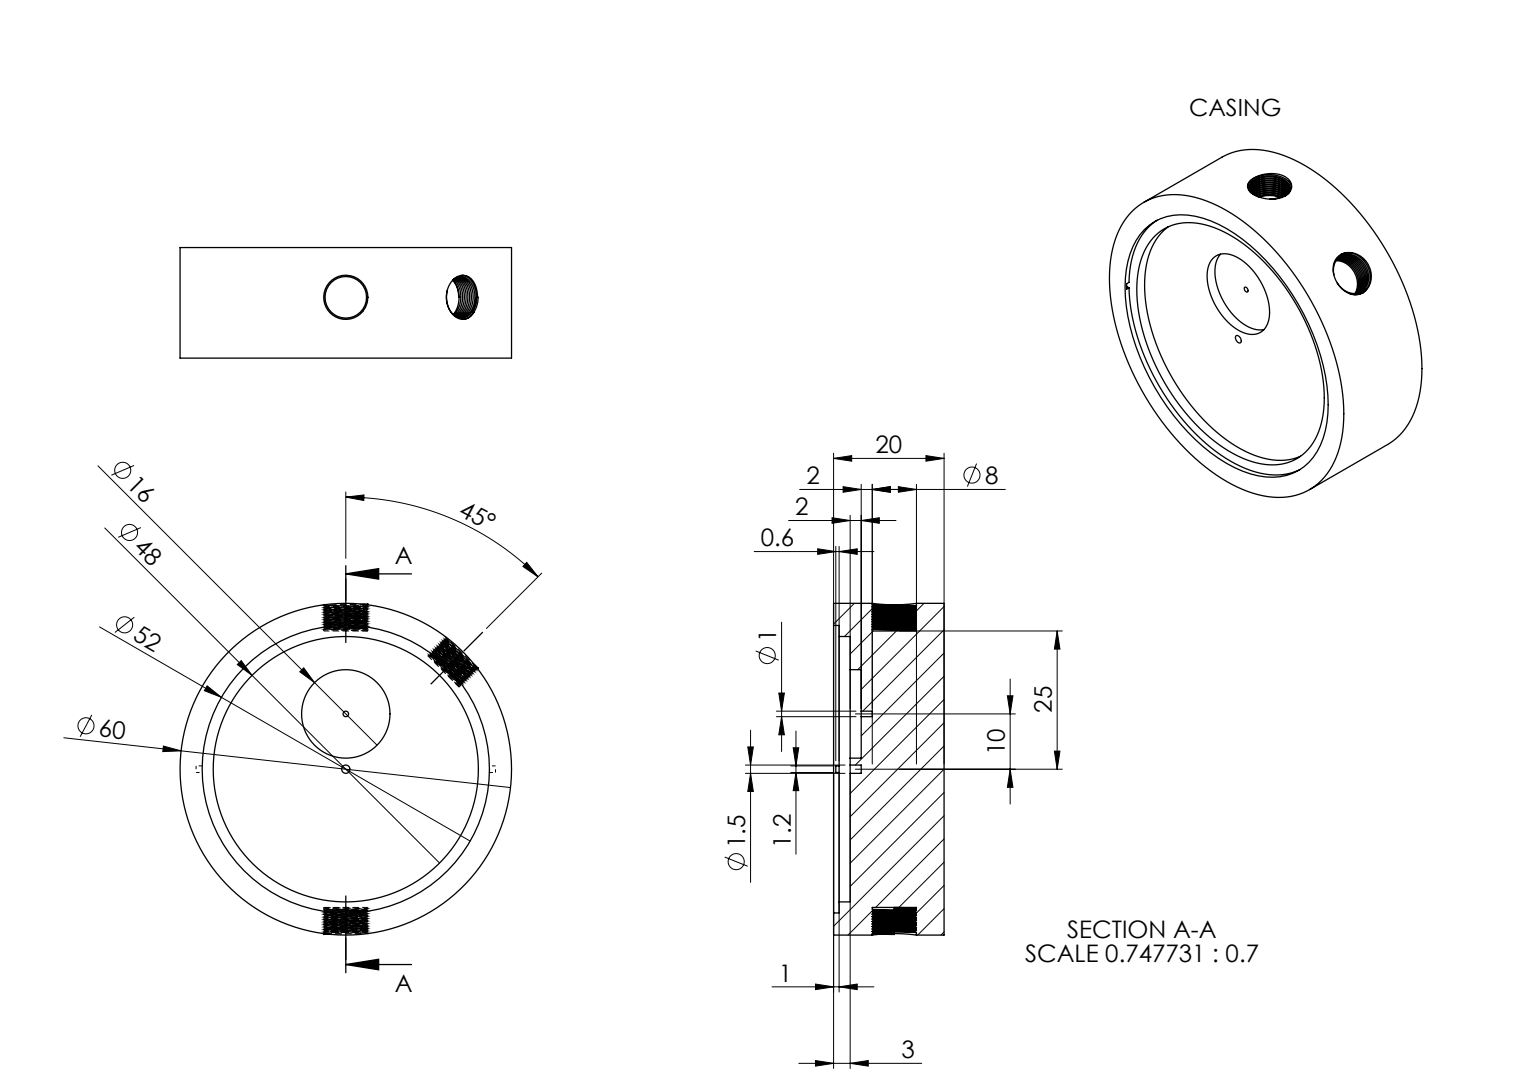
ISO-10303-21;
HEADER;
FILE_DESCRIPTION (('STEP AP214'),
    '1' );
FILE_NAME ('casing.step',
    '2026-10-26T12:50:16',
    ( '' ),
    ( '' ),
    'SwSTEP 2.0',
    'SolidWorks 2026',
    '' );
FILE_SCHEMA (( 'AUTOMOTIVE_DESIGN' ));
ENDSEC;

DATA;
#5=CARTESIAN_POINT ( 'NONE',  ( -3.756430356249995661, 28.14062499938548356, 6.831223922626973533 ) ) ;
#7=CARTESIAN_POINT ( 'NONE',  ( -3.137519842735244810E-15, 26.85624999877096641, 4.999999999999991118 ) ) ;
#13=CARTESIAN_POINT ( 'NONE',  ( 3.999999999999996003, -29.63124999877096499, 6.690598923241487306 ) ) ;
#14=CARTESIAN_POINT ( 'NONE',  ( -1.878215178124995832, 27.65312499938548640, 5.746835883940462963 ) ) ;
#15=CARTESIAN_POINT ( 'NONE',  ( 1.999999999999995781, -26.05000000000000071, 5.535898384862237620 ) ) ;
#21=CARTESIAN_POINT ( 'NONE',  ( -4.000000000000001776, -29.01249999999999929, 11.30940107675849760 ) ) ;
#22=CARTESIAN_POINT ( 'NONE',  ( 1.878215178124995832, -29.34062499938548285, 5.746835883940462963 ) ) ;
#23=ORIENTED_EDGE ( 'NONE', *, *, #8423, .T. ) ;
#24=AXIS2_PLACEMENT_3D ( 'NONE', #8722, #14489, #16466 ) ;
#28=CARTESIAN_POINT ( 'NONE',  ( -1.878215178125000939, -26.86562499938548498, 12.25316411605952283 ) ) ;
#33=CARTESIAN_POINT ( 'NONE',  ( 2.610164000359269210, 29.83019057377770622, 12.11182326528050623 ) ) ;
#34=CARTESIAN_POINT ( 'NONE',  ( 3.756430356250003211, 25.74062499938548498, 6.831223922626973533 ) ) ;
#37=CARTESIAN_POINT ( 'NONE',  ( -1.859271017917182139E-15, -26.18124999877096570, 12.99999999999999289 ) ) ;
#38=CARTESIAN_POINT ( 'NONE',  ( 20.96136040992792715, 18.30516303196848327, 12.25316411605952283 ) ) ;
#41=AXIS2_PLACEMENT_3D ( 'NONE', #20683, #20557, #10217 ) ;
#44=EDGE_CURVE ( 'NONE', #18967, #21735, #3508, .T. ) ;
#45=CARTESIAN_POINT ( 'NONE',  ( 2.620986760973688460E-15, 28.48750000000000071, 13.61880215351699874 ) ) ;
#48=DIRECTION ( 'NONE',  ( -0.7071067811865463515, 0.7071067811865487940, 0.000000000000000000 ) ) ;
#50=CARTESIAN_POINT ( 'NONE',  ( -1.071796769724487675, -29.53615380933863221, 4.999999999999988454 ) ) ;
#52=ORIENTED_EDGE ( 'NONE', *, *, #23161, .T. ) ;
#58=CARTESIAN_POINT ( 'NONE',  ( -3.756430356249996994, 25.47812499938548569, 8.999999999999992895 ) ) ;
#59=DIRECTION ( 'NONE',  ( 0.000000000000000000, 1.000000000000000000, 0.000000000000000000 ) ) ;
#64=ORIENTED_EDGE ( 'NONE', *, *, #14205, .F. ) ;
#65=ADVANCED_FACE ( 'NONE', ( #4510 ), #16441, .F. ) ;
#67=( BOUNDED_CURVE ( )  B_SPLINE_CURVE ( 2, ( #11399, #18754, #8825, #845, #17301 ),
 .UNSPECIFIED., .F., .F. ) 
 B_SPLINE_CURVE_WITH_KNOTS ( ( 3, 2, 3 ),
 ( 0.000000000000000000, 0.01666666666666666644, 0.02500000000000000486 ),
 .UNSPECIFIED. ) 
 CURVE ( )  GEOMETRIC_REPRESENTATION_ITEM ( )  RATIONAL_B_SPLINE_CURVE ( ( 1.000000000000000000, 0.8660254037844387076, 1.000000000000000000, 0.9330127018922194093, 0.9330127018922194093 ) ) 
 REPRESENTATION_ITEM ( '' )  );
#71=CARTESIAN_POINT ( 'NONE',  ( -2.000000000000003997, -26.87500000000000355, 5.535898384862238508 ) ) ;
#76=CARTESIAN_POINT ( 'NONE',  ( -3.756430356249996994, 26.26562499938548711, 8.999999999999992895 ) ) ;
#78=VECTOR ( 'NONE', #8219, 1000.000000000000000 ) ;
#80=CARTESIAN_POINT ( 'NONE',  ( -3.469446951953614189E-15, -30.00000000000000355, 4.999999999999992006 ) ) ;
#82=CARTESIAN_POINT ( 'NONE',  ( 15.67125403804690009, 21.32810828753921228, 11.30940107675849404 ) ) ;
#84=DIRECTION ( 'NONE',  ( 0.000000000000000000, 1.000000000000000000, 0.000000000000000000 ) ) ;
#85=CARTESIAN_POINT ( 'NONE',  ( 0.000000000000000000, 10.00000000000000000, 13.00000000000000178 ) ) ;
#88=CARTESIAN_POINT ( 'NONE',  ( 17.82559248041273037, 23.13798723633140142, 8.999999999999992895 ) ) ;
#91=CARTESIAN_POINT ( 'NONE',  ( -3.752267015613588906E-15, -27.36250000000000071, 4.381197846482986158 ) ) ;
#96=DIRECTION ( 'NONE',  ( 0.000000000000000000, 1.000000000000000000, 0.000000000000000000 ) ) ;
#104=AXIS2_PLACEMENT_3D ( 'NONE', #18680, #4701, #2727 ) ;
#108=FACE_OUTER_BOUND ( 'NONE', #8911, .T. ) ;
#111=FACE_OUTER_BOUND ( 'NONE', #10588, .T. ) ;
#116=CARTESIAN_POINT ( 'NONE',  ( 23.35662086519912606, 17.69976661570667176, 6.690598923241489970 ) ) ;
#119=CARTESIAN_POINT ( 'NONE',  ( 3.472074595960224386, 29.79875828571876184, 6.996763648122163559 ) ) ;
#122=CARTESIAN_POINT ( 'NONE',  ( -3.178742173564956808, 29.83148068024111410, 6.557713274934318548 ) ) ;
#125=VERTEX_POINT ( 'NONE', #4004 ) ;
#130=VERTEX_POINT ( 'NONE', #22041 ) ;
#133=ORIENTED_EDGE ( 'NONE', *, *, #9364, .F. ) ;
#143=CARTESIAN_POINT ( 'NONE',  ( -3.756430356249995661, 26.22812499938548214, 6.831223922626973533 ) ) ;
#149=DIRECTION ( 'NONE',  ( -0.7071067811865487940, -0.7071067811865463515, 0.000000000000000000 ) ) ;
#150=CARTESIAN_POINT ( 'NONE',  ( -3.369928719974892281E-15, -25.50624999877096855, 4.999999999999992006 ) ) ;
#152=CARTESIAN_POINT ( 'NONE',  ( -4.000000000000003553, -28.99374999877096926, 8.999999999999992895 ) ) ;
#153=CARTESIAN_POINT ( 'NONE',  ( -3.756430356249996994, 28.62812499938548427, 8.999999999999992895 ) ) ;
#156=CARTESIAN_POINT ( 'NONE',  ( -3.834746474454188013E-15, -25.95624999877096428, 4.999999999999992006 ) ) ;
#159=CARTESIAN_POINT ( 'NONE',  ( -2.672651547586948120E-15, -29.52812499938548285, 13.33755215474603162 ) ) ;
#160=ORIENTED_EDGE ( 'NONE', *, *, #14930, .T. ) ;
#167=CARTESIAN_POINT ( 'NONE',  ( 1.859271017917182139E-15, 29.78124999877096712, 12.99999999999999289 ) ) ;
#168=CARTESIAN_POINT ( 'NONE',  ( 3.756430356250003211, 26.19062499938548783, 6.831223922626973533 ) ) ;
#172=FACE_OUTER_BOUND ( 'NONE', #2936, .T. ) ;
#173=CARTESIAN_POINT ( 'NONE',  ( 18.33395301051795911, 18.33395301051789161, 13.33755215474602984 ) ) ;
#174=CARTESIAN_POINT ( 'NONE',  ( 17.58044234725058175, 23.23729659674288683, 11.30940107675849404 ) ) ;
#177=CARTESIAN_POINT ( 'NONE',  ( 4.000000000000003553, 28.18750000000000000, 6.690598923241489970 ) ) ;
#178=CARTESIAN_POINT ( 'NONE',  ( 3.756430356250003211, 28.77812499938548285, 6.831223922626973533 ) ) ;
#180=DIRECTION ( 'NONE',  ( 1.000000000000000000, 0.000000000000000000, 0.000000000000000000 ) ) ;
#188=CARTESIAN_POINT ( 'NONE',  ( 4.000000000000003553, 29.44374999877096855, 8.999999999999992895 ) ) ;
#201=CARTESIAN_POINT ( 'NONE',  ( 15.35955758102464408, 20.67195233694332401, 8.999999999999992895 ) ) ;
#202=EDGE_CURVE ( 'NONE', #18727, #446, #20080, .T. ) ;
#203=CARTESIAN_POINT ( 'NONE',  ( -1.878215178124998497, 25.44062499938548427, 12.25316411605951927 ) ) ;
#205=CARTESIAN_POINT ( 'NONE',  ( 3.999999999999996447, -28.76874999877096784, 8.999999999999992895 ) ) ;
#206=CARTESIAN_POINT ( 'NONE',  ( 20.78010053211970032, 20.78010053211962926, 13.61880215351699874 ) ) ;
#210=CARTESIAN_POINT ( 'NONE',  ( 21.65072575558658130, 18.82229863084031507, 5.535898384862238508 ) ) ;
#212=FACE_BOUND ( 'NONE', #16233, .T. ) ;
#213=ORIENTED_EDGE ( 'NONE', *, *, #20465, .F. ) ;
#215=CARTESIAN_POINT ( 'NONE',  ( -4.000000000000003553, -28.18750000000000000, 6.690598923241489970 ) ) ;
#217=ORIENTED_EDGE ( 'NONE', *, *, #6066, .T. ) ;
#219=CARTESIAN_POINT ( 'NONE',  ( 23.82728881686095335, 18.17043456736849549, 8.999999999999992895 ) ) ;
#223=( NAMED_UNIT ( * ) PLANE_ANGLE_UNIT ( ) SI_UNIT ( $, .RADIAN. ) );
#225=( BOUNDED_SURFACE ( )  B_SPLINE_SURFACE ( 1, 2, ( 
 ( #23282, #15066, #19226, #12835, #25256, #13355, #9305, #1328, #23041, #11121, #11003, #7335, #805, #4859, #6951, #3034, #14929, #17290, #15314, #5365, #6826, #4989, #3408, #23165, #3271, #1184, #20809, #11245, #18713, #14809, #25127, #22903, #22782, #7213, #5128, #3154, #5245, #18859, #15195, #2891, #949, #8926, #12968, #18983, #9042, #17024, #13105, #21078, #19100, #11896, #19864, #23669, #17408, #3538, #9928, #7455, #23415, #17792, #7595, #5502, #13493, #15443, #3926, #23933, #5746, #11511, #11387, #7721, #9545, #15581, #17532, #25759, #1963, #17913, #11771, #13997, #19750, #5, #5885, #21462, #15967, #25506, #15705, #23549, #1848, #23795, #25372, #17671, #13730, #5631, #19480, #7979, #6016, #21968, #13611, #19361, #1456, #1574, #21577, #3656, #11632, #19609, #21708, #3793, #1713, #9427, #9810, #9687, #25639, #7840, #15824, #13869, #21843, #20128, #2470, #14641, #12011, #18436, #18572, #4433, #18301 ),
 ( #24054, #14507, #12542, #2614, #10441, #2229, #2094, #531, #16352, #14392, #16485, #4175, #8503, #22479, #10573, #24447, #10187, #4559, #4044, #6524, #20373, #20519, #19988, #654, #8623, #24321, #10061, #22086, #16600, #143, #16090, #24562, #267, #6138, #14122, #8116, #6652, #18060, #6401, #12154, #18184, #393, #8235, #16212, #24181, #6269, #14261, #22228, #12407, #4313, #12287, #20253, #2351, #10306, #8362, #22349, #1037, #20778, #13070, #9481, #10697, #2998, #18952, #8890, #4827, #13549, #5568, #15512, #911, #19534, #11566, #772, #10827, #8745, #16735, #4951, #7655, #10966, #14776, #22871, #18820, #12933, #17460, #9011, #22621, #22752, #12804, #21513, #16992, #2857, #24957, #14897, #16874, #24838, #7039, #24705, #25571, #25432, #6915, #12683, #18684, #9614, #1636, #15027, #23481, #21048, #20911, #20652, #3123, #23005, #5092, #7517, #11091, #19070, #3595, #17594, #1512, #4708, #2735, #6791, #18129 ) ),
 .UNSPECIFIED., .F., .F., .F. ) 
 B_SPLINE_SURFACE_WITH_KNOTS ( ( 2, 2 ),
 ( 3, 2, 2, 2, 2, 2, 2, 2, 2, 2, 2, 2, 2, 2, 2, 2, 2, 2, 2, 2, 2, 2, 2, 2, 2, 2, 2, 2, 2, 2, 2, 2, 2, 2, 2, 2, 2, 2, 2, 2, 2, 2, 2, 2, 2, 2, 2, 2, 2, 2, 2, 2, 2, 2, 2, 2, 2, 2, 2, 2, 3 ),
 ( 0.000000000000000000, 1.000000000000000000 ),
 ( 0.000000000000000000, 0.01666666666666666644, 0.03333333333333333287, 0.05000000000000000278, 0.06666666666666666574, 0.08333333333333332871, 0.1000000000000000056, 0.1166666666666666685, 0.1333333333333333315, 0.1499999999999999944, 0.1666666666666666574, 0.1833333333333333204, 0.2000000000000000111, 0.2166666666666666741, 0.2333333333333333370, 0.2500000000000000000, 0.2666666666666666630, 0.2833333333333333259, 0.2999999999999999889, 0.3166666666666666519, 0.3333333333333333148, 0.3499999999999999778, 0.3666666666666666408, 0.3833333333333333592, 0.4000000000000000222, 0.4166666666666666852, 0.4333333333333333481, 0.4500000000000000111, 0.4666666666666666741, 0.4833333333333333370, 0.5000000000000000000, 0.5166666666666667185, 0.5333333333333333259, 0.5500000000000000444, 0.5666666666666666519, 0.5833333333333333703, 0.5999999999999999778, 0.6166666666666666963, 0.6333333333333333037, 0.6500000000000000222, 0.6666666666666666297, 0.6833333333333333481, 0.6999999999999999556, 0.7166666666666666741, 0.7333333333333332815, 0.7500000000000000000, 0.7666666666666667185, 0.7833333333333333259, 0.8000000000000000444, 0.8166666666666666519, 0.8333333333333333703, 0.8499999999999999778, 0.8666666666666666963, 0.8833333333333333037, 0.9000000000000000222, 0.9166666666666666297, 0.9333333333333333481, 0.9499999999999999556, 0.9666666666666666741, 0.9833333333333332815, 1.000000000000000000 ),
 .UNSPECIFIED. ) 
 GEOMETRIC_REPRESENTATION_ITEM ( )  RATIONAL_B_SPLINE_SURFACE ( (
 ( 1.000000000000000000, 0.8660254037844387076, 1.000000000000000000, 0.8660254037844387076, 1.000000000000000000, 0.8660254037844387076, 1.000000000000000000, 0.8660254037844387076, 1.000000000000000000, 0.8660254037844387076, 1.000000000000000000, 0.8660254037844387076, 1.000000000000000000, 0.8660254037844387076, 1.000000000000000000, 0.8660254037844387076, 1.000000000000000000, 0.8660254037844387076, 1.000000000000000000, 0.8660254037844387076, 1.000000000000000000, 0.8660254037844387076, 1.000000000000000000, 0.8660254037844387076, 1.000000000000000000, 0.8660254037844387076, 1.000000000000000000, 0.8660254037844387076, 1.000000000000000000, 0.8660254037844387076, 1.000000000000000000, 0.8660254037844387076, 1.000000000000000000, 0.8660254037844387076, 1.000000000000000000, 0.8660254037844387076, 1.000000000000000000, 0.8660254037844387076, 1.000000000000000000, 0.8660254037844387076, 1.000000000000000000, 0.8660254037844387076, 1.000000000000000000, 0.8660254037844387076, 1.000000000000000000, 0.8660254037844387076, 1.000000000000000000, 0.8660254037844387076, 1.000000000000000000, 0.8660254037844387076, 1.000000000000000000, 0.8660254037844387076, 1.000000000000000000, 0.8660254037844387076, 1.000000000000000000, 0.8660254037844387076, 1.000000000000000000, 0.8660254037844387076, 1.000000000000000000, 0.8660254037844387076, 1.000000000000000000, 0.8660254037844387076, 1.000000000000000000, 0.8660254037844387076, 1.000000000000000000, 0.8660254037844387076, 1.000000000000000000, 0.8660254037844387076, 1.000000000000000000, 0.8660254037844387076, 1.000000000000000000, 0.8660254037844387076, 1.000000000000000000, 0.8660254037844387076, 1.000000000000000000, 0.8660254037844387076, 1.000000000000000000, 0.8660254037844387076, 1.000000000000000000, 0.8660254037844387076, 1.000000000000000000, 0.8660254037844387076, 1.000000000000000000, 0.8660254037844387076, 1.000000000000000000, 0.8660254037844387076, 1.000000000000000000, 0.8660254037844387076, 1.000000000000000000, 0.8660254037844387076, 1.000000000000000000, 0.8660254037844387076, 1.000000000000000000, 0.8660254037844387076, 1.000000000000000000, 0.8660254037844387076, 1.000000000000000000, 0.8660254037844387076, 1.000000000000000000, 0.8660254037844387076, 1.000000000000000000, 0.8660254037844387076, 1.000000000000000000, 0.8660254037844387076, 1.000000000000000000, 0.8660254037844387076, 1.000000000000000000, 0.8660254037844387076, 1.000000000000000000, 0.8660254037844387076, 1.000000000000000000, 0.8660254037844387076, 1.000000000000000000, 0.8660254037844387076, 1.000000000000000000, 0.8660254037844387076, 1.000000000000000000, 0.8660254037844387076, 1.000000000000000000, 0.8660254037844387076, 1.000000000000000000),
 ( 1.000000000000000000, 0.8660254037844387076, 1.000000000000000000, 0.8660254037844387076, 1.000000000000000000, 0.8660254037844387076, 1.000000000000000000, 0.8660254037844387076, 1.000000000000000000, 0.8660254037844387076, 1.000000000000000000, 0.8660254037844387076, 1.000000000000000000, 0.8660254037844387076, 1.000000000000000000, 0.8660254037844387076, 1.000000000000000000, 0.8660254037844387076, 1.000000000000000000, 0.8660254037844387076, 1.000000000000000000, 0.8660254037844387076, 1.000000000000000000, 0.8660254037844387076, 1.000000000000000000, 0.8660254037844387076, 1.000000000000000000, 0.8660254037844387076, 1.000000000000000000, 0.8660254037844387076, 1.000000000000000000, 0.8660254037844387076, 1.000000000000000000, 0.8660254037844387076, 1.000000000000000000, 0.8660254037844387076, 1.000000000000000000, 0.8660254037844387076, 1.000000000000000000, 0.8660254037844387076, 1.000000000000000000, 0.8660254037844387076, 1.000000000000000000, 0.8660254037844387076, 1.000000000000000000, 0.8660254037844387076, 1.000000000000000000, 0.8660254037844387076, 1.000000000000000000, 0.8660254037844387076, 1.000000000000000000, 0.8660254037844387076, 1.000000000000000000, 0.8660254037844387076, 1.000000000000000000, 0.8660254037844387076, 1.000000000000000000, 0.8660254037844387076, 1.000000000000000000, 0.8660254037844387076, 1.000000000000000000, 0.8660254037844387076, 1.000000000000000000, 0.8660254037844387076, 1.000000000000000000, 0.8660254037844387076, 1.000000000000000000, 0.8660254037844387076, 1.000000000000000000, 0.8660254037844387076, 1.000000000000000000, 0.8660254037844387076, 1.000000000000000000, 0.8660254037844387076, 1.000000000000000000, 0.8660254037844387076, 1.000000000000000000, 0.8660254037844387076, 1.000000000000000000, 0.8660254037844387076, 1.000000000000000000, 0.8660254037844387076, 1.000000000000000000, 0.8660254037844387076, 1.000000000000000000, 0.8660254037844387076, 1.000000000000000000, 0.8660254037844387076, 1.000000000000000000, 0.8660254037844387076, 1.000000000000000000, 0.8660254037844387076, 1.000000000000000000, 0.8660254037844387076, 1.000000000000000000, 0.8660254037844387076, 1.000000000000000000, 0.8660254037844387076, 1.000000000000000000, 0.8660254037844387076, 1.000000000000000000, 0.8660254037844387076, 1.000000000000000000, 0.8660254037844387076, 1.000000000000000000, 0.8660254037844387076, 1.000000000000000000, 0.8660254037844387076, 1.000000000000000000, 0.8660254037844387076, 1.000000000000000000, 0.8660254037844387076, 1.000000000000000000, 0.8660254037844387076, 1.000000000000000000, 0.8660254037844387076, 1.000000000000000000, 0.8660254037844387076, 1.000000000000000000, 0.8660254037844387076, 1.000000000000000000) ) ) 
 REPRESENTATION_ITEM ( '' )  SURFACE ( )  );
#230=CIRCLE ( 'NONE', #3567, 26.00000000000000355 ) ;
#234=CARTESIAN_POINT ( 'NONE',  ( 22.12360341637413441, 16.46674916688168366, 6.690598923241489970 ) ) ;
#235=CARTESIAN_POINT ( 'NONE',  ( 21.07620149587250680, 15.41934724638005605, 11.30940107675849760 ) ) ;
#237=CARTESIAN_POINT ( 'NONE',  ( 16.26111872703749128, 21.57351348295617299, 11.16877607737301226 ) ) ;
#238=CARTESIAN_POINT ( 'NONE',  ( 20.69613160098474580, 17.86770447623847957, 5.535898384862238508 ) ) ;
#245=CARTESIAN_POINT ( 'NONE',  ( -1.290629128713961293, 29.97320584640673147, 5.204870533884474071 ) ) ;
#249=AXIS2_PLACEMENT_3D ( 'NONE', #7329, #17401, #17148 ) ;
#253=CARTESIAN_POINT ( 'NONE',  ( 1.878215178124998497, -26.79062499938548214, 12.25316411605951927 ) ) ;
#256=VERTEX_POINT ( 'NONE', #11047 ) ;
#267=CARTESIAN_POINT ( 'NONE',  ( -1.878215178124998497, 26.34062499938548285, 12.25316411605951927 ) ) ;
#274=CARTESIAN_POINT ( 'NONE',  ( 15.32653948221845575, 20.98339373171076971, 8.999999999999992895 ) ) ;
#275=CARTESIAN_POINT ( 'NONE',  ( 3.999999999999996003, -29.18124999877096926, 6.690598923241487306 ) ) ;
#278=DIRECTION ( 'NONE',  ( 0.000000000000000000, 1.000000000000000000, 0.000000000000000000 ) ) ;
#280=CARTESIAN_POINT ( 'NONE',  ( 3.178742173564956808, -29.83148068024111410, 6.557713274934318548 ) ) ;
#282=CARTESIAN_POINT ( 'NONE',  ( 1.057460391440397258E-14, -29.16249999999999787, 4.999999999999992006 ) ) ;
#283=FACE_OUTER_BOUND ( 'NONE', #1653, .T. ) ;
#285=EDGE_LOOP ( 'NONE', ( #3996, #19961, #21885, #25596, #64, #22498, #18380, #2629, #2882, #13648, #16581, #11690, #2311, #3515, #5348, #18845, #16021, #25747, #20827, #6154, #13089, #936, #2532, #21309 ) ) ;
#290=EDGE_LOOP ( 'NONE', ( #13571, #12401, #24240, #13980, #21957, #2916, #23588, #1468, #14108, #13538, #2496, #5234, #22275, #20569, #6506, #25331, #10531, #8615, #1170, #12139, #14587, #14625, #15332, #12330, #21832 ) ) ;
#292=CARTESIAN_POINT ( 'NONE',  ( 3.756430356250002323, 27.01562499938548356, 11.16877607737301403 ) ) ;
#295=CARTESIAN_POINT ( 'NONE',  ( 20.11283227250407180, 17.45663489454462436, 5.746835883940462963 ) ) ;
#301=CARTESIAN_POINT ( 'NONE',  ( 3.756430356250003655, 29.64062499938548356, 8.999999999999992895 ) ) ;
#304=CARTESIAN_POINT ( 'NONE',  ( 21.21320343559646915, 21.21320343559638744, 8.999999999999992895 ) ) ;
#312=CARTESIAN_POINT ( 'NONE',  ( 21.42091605170094937, 15.76406180220850040, 8.999999999999992895 ) ) ;
#315=DIRECTION ( 'NONE',  ( 0.000000000000000000, 1.000000000000000000, 0.000000000000000000 ) ) ;
#319=CARTESIAN_POINT ( 'NONE',  ( 4.000000000000003553, 29.08750000000000213, 6.690598923241489970 ) ) ;
#323=CARTESIAN_POINT ( 'NONE',  ( -3.756430356249995661, 26.67812499938548498, 6.831223922626973533 ) ) ;
#325=CARTESIAN_POINT ( 'NONE',  ( 18.91510639674018890, 21.74353352148630236, 5.535898384862237620 ) ) ;
#328=CARTESIAN_POINT ( 'NONE',  ( 4.000000000000003553, 25.03750000000000142, 6.690598923241489970 ) ) ;
#329=CARTESIAN_POINT ( 'NONE',  ( 1.878215178124998497, -25.89062499938548356, 12.25316411605951927 ) ) ;
#331=AXIS2_PLACEMENT_3D ( 'NONE', #1726, #17803, #5513 ) ;
#338=ORIENTED_EDGE ( 'NONE', *, *, #8418, .T. ) ;
#339=CARTESIAN_POINT ( 'NONE',  ( 1.071796769724493448, -29.12634618820329990, 4.999999999999995559 ) ) ;
#347=CARTESIAN_POINT ( 'NONE',  ( 3.756430356249996994, -26.82812499938548711, 8.999999999999992895 ) ) ;
#356=CARTESIAN_POINT ( 'NONE',  ( 19.96824085905927149, 21.48399038691124474, 12.99999999999999289 ) ) ;
#358=CIRCLE ( 'NONE', #25835, 0.5000000000000001110 ) ;
#360=CARTESIAN_POINT ( 'NONE',  ( -3.469446951953614189E-15, -30.00000000000000355, 8.999999999999992895 ) ) ;
#361=CARTESIAN_POINT ( 'NONE',  ( 21.67957950013421353, 16.36718474421539682, 11.16877607737301226 ) ) ;
#363=CARTESIAN_POINT ( 'NONE',  ( 16.55955693104344206, 22.21641118053575426, 8.999999999999992895 ) ) ;
#365=CARTESIAN_POINT ( 'NONE',  ( 3.999999999999996447, -27.02500000000000213, 8.999999999999992895 ) ) ;
#368=CARTESIAN_POINT ( 'NONE',  ( -2.007411586324088226, 29.93355017142139118, 12.46960170373642640 ) ) ;
#370=CARTESIAN_POINT ( 'NONE',  ( 17.85665593321704137, 17.85665593321697386, 4.662447845253954171 ) ) ;
#371=CARTESIAN_POINT ( 'NONE',  ( -1.626862140677534194E-14, -28.03750000000000497, 12.99999999999999289 ) ) ;
#374=CARTESIAN_POINT ( 'NONE',  ( 2.620986760973688460E-15, 26.63124999877097565, 13.61880215351699874 ) ) ;
#375=CARTESIAN_POINT ( 'NONE',  ( 3.756430356249996994, -26.71562499938548285, 8.999999999999992895 ) ) ;
#377=ORIENTED_EDGE ( 'NONE', *, *, #20034, .T. ) ;
#393=CARTESIAN_POINT ( 'NONE',  ( -3.756430356249995661, 26.67812499938548498, 6.831223922626973533 ) ) ;
#400=CARTESIAN_POINT ( 'NONE',  ( -1.999999999999995781, 28.69374999877096855, 5.535898384862237620 ) ) ;
#401=CARTESIAN_POINT ( 'NONE',  ( -3.756430356250003655, -25.70312499938548356, 8.999999999999992895 ) ) ;
#410=CARTESIAN_POINT ( 'NONE',  ( 21.21320343559646915, 21.21320343559638744, 8.999999999999992895 ) ) ;
#421=VERTEX_POINT ( 'NONE', #17718 ) ;
#424=CARTESIAN_POINT ( 'NONE',  ( -1.878215178124995832, 25.85312499938548569, 5.746835883940462963 ) ) ;
#426=ADVANCED_FACE ( 'NONE', ( #15751 ), #3586, .T. ) ;
#430=CARTESIAN_POINT ( 'NONE',  ( 20.64316235839397962, 17.98696498043453573, 12.25316411605952283 ) ) ;
#437=CARTESIAN_POINT ( 'NONE',  ( -1.878215178124995832, 28.89062499938548356, 5.746835883940462963 ) ) ;
#440=CARTESIAN_POINT ( 'NONE',  ( 18.19474136253732865, 18.19474136253726826, 12.99999999999999289 ) ) ;
#446=VERTEX_POINT ( 'NONE', #13409 ) ;
#449=CARTESIAN_POINT ( 'NONE',  ( -3.999999999999996447, 26.12500000000000355, 8.999999999999992895 ) ) ;
#461=AXIS2_PLACEMENT_3D ( 'NONE', #21744, #5539, #19508 ) ;
#465=CARTESIAN_POINT ( 'NONE',  ( 3.735045420075836212E-15, 27.05312499938548498, 4.662447845253954171 ) ) ;
#467=CARTESIAN_POINT ( 'NONE',  ( 17.93620544610053003, 17.93620544610046252, 4.662447845253954171 ) ) ;
#468=CARTESIAN_POINT ( 'NONE',  ( 23.66156066545488201, 18.00470641596242771, 11.30940107675849760 ) ) ;
#471=CARTESIAN_POINT ( 'NONE',  ( 0.000000000000000000, 0.000000000000000000, 20.00001200000000168 ) ) ;
#476=VERTEX_POINT ( 'NONE', #17452 ) ;
#478=CARTESIAN_POINT ( 'NONE',  ( -4.000000000000003553, -28.15000000000000213, 8.999999999999992895 ) ) ;
#487=CARTESIAN_POINT ( 'NONE',  ( -1.878215178125004048, -27.57812499938548711, 5.746835883940462963 ) ) ;
#494=CARTESIAN_POINT ( 'NONE',  ( 21.86285778994254514, 19.03443066519628601, 12.46410161513774817 ) ) ;
#499=CARTESIAN_POINT ( 'NONE',  ( 18.02680350200553150, 20.85523062675164851, 12.46410161513774639 ) ) ;
#501=CARTESIAN_POINT ( 'NONE',  ( 15.94292067550354730, 21.25531543142222901, 11.16877607737301226 ) ) ;
#502=CARTESIAN_POINT ( 'NONE',  ( 22.18105584147648912, 19.35262871673023000, 12.46410161513774817 ) ) ;
#503=CARTESIAN_POINT ( 'NONE',  ( 3.834746474454188013E-15, 28.26249999999999929, 4.999999999999992006 ) ) ;
#504=CARTESIAN_POINT ( 'NONE',  ( 21.55218544786934132, 20.03643592001721530, 12.99999999999999467 ) ) ;
#506=CARTESIAN_POINT ( 'NONE',  ( 27.09999999999999787, 0.6000000000000000888, 19.59999999999999787 ) ) ;
#509=CARTESIAN_POINT ( 'NONE',  ( 18.33395301051795911, 18.33395301051789517, 13.33755215474603162 ) ) ;
#511=CARTESIAN_POINT ( 'NONE',  ( 3.756430356250003655, 29.69687499938548569, 8.999999999999992895 ) ) ;
#513=CARTESIAN_POINT ( 'NONE',  ( 3.756430356249996994, -27.16562499938548214, 8.999999999999992895 ) ) ;
#514=CARTESIAN_POINT ( 'NONE',  ( -3.999999999999995559, 25.18750000000000000, 6.690598923241487306 ) ) ;
#517=LINE ( 'NONE', #10811, #790 ) ;
#520=CARTESIAN_POINT ( 'NONE',  ( 3.756430356249995661, -29.49062499938548498, 6.831223922626973533 ) ) ;
#522=AXIS2_PLACEMENT_3D ( 'NONE', #18913, #11050, #20738 ) ;
#531=CARTESIAN_POINT ( 'NONE',  ( -3.756430356249997882, 25.40312499938548285, 11.16877607737301226 ) ) ;
#540=CARTESIAN_POINT ( 'NONE',  ( 1.999999999999998224, -29.29374999877096997, 12.46410161513774639 ) ) ;
#542=CARTESIAN_POINT ( 'NONE',  ( 21.21320343559646915, 21.21320343559638744, 12.99999999999999289 ) ) ;
#544=CARTESIAN_POINT ( 'NONE',  ( 1.290629128713961293, -29.97320584640673147, 5.204870533884474071 ) ) ;
#548=LINE ( 'NONE', #4449, #1635 ) ;
#551=ORIENTED_EDGE ( 'NONE', *, *, #25079, .T. ) ;
#555=CARTESIAN_POINT ( 'NONE',  ( -4.000000000000003553, -27.73750000000000071, 6.690598923241489970 ) ) ;
#557=EDGE_LOOP ( 'NONE', ( #23842, #6060, #17814, #23687, #3257, #25679 ) ) ;
#559=CARTESIAN_POINT ( 'NONE',  ( 3.756430356250002323, 26.56562499938548783, 11.16877607737301403 ) ) ;
#563=CARTESIAN_POINT ( 'NONE',  ( 21.73261250872320716, 16.42021775280438689, 6.831223922626973533 ) ) ;
#570=CARTESIAN_POINT ( 'NONE',  ( -1.071796769724487230, 27.77634618820330559, 4.999999999999992006 ) ) ;
#572=CARTESIAN_POINT ( 'NONE',  ( -1.878215178124998497, 29.04062499938548569, 12.25316411605951927 ) ) ;
#584=CARTESIAN_POINT ( 'NONE',  ( 1.057460391440397258E-14, -28.71250000000000213, 4.999999999999992006 ) ) ;
#589=ORIENTED_EDGE ( 'NONE', *, *, #21385, .T. ) ;
#590=FACE_OUTER_BOUND ( 'NONE', #13824, .T. ) ;
#592=CARTESIAN_POINT ( 'NONE',  ( 1.071796769724487675, 29.14240381056766438, 4.999999999999988454 ) ) ;
#594=CARTESIAN_POINT ( 'NONE',  ( 20.53936981547090568, 15.22697505955208896, 6.831223922626973533 ) ) ;
#596=CARTESIAN_POINT ( 'NONE',  ( -1.878215178124995832, 28.44062499938548427, 5.746835883940462963 ) ) ;
#598=ADVANCED_FACE ( 'NONE', ( #6456 ), #4362, .F. ) ;
#599=APPLICATION_CONTEXT ( 'automotive_design' ) ;
#602=CARTESIAN_POINT ( 'NONE',  ( 1.859271017917182139E-15, 29.33124999877096428, 12.99999999999999289 ) ) ;
#603=CARTESIAN_POINT ( 'NONE',  ( -2.672651547586948120E-15, -27.72812499938548569, 13.33755215474603162 ) ) ;
#608=CARTESIAN_POINT ( 'NONE',  ( -3.752267015613588906E-15, -29.16250000000000142, 4.381197846482986158 ) ) ;
#611=ORIENTED_EDGE ( 'NONE', *, *, #24958, .T. ) ;
#617=CARTESIAN_POINT ( 'NONE',  ( -2.672651547586948120E-15, -26.04062499938548925, 13.33755215474603162 ) ) ;
#619=CARTESIAN_POINT ( 'NONE',  ( 20.05209915500855544, 18.53634962715644363, 4.999999999999989342 ) ) ;
#622=CARTESIAN_POINT ( 'NONE',  ( 3.469446951953614189E-15, 30.00000000000000355, 4.999999999999992006 ) ) ;
#623=CARTESIAN_POINT ( 'NONE',  ( 18.60454468811453310, 20.12029421596650991, 4.999999999999992006 ) ) ;
#626=CARTESIAN_POINT ( 'NONE',  ( 16.89751483010538990, 22.20990958602406451, 11.16877607737301226 ) ) ;
#627=CARTESIAN_POINT ( 'NONE',  ( 18.87533163942939041, 21.70375876417550032, 5.535898384862237620 ) ) ;
#628=CARTESIAN_POINT ( 'NONE',  ( 23.96650046397252609, 18.30964621448006824, 8.999999999999992895 ) ) ;
#629=CARTESIAN_POINT ( 'NONE',  ( 23.66156066545488201, 18.00470641596242771, 11.30940107675849760 ) ) ;
#637=CARTESIAN_POINT ( 'NONE',  ( 2.000000000000000888, 27.56874999877096855, 12.46410161513774817 ) ) ;
#638=CARTESIAN_POINT ( 'NONE',  ( 3.756430356249995661, -25.77812499938548640, 6.831223922626973533 ) ) ;
#640=ORIENTED_EDGE ( 'NONE', *, *, #22909, .T. ) ;
#644=CARTESIAN_POINT ( 'NONE',  ( 3.756430356249995661, -25.32812499938548356, 6.831223922626973533 ) ) ;
#645=ORIENTED_EDGE ( 'NONE', *, *, #15056, .T. ) ;
#646=ORIENTED_EDGE ( 'NONE', *, *, #19907, .T. ) ;
#653=CARTESIAN_POINT ( 'NONE',  ( -3.369928719974892281E-15, -25.50624999877096855, 4.999999999999992006 ) ) ;
#654=CARTESIAN_POINT ( 'NONE',  ( 3.756430356250002323, 26.00312499938548427, 11.16877607737301226 ) ) ;
#658=DIRECTION ( 'NONE',  ( 0.000000000000000000, 0.000000000000000000, -1.000000000000000000 ) ) ;
#660=CARTESIAN_POINT ( 'NONE',  ( -3.999999999999997335, 28.80624999877096926, 11.30940107675849404 ) ) ;
#661=CARTESIAN_POINT ( 'NONE',  ( -3.735045420075836212E-15, -27.16562499938548569, 4.662447845253954171 ) ) ;
#663=CARTESIAN_POINT ( 'NONE',  ( 3.999999999999996447, -26.12500000000000355, 8.999999999999992895 ) ) ;
#664=CARTESIAN_POINT ( 'NONE',  ( 1.999999999999995781, -25.15000000000000213, 5.535898384862237620 ) ) ;
#665=CARTESIAN_POINT ( 'NONE',  ( 3.974007292349814424, -29.73566758725665338, 9.525109153848150711 ) ) ;
#670=EDGE_CURVE ( 'NONE', #18554, #13915, #7548, .T. ) ;
#673=ORIENTED_EDGE ( 'NONE', *, *, #14998, .F. ) ;
#676=ADVANCED_FACE ( 'NONE', ( #6327 ), #18231, .F. ) ;
#681=CARTESIAN_POINT ( 'NONE',  ( 1.878215178125000939, 28.77812499938548640, 12.25316411605952283 ) ) ;
#684=CARTESIAN_POINT ( 'NONE',  ( 17.53391093317328142, 22.84630568909195958, 11.16877607737301226 ) ) ;
#695=CARTESIAN_POINT ( 'NONE',  ( -1.626862140677534194E-14, -28.03750000000000497, 12.99999999999999289 ) ) ;
#696=AXIS2_PLACEMENT_3D ( 'NONE', #9375, #6205, #16157 ) ;
#697=ORIENTED_EDGE ( 'NONE', *, *, #18302, .T. ) ;
#709=CARTESIAN_POINT ( 'NONE',  ( 16.28113363682029657, 21.93798788631260877, 8.999999999999992895 ) ) ;
#710=CARTESIAN_POINT ( 'NONE',  ( 4.000000000000001776, 26.76250000000000284, 11.30940107675849760 ) ) ;
#712=CARTESIAN_POINT ( 'NONE',  ( 19.23778763078571430, 16.58159025282627397, 5.746835883940462963 ) ) ;
#713=ADVANCED_FACE ( 'NONE', ( #25117 ), #1318, .F. ) ;
#715=CARTESIAN_POINT ( 'NONE',  ( 3.735045420075836212E-15, 28.40312499938548640, 4.662447845253954171 ) ) ;
#716=CARTESIAN_POINT ( 'NONE',  ( 19.55598568231966539, 16.89978830436022150, 5.746835883940462963 ) ) ;
#717=CARTESIAN_POINT ( 'NONE',  ( 20.14370442905180880, 20.14370442905173775, 13.61880215351699874 ) ) ;
#720=CARTESIAN_POINT ( 'NONE',  ( -3.735045420075836212E-15, -27.05312499938548498, 4.662447845253954171 ) ) ;
#724=CARTESIAN_POINT ( 'NONE',  ( 1.999999999999995781, -28.75000000000000000, 5.535898384862237620 ) ) ;
#731=CARTESIAN_POINT ( 'NONE',  ( 1.878215178124995832, -26.75312499938548783, 5.746835883940462963 ) ) ;
#739=( BOUNDED_CURVE ( )  B_SPLINE_CURVE ( 2, ( #20311, #10242, #24247, #15891, #16419, #18125, #8045, #19919, #14185 ),
 .UNSPECIFIED., .F., .F. ) 
 B_SPLINE_CURVE_WITH_KNOTS ( ( 3, 2, 2, 2, 3 ),
 ( 0.8750000000000000000, 0.8833333333333333037, 0.9000000000000000222, 0.9166666666666666297, 0.9250000000000000444 ),
 .UNSPECIFIED. ) 
 CURVE ( )  GEOMETRIC_REPRESENTATION_ITEM ( )  RATIONAL_B_SPLINE_CURVE ( ( 0.9330127018922194093, 0.9330127018922194093, 1.000000000000000000, 0.8660254037844387076, 1.000000000000000000, 0.8660254037844387076, 1.000000000000000000, 0.9330127018922189652, 0.9330127018922194093 ) ) 
 REPRESENTATION_ITEM ( '' )  );
#744=CARTESIAN_POINT ( 'NONE',  ( 1.999999999999995781, -28.24374999877096570, 5.535898384862237620 ) ) ;
#745=CARTESIAN_POINT ( 'NONE',  ( 16.23460222274299980, 21.54699697866167440, 8.999999999999992895 ) ) ;
#746=CARTESIAN_POINT ( 'NONE',  ( 20.19238178538755690, 17.53618440742811302, 5.746835883940462963 ) ) ;
#748=( BOUNDED_CURVE ( )  B_SPLINE_CURVE ( 2, ( #10541, #623, #16571, #872, #4915, #24529, #14867, #6614, #12897 ),
 .UNSPECIFIED., .F., .F. ) 
 B_SPLINE_CURVE_WITH_KNOTS ( ( 3, 2, 2, 2, 3 ),
 ( 0.5250000000000000222, 0.5333333333333333259, 0.5500000000000000444, 0.5666666666666666519, 0.5750000000000000666 ),
 .UNSPECIFIED. ) 
 CURVE ( )  GEOMETRIC_REPRESENTATION_ITEM ( )  RATIONAL_B_SPLINE_CURVE ( ( 0.9330127018922194093, 0.9330127018922194093, 1.000000000000000000, 0.8660254037844387076, 1.000000000000000000, 0.8660254037844387076, 1.000000000000000000, 0.9330127018922189652, 0.9330127018922194093 ) ) 
 REPRESENTATION_ITEM ( '' )  );
#752=CARTESIAN_POINT ( 'NONE',  ( 19.68856820379214057, 17.03237082583270023, 12.25316411605952283 ) ) ;
#753=ORIENTED_EDGE ( 'NONE', *, *, #6718, .T. ) ;
#755=CARTESIAN_POINT ( 'NONE',  ( 4.000000000000001776, 27.60624999877096641, 11.30940107675849760 ) ) ;
#756=CARTESIAN_POINT ( 'NONE',  ( -2.672651547586948120E-15, -27.72812499938548569, 13.33755215474602984 ) ) ;
#761=CARTESIAN_POINT ( 'NONE',  ( -3.756430356250004099, -29.34062499938548640, 6.831223922626973533 ) ) ;
#763=ORIENTED_EDGE ( 'NONE', *, *, #18899, .F. ) ;
#767=CARTESIAN_POINT ( 'NONE',  ( 1.071796769724494558, 27.79240381056766651, 4.999999999999992895 ) ) ;
#769=EDGE_CURVE ( 'NONE', #20241, #8698, #8602, .T. ) ;
#772=CARTESIAN_POINT ( 'NONE',  ( 3.756430356250002323, 27.80312499938548143, 11.16877607737301226 ) ) ;
#777=CARTESIAN_POINT ( 'NONE',  ( 23.01498157845693981, 19.24484030382106781, 11.99618178085344589 ) ) ;
#778=CARTESIAN_POINT ( 'NONE',  ( 1.859271017917182139E-15, 28.88124999877096499, 12.99999999999999289 ) ) ;
#779=CARTESIAN_POINT ( 'NONE',  ( 3.756430356249996994, -27.72812499938548569, 8.999999999999992895 ) ) ;
#780=CARTESIAN_POINT ( 'NONE',  ( -3.756430356249997882, 29.56562499938549138, 11.16877607737301226 ) ) ;
#783=AXIS2_PLACEMENT_3D ( 'NONE', #21558, #5346, #13473 ) ;
#784=CARTESIAN_POINT ( 'NONE',  ( 1.071796769724487230, -25.13259618943233420, 4.999999999999992006 ) ) ;
#785=PLANE ( 'NONE',  #21415 ) ;
#786=ORIENTED_EDGE ( 'NONE', *, *, #24587, .F. ) ;
#790=VECTOR ( 'NONE', #20010, 1000.000000000000000 ) ;
#794=ORIENTED_EDGE ( 'NONE', *, *, #11379, .T. ) ;
#796=CARTESIAN_POINT ( 'NONE',  ( 27.09999999999999787, -0.5999999999999998668, 19.00000000000000000 ) ) ;
#799=CARTESIAN_POINT ( 'NONE',  ( -1.878215178124998497, 29.15312499938548640, 12.25316411605951927 ) ) ;
#805=CARTESIAN_POINT ( 'NONE',  ( 3.756430356250003655, 25.70312499938548356, 8.999999999999992895 ) ) ;
#815=CYLINDRICAL_SURFACE ( 'NONE', #1171, 4.000000000000000000 ) ;
#825=CARTESIAN_POINT ( 'NONE',  ( 1.878215178124998497, -26.00312499938548783, 12.25316411605951927 ) ) ;
#827=CARTESIAN_POINT ( 'NONE',  ( 23.26836714124207361, 18.93629030671969460, 11.57226653943512851 ) ) ;
#833=CARTESIAN_POINT ( 'NONE',  ( 3.999999999999995559, -27.43750000000000000, 6.690598923241487306 ) ) ;
#835=FACE_OUTER_BOUND ( 'NONE', #22363, .T. ) ;
#836=CARTESIAN_POINT ( 'NONE',  ( 3.834746474454188013E-15, 28.20624999877096428, 4.999999999999992006 ) ) ;
#837=CARTESIAN_POINT ( 'NONE',  ( 16.97706434298888212, 22.28945909890755317, 11.16877607737301226 ) ) ;
#839=CARTESIAN_POINT ( 'NONE',  ( 3.756430356250003655, 29.19062499938548072, 8.999999999999992895 ) ) ;
#842=CARTESIAN_POINT ( 'NONE',  ( 16.95282131294928263, 19.60901869090858796, 5.746835883940462963 ) ) ;
#843=CARTESIAN_POINT ( 'NONE',  ( 20.85081121023834427, 15.19395696074590596, 6.690598923241489970 ) ) ;
#845=CARTESIAN_POINT ( 'NONE',  ( -1.071796769724494336, -25.09240381056766367, 4.999999999999992895 ) ) ;
#848=CARTESIAN_POINT ( 'NONE',  ( -1.878215178125000939, -26.41562499938548214, 12.25316411605952283 ) ) ;
#852=CARTESIAN_POINT ( 'NONE',  ( 4.000000000000003553, 29.89374999877096784, 8.999999999999992895 ) ) ;
#862=CARTESIAN_POINT ( 'NONE',  ( 1.878215178124995832, -27.20312499938548711, 5.746835883940462963 ) ) ;
#863=DIRECTION ( 'NONE',  ( 0.000000000000000000, 0.000000000000000000, -1.000000000000000000 ) ) ;
#872=CARTESIAN_POINT ( 'NONE',  ( 16.57281518405975262, 22.22966943355206126, 6.690598923241487306 ) ) ;
#874=CARTESIAN_POINT ( 'NONE',  ( 1.878215178125000939, 25.51562499938548356, 12.25316411605952283 ) ) ;
#876=CARTESIAN_POINT ( 'NONE',  ( 15.00834143068450999, 20.66519568017682573, 8.999999999999992895 ) ) ;
#877=CARTESIAN_POINT ( 'NONE',  ( 19.76811771667562567, 17.11192033871618534, 12.25316411605952283 ) ) ;
#879=CYLINDRICAL_SURFACE ( 'NONE', #12623, 4.000000000000000000 ) ;
#883=CARTESIAN_POINT ( 'NONE',  ( -3.469446951953614189E-15, -30.00000000000000355, 4.999999999999992006 ) ) ;
#885=CARTESIAN_POINT ( 'NONE',  ( 4.000000000000003553, 25.39374999877096784, 8.999999999999992895 ) ) ;
#888=CARTESIAN_POINT ( 'NONE',  ( -3.999999999999996003, 27.83124999877096784, 6.690598923241487306 ) ) ;
#889=CARTESIAN_POINT ( 'NONE',  ( 1.878215178124995832, -27.99062499938548143, 5.746835883940462963 ) ) ;
#891=CARTESIAN_POINT ( 'NONE',  ( -1.071796769724487230, 25.31740381056767220, 12.99999999999999467 ) ) ;
#896=CARTESIAN_POINT ( 'NONE',  ( 1.878215178124995832, -26.64062499938548711, 5.746835883940462963 ) ) ;
#905=( BOUNDED_CURVE ( )  B_SPLINE_CURVE ( 2, ( #836, #22811, #4886, #22547, #12860, #20838, #2928, #10889, #5157 ),
 .UNSPECIFIED., .F., .F. ) 
 B_SPLINE_CURVE_WITH_KNOTS ( ( 3, 2, 2, 2, 3 ),
 ( 0.6250000000000000000, 0.6333333333333333037, 0.6500000000000000222, 0.6666666666666666297, 0.6750000000000000444 ),
 .UNSPECIFIED. ) 
 CURVE ( )  GEOMETRIC_REPRESENTATION_ITEM ( )  RATIONAL_B_SPLINE_CURVE ( ( 0.9330127018922194093, 0.9330127018922194093, 1.000000000000000000, 0.8660254037844387076, 1.000000000000000000, 0.8660254037844387076, 1.000000000000000000, 0.9330127018922189652, 0.9330127018922194093 ) ) 
 REPRESENTATION_ITEM ( '' )  );
#909=CARTESIAN_POINT ( 'NONE',  ( 21.21320343559646915, 21.21320343559638744, 12.99999999999999289 ) ) ;
#911=CARTESIAN_POINT ( 'NONE',  ( -1.878215178124998497, 27.69062499938548427, 12.25316411605951927 ) ) ;
#912=CARTESIAN_POINT ( 'NONE',  ( 16.91752973988819164, 22.57438398938050028, 8.999999999999992895 ) ) ;
#916=CARTESIAN_POINT ( 'NONE',  ( 22.71619846896431483, 19.59662171127745367, 12.34935938736417071 ) ) ;
#919=CARTESIAN_POINT ( 'NONE',  ( -3.756430356250004099, -27.99062499938548498, 6.831223922626973533 ) ) ;
#920=VECTOR ( 'NONE', #11822, 1000.000000000000000 ) ;
#925=EDGE_CURVE ( 'NONE', #2876, #7537, #14389, .T. ) ;
#926=CARTESIAN_POINT ( 'NONE',  ( 1.057460391440397258E-14, -28.71250000000000213, 4.999999999999992006 ) ) ;
#933=VERTEX_POINT ( 'NONE', #17905 ) ;
#936=ORIENTED_EDGE ( 'NONE', *, *, #14930, .F. ) ;
#939=VERTEX_POINT ( 'NONE', #5622 ) ;
#941=CARTESIAN_POINT ( 'NONE',  ( -3.756430356249997438, 28.66562499938548569, 11.16877607737301048 ) ) ;
#947=CARTESIAN_POINT ( 'NONE',  ( 18.11727402765218287, 23.42966878357085037, 6.831223922626973533 ) ) ;
#949=CARTESIAN_POINT ( 'NONE',  ( -1.878215178124995832, 26.75312499938548783, 5.746835883940462963 ) ) ;
#950=CARTESIAN_POINT ( 'NONE',  ( -20.67279826512042007, -15.85973458909327150, 20.00001200000000168 ) ) ;
#952=LINE ( 'NONE', #11007, #17147 ) ;
#954=CARTESIAN_POINT ( 'NONE',  ( 20.26302869750798408, 20.26302869750790947, 4.999999999999992006 ) ) ;
#957=CARTESIAN_POINT ( 'NONE',  ( 2.000000000000003997, 27.71874999877097068, 5.535898384862238508 ) ) ;
#961=VERTEX_POINT ( 'NONE', #19858 ) ;
#965=CARTESIAN_POINT ( 'NONE',  ( -1.878215178125004048, -25.32812499938548356, 5.746835883940462963 ) ) ;
#967=PLANE ( 'NONE',  #8845 ) ;
#969=ORIENTED_EDGE ( 'NONE', *, *, #11626, .T. ) ;
#970=CARTESIAN_POINT ( 'NONE',  ( 3.999999999999996447, -29.27500000000000213, 8.999999999999992895 ) ) ;
#972=CARTESIAN_POINT ( 'NONE',  ( 17.74838020778238246, 20.57680733252850303, 12.46410161513774639 ) ) ;
#976=CARTESIAN_POINT ( 'NONE',  ( 21.04090992281141581, 18.38471254485196837, 12.25316411605952283 ) ) ;
#978=CARTESIAN_POINT ( 'NONE',  ( 2.000000000000003997, 26.87500000000000355, 5.535898384862238508 ) ) ;
#979=CARTESIAN_POINT ( 'NONE',  ( 20.08631576820957321, 17.43011839025013288, 12.25316411605952283 ) ) ;
#983=CARTESIAN_POINT ( 'NONE',  ( -3.735045420075836212E-15, -27.95312499938548001, 4.662447845253954171 ) ) ;
#987=LINE ( 'NONE', #19022, #11275 ) ;
#990=VERTEX_POINT ( 'NONE', #9919 ) ;
#991=DIRECTION ( 'NONE',  ( 0.000000000000000000, -1.000000000000000000, 0.000000000000000000 ) ) ;
#994=ORIENTED_EDGE ( 'NONE', *, *, #24626, .F. ) ;
#995=CARTESIAN_POINT ( 'NONE',  ( -3.999999999999996447, 25.67500000000000071, 8.999999999999992895 ) ) ;
#1003=CARTESIAN_POINT ( 'NONE',  ( 3.959305671612554781E-15, 30.00000000000000355, 12.99999999999999289 ) ) ;
#1008=CARTESIAN_POINT ( 'NONE',  ( 1.878215178125000939, 27.31562499938548427, 12.25316411605952283 ) ) ;
#1009=CARTESIAN_POINT ( 'NONE',  ( 21.76563060752939549, 16.10877635803693764, 6.690598923241489970 ) ) ;
#1010=CARTESIAN_POINT ( 'NONE',  ( 19.35704813498177046, 16.52862101023551844, 12.46410161513774817 ) ) ;
#1011=CARTESIAN_POINT ( 'NONE',  ( 20.51057983692150444, 17.85438245896205700, 5.746835883940462963 ) ) ;
#1015=( BOUNDED_SURFACE ( )  B_SPLINE_SURFACE ( 1, 2, ( 
 ( #20359, #23917, #22212, #24040, #19970, #12521, #4299, #10557, #20237, #8483, #12270, #2334, #7960, #4030, #8345, #24161, #25873, #15946, #11996, #2075, #6121, #14105, #22069, #10417, #4158, #12134, #20111, #2215, #10172, #16469, #14242, #22336, #10294, #374, #16333, #6387, #14377, #24545, #18556, #18669, #2717, #10807, #19051, #22987, #4931, #2978, #20635, #10946, #21149, #3220, #1136, #8725, #10680, #7159, #13051, #18937, #16856, #22735, #637, #755, #20891, #8605, #20761, #5072, #25073, #888, #1021, #16712, #4814, #24940, #12914, #16586, #13179, #6630, #14622, #16975, #8995, #24821, #3108, #5200, #12789, #21029, #2840, #6898, #12664, #11073, #22602, #9109, #17098, #14881, #4685, #24687, #7020, #22856, #6772, #14757, #15150, #15006, #18800, #8872, #23118, #7886, #3355, #13298, #17836, #2147, #21890, #21272, #188, #11330, #16015, #6182, #11938, #19908, #2007, #15386, #14171, #9977, #3973, #6062, #17968 ),
 ( #24100, #11192, #5935, #19313, #12064, #23981, #58, #23359, #5448, #14046, #15876, #1408, #9383, #25805, #10112, #8031, #17362, #8158, #25327, #22011, #22143, #4089, #20043, #18113, #13440, #19172, #16139, #1269, #9253, #17241, #21410, #25211, #5318, #7291, #15267, #23235, #7407, #23848, #3491, #13920, #11462, #19793, #1890, #9854, #25768, #1856, #7848, #15589, #17680, #19760, #9554, #1972, #5894, #9938, #17923, #15714, #13880, #13620, #1723, #9698, #15979, #2102, #21853, #15833, #14, #23559, #19999, #3936, #11904, #11783, #5640, #9817, #14130, #17802, #21585, #3665, #23942, #17543, #19872, #6025, #4052, #21977, #7990, #14007, #25518, #12021, #24064, #10070, #18071, #11643, #153, #19618, #25649, #7605, #23806, #7729, #23677, #5754, #8124, #6146, #16099, #13741, #22096, #21718, #4185, #3803, #19489, #1585, #12691, #4569, #10706, #16609, #18446, #16364, #22760, #780, #4719, #8245, #8631, #22632, #12162 ) ),
 .UNSPECIFIED., .F., .F., .T. ) 
 B_SPLINE_SURFACE_WITH_KNOTS ( ( 2, 2 ),
 ( 3, 2, 2, 2, 2, 2, 2, 2, 2, 2, 2, 2, 2, 2, 2, 2, 2, 2, 2, 2, 2, 2, 2, 2, 2, 2, 2, 2, 2, 2, 2, 2, 2, 2, 2, 2, 2, 2, 2, 2, 2, 2, 2, 2, 2, 2, 2, 2, 2, 2, 2, 2, 2, 2, 2, 2, 2, 2, 2, 2, 3 ),
 ( 0.000000000000000000, 1.000000000000000000 ),
 ( 0.000000000000000000, 0.01666666666666666644, 0.03333333333333333287, 0.05000000000000000278, 0.06666666666666666574, 0.08333333333333332871, 0.1000000000000000056, 0.1166666666666666685, 0.1333333333333333315, 0.1499999999999999944, 0.1666666666666666574, 0.1833333333333333204, 0.2000000000000000111, 0.2166666666666666741, 0.2333333333333333370, 0.2500000000000000000, 0.2666666666666666630, 0.2833333333333333259, 0.2999999999999999889, 0.3166666666666666519, 0.3333333333333333148, 0.3499999999999999778, 0.3666666666666666408, 0.3833333333333333592, 0.4000000000000000222, 0.4166666666666666852, 0.4333333333333333481, 0.4500000000000000111, 0.4666666666666666741, 0.4833333333333333370, 0.5000000000000000000, 0.5166666666666667185, 0.5333333333333333259, 0.5500000000000000444, 0.5666666666666666519, 0.5833333333333333703, 0.5999999999999999778, 0.6166666666666666963, 0.6333333333333333037, 0.6500000000000000222, 0.6666666666666666297, 0.6833333333333333481, 0.6999999999999999556, 0.7166666666666666741, 0.7333333333333332815, 0.7500000000000000000, 0.7666666666666667185, 0.7833333333333333259, 0.8000000000000000444, 0.8166666666666666519, 0.8333333333333333703, 0.8499999999999999778, 0.8666666666666666963, 0.8833333333333333037, 0.9000000000000000222, 0.9166666666666666297, 0.9333333333333333481, 0.9499999999999999556, 0.9666666666666666741, 0.9833333333333332815, 1.000000000000000000 ),
 .UNSPECIFIED. ) 
 GEOMETRIC_REPRESENTATION_ITEM ( )  RATIONAL_B_SPLINE_SURFACE ( (
 ( 1.000000000000000000, 0.8660254037844387076, 1.000000000000000000, 0.8660254037844387076, 1.000000000000000000, 0.8660254037844387076, 1.000000000000000000, 0.8660254037844387076, 1.000000000000000000, 0.8660254037844387076, 1.000000000000000000, 0.8660254037844387076, 1.000000000000000000, 0.8660254037844387076, 1.000000000000000000, 0.8660254037844387076, 1.000000000000000000, 0.8660254037844387076, 1.000000000000000000, 0.8660254037844387076, 1.000000000000000000, 0.8660254037844387076, 1.000000000000000000, 0.8660254037844387076, 1.000000000000000000, 0.8660254037844387076, 1.000000000000000000, 0.8660254037844387076, 1.000000000000000000, 0.8660254037844387076, 1.000000000000000000, 0.8660254037844387076, 1.000000000000000000, 0.8660254037844387076, 1.000000000000000000, 0.8660254037844387076, 1.000000000000000000, 0.8660254037844387076, 1.000000000000000000, 0.8660254037844387076, 1.000000000000000000, 0.8660254037844387076, 1.000000000000000000, 0.8660254037844387076, 1.000000000000000000, 0.8660254037844387076, 1.000000000000000000, 0.8660254037844387076, 1.000000000000000000, 0.8660254037844387076, 1.000000000000000000, 0.8660254037844387076, 1.000000000000000000, 0.8660254037844387076, 1.000000000000000000, 0.8660254037844387076, 1.000000000000000000, 0.8660254037844387076, 1.000000000000000000, 0.8660254037844387076, 1.000000000000000000, 0.8660254037844387076, 1.000000000000000000, 0.8660254037844387076, 1.000000000000000000, 0.8660254037844387076, 1.000000000000000000, 0.8660254037844387076, 1.000000000000000000, 0.8660254037844387076, 1.000000000000000000, 0.8660254037844387076, 1.000000000000000000, 0.8660254037844387076, 1.000000000000000000, 0.8660254037844387076, 1.000000000000000000, 0.8660254037844387076, 1.000000000000000000, 0.8660254037844387076, 1.000000000000000000, 0.8660254037844387076, 1.000000000000000000, 0.8660254037844387076, 1.000000000000000000, 0.8660254037844387076, 1.000000000000000000, 0.8660254037844387076, 1.000000000000000000, 0.8660254037844387076, 1.000000000000000000, 0.8660254037844387076, 1.000000000000000000, 0.8660254037844387076, 1.000000000000000000, 0.8660254037844387076, 1.000000000000000000, 0.8660254037844387076, 1.000000000000000000, 0.8660254037844387076, 1.000000000000000000, 0.8660254037844387076, 1.000000000000000000, 0.8660254037844387076, 1.000000000000000000, 0.8660254037844387076, 1.000000000000000000, 0.8660254037844387076, 1.000000000000000000, 0.8660254037844387076, 1.000000000000000000, 0.8660254037844387076, 1.000000000000000000, 0.8660254037844387076, 1.000000000000000000, 0.8660254037844387076, 1.000000000000000000, 0.8660254037844387076, 1.000000000000000000, 0.8660254037844387076, 1.000000000000000000),
 ( 1.000000000000000000, 0.8660254037844387076, 1.000000000000000000, 0.8660254037844387076, 1.000000000000000000, 0.8660254037844387076, 1.000000000000000000, 0.8660254037844387076, 1.000000000000000000, 0.8660254037844387076, 1.000000000000000000, 0.8660254037844387076, 1.000000000000000000, 0.8660254037844387076, 1.000000000000000000, 0.8660254037844387076, 1.000000000000000000, 0.8660254037844387076, 1.000000000000000000, 0.8660254037844387076, 1.000000000000000000, 0.8660254037844387076, 1.000000000000000000, 0.8660254037844387076, 1.000000000000000000, 0.8660254037844387076, 1.000000000000000000, 0.8660254037844387076, 1.000000000000000000, 0.8660254037844387076, 1.000000000000000000, 0.8660254037844387076, 1.000000000000000000, 0.8660254037844387076, 1.000000000000000000, 0.8660254037844387076, 1.000000000000000000, 0.8660254037844387076, 1.000000000000000000, 0.8660254037844387076, 1.000000000000000000, 0.8660254037844387076, 1.000000000000000000, 0.8660254037844387076, 1.000000000000000000, 0.8660254037844387076, 1.000000000000000000, 0.8660254037844387076, 1.000000000000000000, 0.8660254037844387076, 1.000000000000000000, 0.8660254037844387076, 1.000000000000000000, 0.8660254037844387076, 1.000000000000000000, 0.8660254037844387076, 1.000000000000000000, 0.8660254037844387076, 1.000000000000000000, 0.8660254037844387076, 1.000000000000000000, 0.8660254037844387076, 1.000000000000000000, 0.8660254037844387076, 1.000000000000000000, 0.8660254037844387076, 1.000000000000000000, 0.8660254037844387076, 1.000000000000000000, 0.8660254037844387076, 1.000000000000000000, 0.8660254037844387076, 1.000000000000000000, 0.8660254037844387076, 1.000000000000000000, 0.8660254037844387076, 1.000000000000000000, 0.8660254037844387076, 1.000000000000000000, 0.8660254037844387076, 1.000000000000000000, 0.8660254037844387076, 1.000000000000000000, 0.8660254037844387076, 1.000000000000000000, 0.8660254037844387076, 1.000000000000000000, 0.8660254037844387076, 1.000000000000000000, 0.8660254037844387076, 1.000000000000000000, 0.8660254037844387076, 1.000000000000000000, 0.8660254037844387076, 1.000000000000000000, 0.8660254037844387076, 1.000000000000000000, 0.8660254037844387076, 1.000000000000000000, 0.8660254037844387076, 1.000000000000000000, 0.8660254037844387076, 1.000000000000000000, 0.8660254037844387076, 1.000000000000000000, 0.8660254037844387076, 1.000000000000000000, 0.8660254037844387076, 1.000000000000000000, 0.8660254037844387076, 1.000000000000000000, 0.8660254037844387076, 1.000000000000000000, 0.8660254037844387076, 1.000000000000000000, 0.8660254037844387076, 1.000000000000000000, 0.8660254037844387076, 1.000000000000000000, 0.8660254037844387076, 1.000000000000000000) ) ) 
 REPRESENTATION_ITEM ( '' )  SURFACE ( )  );
#1017=CARTESIAN_POINT ( 'NONE',  ( 21.38789795289476103, 16.07550319697594432, 8.999999999999992895 ) ) ;
#1019=ORIENTED_EDGE ( 'NONE', *, *, #4892, .T. ) ;
#1021=CARTESIAN_POINT ( 'NONE',  ( -3.999999999999996447, 27.86874999877096570, 8.999999999999992895 ) ) ;
#1022=CARTESIAN_POINT ( 'NONE',  ( 3.999999999999996447, -25.22500000000000142, 8.999999999999992895 ) ) ;
#1025=CARTESIAN_POINT ( 'NONE',  ( 18.05905254985559338, 19.57480207770756664, 12.99999999999999467 ) ) ;
#1027=CARTESIAN_POINT ( 'NONE',  ( -3.756430356250002323, -28.70312499938548356, 11.16877607737301226 ) ) ;
#1028=ORIENTED_EDGE ( 'NONE', *, *, #14569, .T. ) ;
#1029=ORIENTED_EDGE ( 'NONE', *, *, #11563, .T. ) ;
#1030=CARTESIAN_POINT ( 'NONE',  ( 20.28164449898397947, 22.10686971680496882, 5.204870533884474959 ) ) ;
#1037=CARTESIAN_POINT ( 'NONE',  ( -1.878215178124998497, 27.24062499938548498, 12.25316411605951927 ) ) ;
#1046=CARTESIAN_POINT ( 'NONE',  ( -3.735045420075836212E-15, -28.06562499938548427, 4.662447845253954171 ) ) ;
#1047=CARTESIAN_POINT ( 'NONE',  ( 18.55713358789543932, 21.38556071264155634, 5.535898384862237620 ) ) ;
#1049=CARTESIAN_POINT ( 'NONE',  ( -1.999999999999995781, 25.99374999877096926, 5.535898384862237620 ) ) ;
#1057=ORIENTED_EDGE ( 'NONE', *, *, #1504, .F. ) ;
#1059=CARTESIAN_POINT ( 'NONE',  ( -1.071796769724498999, -27.60759618943233207, 12.99999999999998757 ) ) ;
#1062=CARTESIAN_POINT ( 'NONE',  ( 3.756430356250003211, 27.99062499938548498, 6.831223922626973533 ) ) ;
#1064=ADVANCED_FACE ( 'NONE', ( #24442 ), #12677, .F. ) ;
#1066=CARTESIAN_POINT ( 'NONE',  ( 23.29708626209844269, 17.98469150617961887, 8.999999999999992895 ) ) ;
#1067=DIRECTION ( 'NONE',  ( -0.000000000000000000, -0.000000000000000000, 1.000000000000000000 ) ) ;
#1072=DIRECTION ( 'NONE',  ( -0.7071067811865487940, -0.7071067811865463515, 0.000000000000000000 ) ) ;
#1077=CARTESIAN_POINT ( 'NONE',  ( -1.071796769724494558, -25.54240381056766651, 4.999999999999992895 ) ) ;
#1084=CARTESIAN_POINT ( 'NONE',  ( -2.672651547586948120E-15, -26.04062499938548925, 13.33755215474602984 ) ) ;
#1092=CARTESIAN_POINT ( 'NONE',  ( 15.67775563255858984, 20.99015038847727155, 8.999999999999992895 ) ) ;
#1095=CARTESIAN_POINT ( 'NONE',  ( -1.878215178124995832, 29.34062499938548285, 5.746835883940462963 ) ) ;
#1096=EDGE_CURVE ( 'NONE', #4544, #12039, #7136, .T. ) ;
#1097=CARTESIAN_POINT ( 'NONE',  ( 21.17576591853880075, 15.86337116261998048, 6.831223922626973533 ) ) ;
#1098=CARTESIAN_POINT ( 'NONE',  ( 3.469446951953614189E-15, 30.00000000000000355, 8.999999999999992895 ) ) ;
#1101=CARTESIAN_POINT ( 'NONE',  ( 1.878215178124998497, -27.69062499938548427, 12.25316411605951927 ) ) ;
#1103=CARTESIAN_POINT ( 'NONE',  ( 25.99307600111999150, -0.5999999999999998668, 20.00001200000000168 ) ) ;
#1105=CARTESIAN_POINT ( 'NONE',  ( 0.5788183228083377818, 29.99578766836522092, 12.96878440844335678 ) ) ;
#1111=VERTEX_POINT ( 'NONE', #20862 ) ;
#1112=CARTESIAN_POINT ( 'NONE',  ( -3.735045420075836212E-15, -29.41562499938548569, 4.662447845253954171 ) ) ;
#1113=CARTESIAN_POINT ( 'NONE',  ( 4.000000000000003553, 25.93750000000000000, 6.690598923241489970 ) ) ;
#1115=CARTESIAN_POINT ( 'NONE',  ( 20.94803839265150458, 18.11961126790524901, 12.46410161513774817 ) ) ;
#1119=CARTESIAN_POINT ( 'NONE',  ( -1.999999999999995781, 26.95000000000000284, 5.535898384862237620 ) ) ;
#1123=CARTESIAN_POINT ( 'NONE',  ( -1.878215178124995832, 26.64062499938548711, 5.746835883940462963 ) ) ;
#1124=CARTESIAN_POINT ( 'NONE',  ( -4.000000000000002665, -29.73213749463701205, 8.735714247490120599 ) ) ;
#1125=CARTESIAN_POINT ( 'NONE',  ( 17.85210898470722896, 23.16450374062589646, 11.16877607737301226 ) ) ;
#1126=CARTESIAN_POINT ( 'NONE',  ( 22.49925389301043666, 19.67082676826417398, 12.46410161513774817 ) ) ;
#1127=CARTESIAN_POINT ( 'NONE',  ( 17.26224429571663066, 22.91909854520893930, 11.30940107675849404 ) ) ;
#1130=EDGE_CURVE ( 'NONE', #17660, #23467, #24227, .T. ) ;
#1131=CARTESIAN_POINT ( 'NONE',  ( 20.43103032403801578, 17.77483294607857189, 5.746835883940462963 ) ) ;
#1132=CARTESIAN_POINT ( 'NONE',  ( 3.137519842735244810E-15, -26.85624999877096641, 4.999999999999991118 ) ) ;
#1136=CARTESIAN_POINT ( 'NONE',  ( 2.000000000000003997, 27.26874999877097139, 5.535898384862238508 ) ) ;
#1137=CARTESIAN_POINT ( 'NONE',  ( 1.878215178124998497, -29.49062499938548498, 12.25316411605951927 ) ) ;
#1138=CARTESIAN_POINT ( 'NONE',  ( 5.577813053751546416E-15, 25.33750000000000213, 12.99999999999999289 ) ) ;
#1142=CARTESIAN_POINT ( 'NONE',  ( -3.756430356250003655, -27.39062499938548356, 8.999999999999992895 ) ) ;
#1146=CARTESIAN_POINT ( 'NONE',  ( 18.29814930579269827, 23.77352349748025517, 7.961019890438434388 ) ) ;
#1150=ADVANCED_FACE ( 'NONE', ( #17075 ), #10655, .F. ) ;
#1151=DIRECTION ( 'NONE',  ( 0.000000000000000000, 1.000000000000000000, 0.000000000000000000 ) ) ;
#1153=CYLINDRICAL_SURFACE ( 'NONE', #17186, 4.000000000000000000 ) ;
#1156=CARTESIAN_POINT ( 'NONE',  ( -3.834746474454188013E-15, -25.56250000000000000, 4.999999999999992006 ) ) ;
#1159=CARTESIAN_POINT ( 'NONE',  ( -2.672651547586948120E-15, -29.64062499938548356, 13.33755215474602984 ) ) ;
#1163=CARTESIAN_POINT ( 'NONE',  ( 8.831537335106614961E-15, 27.13750000000000284, 12.99999999999999112 ) ) ;
#1164=CARTESIAN_POINT ( 'NONE',  ( 3.595408253811773758, -29.78394301743083261, 10.77252090037689136 ) ) ;
#1170=ORIENTED_EDGE ( 'NONE', *, *, #23564, .T. ) ;
#1171=AXIS2_PLACEMENT_3D ( 'NONE', #304, #18486, #14429 ) ;
#1173=VERTEX_POINT ( 'NONE', #5181 ) ;
#1175=VERTEX_POINT ( 'NONE', #16952 ) ;
#1180=CARTESIAN_POINT ( 'NONE',  ( -30.00000000000000355, 0.000000000000000000, 20.00000000000000000 ) ) ;
#1183=CARTESIAN_POINT ( 'NONE',  ( 19.92494326818769323, 19.92494326818762218, 13.33755215474602984 ) ) ;
#1184=CARTESIAN_POINT ( 'NONE',  ( 3.756430356250004099, 26.19062499938548783, 6.831223922626973533 ) ) ;
#1185=CARTESIAN_POINT ( 'NONE',  ( -4.000000000000001776, -26.70624999877097139, 11.30940107675849760 ) ) ;
#1192=CARTESIAN_POINT ( 'NONE',  ( 17.48763458135079318, 23.14448883084309827, 6.690598923241487306 ) ) ;
#1193=CARTESIAN_POINT ( 'NONE',  ( -3.752267015613588906E-15, -25.50624999877097565, 4.381197846482986158 ) ) ;
#1199=ORIENTED_EDGE ( 'NONE', *, *, #5496, .T. ) ;
#1205=CARTESIAN_POINT ( 'NONE',  ( -3.735045420075836212E-15, -26.71562499938548640, 4.662447845253954171 ) ) ;
#1208=DIRECTION ( 'NONE',  ( 0.000000000000000000, 1.000000000000000000, 0.000000000000000000 ) ) ;
#1210=ADVANCED_FACE ( 'NONE', ( #3711 ), #1900, .F. ) ;
#1216=CARTESIAN_POINT ( 'NONE',  ( 1.071796769724487230, -27.38259618943233420, 4.999999999999992006 ) ) ;
#1221=CARTESIAN_POINT ( 'NONE',  ( 16.31415173562648491, 21.62654649154516306, 8.999999999999992895 ) ) ;
#1223=CARTESIAN_POINT ( 'NONE',  ( 1.878215178125000939, 29.56562499938548427, 12.25316411605952283 ) ) ;
#1224=CARTESIAN_POINT ( 'NONE',  ( 21.44093096148375466, 16.12853620556493794, 11.16877607737301403 ) ) ;
#1225=FACE_OUTER_BOUND ( 'NONE', #6945, .T. ) ;
#1228=VERTEX_POINT ( 'NONE', #17343 ) ;
#1234=DIRECTION ( 'NONE',  ( 0.000000000000000000, 1.000000000000000000, 0.000000000000000000 ) ) ;
#1242=CARTESIAN_POINT ( 'NONE',  ( 3.756430356249996105, -29.04062499938548569, 6.831223922626973533 ) ) ;
#1247=CARTESIAN_POINT ( 'NONE',  ( 21.05410440982949183, 18.22567728508322205, 5.535898384862238508 ) ) ;
#1255=CARTESIAN_POINT ( 'NONE',  ( 1.878215178125000939, 26.86562499938548498, 12.25316411605952283 ) ) ;
#1257=CARTESIAN_POINT ( 'NONE',  ( -2.444316569969958497, -29.90105888194226580, 5.822820249163556561 ) ) ;
#1258=CARTESIAN_POINT ( 'NONE',  ( 17.53391093317328142, 22.84630568909195958, 11.16877607737301226 ) ) ;
#1259=CARTESIAN_POINT ( 'NONE',  ( 19.55598568231966539, 16.89978830436022150, 5.746835883940462963 ) ) ;
#1263=CARTESIAN_POINT ( 'NONE',  ( -3.469446951953614189E-15, -25.00000000000000000, 8.999999999999992895 ) ) ;
#1265=CARTESIAN_POINT ( 'NONE',  ( 17.18919637734483885, 22.50159113326351346, 8.999999999999992895 ) ) ;
#1266=CARTESIAN_POINT ( 'NONE',  ( 21.51241069055853927, 19.99666116270642036, 12.99999999999999467 ) ) ;
#1268=CARTESIAN_POINT ( 'NONE',  ( 21.46069080901174786, 15.80383655951930066, 8.999999999999992895 ) ) ;
#1269=CARTESIAN_POINT ( 'NONE',  ( 3.735045420075836212E-15, 26.26562499938548356, 4.662447845253954171 ) ) ;
#1270=CARTESIAN_POINT ( 'NONE',  ( -3.756430356250003655, -29.19062499938548072, 8.999999999999992895 ) ) ;
#1275=ORIENTED_EDGE ( 'NONE', *, *, #7993, .T. ) ;
#1276=CARTESIAN_POINT ( 'NONE',  ( -3.756430356250002323, -28.25312499938548427, 11.16877607737301226 ) ) ;
#1278=EDGE_LOOP ( 'NONE', ( #4589, #25272, #5489, #14857 ) ) ;
#1288=CARTESIAN_POINT ( 'NONE',  ( -4.000000000000003553, -27.25000000000000000, 8.999999999999992895 ) ) ;
#1294=FACE_OUTER_BOUND ( 'NONE', #19245, .T. ) ;
#1296=DIRECTION ( 'NONE',  ( 0.7071067811865487940, 0.7071067811865463515, -0.000000000000000000 ) ) ;
#1297=LINE ( 'NONE', #23257, #6343 ) ;
#1298=CARTESIAN_POINT ( 'NONE',  ( 3.756430356249997882, -29.11562499938548143, 11.16877607737301226 ) ) ;
#1301=VECTOR ( 'NONE', #19260, 1000.000000000000000 ) ;
#1302=CARTESIAN_POINT ( 'NONE',  ( -27.10000000000000497, -0.5999999999999998668, 19.59999999999999787 ) ) ;
#1306=CARTESIAN_POINT ( 'NONE',  ( 1.071796769724488563, -27.06115380933863435, 12.99999999999999289 ) ) ;
#1308=CARTESIAN_POINT ( 'NONE',  ( 21.21320343559646915, 21.21320343559638744, 12.99999999999999289 ) ) ;
#1312=ORIENTED_EDGE ( 'NONE', *, *, #25575, .F. ) ;
#1316=DIRECTION ( 'NONE',  ( 0.000000000000000000, 0.000000000000000000, -1.000000000000000000 ) ) ;
#1318=CYLINDRICAL_SURFACE ( 'NONE', #6505, 4.000000000000000000 ) ;
#1321=EDGE_CURVE ( 'NONE', #10871, #23470, #3412, .T. ) ;
#1322=VECTOR ( 'NONE', #7540, 1000.000000000000000 ) ;
#1328=CARTESIAN_POINT ( 'NONE',  ( -3.756430356249997882, 25.51562499938548356, 11.16877607737301226 ) ) ;
#1337=CARTESIAN_POINT ( 'NONE',  ( 19.51936408540558077, 21.03511361325754692, 4.999999999999992006 ) ) ;
#1338=CARTESIAN_POINT ( 'NONE',  ( 3.999999999999996447, -26.06874999877096855, 8.999999999999992895 ) ) ;
#1342=DIRECTION ( 'NONE',  ( 0.000000000000000000, 0.000000000000000000, 1.000000000000000000 ) ) ;
#1348=VERTEX_POINT ( 'NONE', #20279 ) ;
#1349=CARTESIAN_POINT ( 'NONE',  ( -1.878215178125004048, -28.92812499938548854, 5.746835883940462963 ) ) ;
#1352=VECTOR ( 'NONE', #18435, 1000.000000000000000 ) ;
#1353=VECTOR ( 'NONE', #17499, 1000.000000000000000 ) ;
#1357=DIRECTION ( 'NONE',  ( 1.000000000000000000, 0.000000000000000000, 0.000000000000000000 ) ) ;
#1362=CARTESIAN_POINT ( 'NONE',  ( 20.85756786700484966, 15.54517311108603472, 6.831223922626973533 ) ) ;
#1366=CARTESIAN_POINT ( 'NONE',  ( 2.000000000000003997, 25.52500000000000213, 5.535898384862238508 ) ) ;
#1368=CARTESIAN_POINT ( 'NONE',  ( 19.20899765223631661, 19.20899765223624200, 4.662447845253954171 ) ) ;
#1371=ORIENTED_EDGE ( 'NONE', *, *, #18568, .F. ) ;
#1373=CARTESIAN_POINT ( 'NONE',  ( 3.756430356249996994, -28.96562499938548285, 8.999999999999992895 ) ) ;
#1377=DIRECTION ( 'NONE',  ( 0.000000000000000000, 1.000000000000000000, 0.000000000000000000 ) ) ;
#1378=ORIENTED_EDGE ( 'NONE', *, *, #11699, .F. ) ;
#1384=CARTESIAN_POINT ( 'NONE',  ( -1.878215178125000939, -28.77812499938548640, 12.25316411605952283 ) ) ;
#1385=CARTESIAN_POINT ( 'NONE',  ( 0.000000000000000000, 0.000000000000000000, 17.00000000000000000 ) ) ;
#1394=EDGE_CURVE ( 'NONE', #7772, #25535, #6551, .T. ) ;
#1396=( GEOMETRIC_REPRESENTATION_CONTEXT ( 3 ) GLOBAL_UNCERTAINTY_ASSIGNED_CONTEXT ( ( #7042 ) ) GLOBAL_UNIT_ASSIGNED_CONTEXT ( ( #11728, #223, #13826 ) ) REPRESENTATION_CONTEXT ( 'NONE', 'WORKASPACE' ) );
#1397=CARTESIAN_POINT ( 'NONE',  ( 3.735045420075836212E-15, 27.05312499938548498, 4.662447845253954171 ) ) ;
#1399=CARTESIAN_POINT ( 'NONE',  ( 22.95237170627000367, 17.63997695035117985, 11.16877607737301226 ) ) ;
#1400=CARTESIAN_POINT ( 'NONE',  ( 20.64088888413906986, 20.64088888413900236, 13.33755215474602984 ) ) ;
#1404=CARTESIAN_POINT ( 'NONE',  ( 17.53391093317328142, 22.84630568909195958, 11.16877607737301048 ) ) ;
#1405=CARTESIAN_POINT ( 'NONE',  ( 20.68849525807644696, 19.17274573022432094, 4.999999999999992895 ) ) ;
#1408=CARTESIAN_POINT ( 'NONE',  ( 3.756430356250002323, 25.66562499938548569, 11.16877607737301226 ) ) ;
#1409=CARTESIAN_POINT ( 'NONE',  ( 3.756430356249997882, -29.00312499938548072, 11.16877607737301226 ) ) ;
#1415=CARTESIAN_POINT ( 'NONE',  ( 1.878215178124998497, -28.14062499938548356, 12.25316411605951927 ) ) ;
#1416=ORIENTED_EDGE ( 'NONE', *, *, #16411, .F. ) ;
#1423=CARTESIAN_POINT ( 'NONE',  ( -27.10000000000000497, 0.6000000000000000888, 19.00000000000000000 ) ) ;
#1425=DIRECTION ( 'NONE',  ( 0.000000000000000000, -1.000000000000000000, 0.000000000000000000 ) ) ;
#1427=CARTESIAN_POINT ( 'NONE',  ( -3.999999999999996447, 26.57500000000000284, 8.999999999999992895 ) ) ;
#1430=CARTESIAN_POINT ( 'NONE',  ( 21.07620149587250680, 15.41934724638005605, 11.30940107675849760 ) ) ;
#1433=CARTESIAN_POINT ( 'NONE',  ( 3.756430356249997882, -28.66562499938548569, 11.16877607737301226 ) ) ;
#1436=CARTESIAN_POINT ( 'NONE',  ( 18.23451611984813425, 18.23451611984805609, 12.99999999999999112 ) ) ;
#1438=CARTESIAN_POINT ( 'NONE',  ( 20.91578934480144625, 19.40003981694932733, 12.99999999999999467 ) ) ;
#1440=CARTESIAN_POINT ( 'NONE',  ( 3.999999999999996447, -26.96874999877096712, 8.999999999999992895 ) ) ;
#1450=( BOUNDED_CURVE ( )  B_SPLINE_CURVE ( 2, ( #24955, #20651, #14896, #8622, #12803, #20777, #2733, #5091, #2856 ),
 .UNSPECIFIED., .F., .F. ) 
 B_SPLINE_CURVE_WITH_KNOTS ( ( 3, 2, 2, 2, 3 ),
 ( 0.3750000000000000000, 0.3833333333333333592, 0.4000000000000000222, 0.4166666666666666852, 0.4250000000000000444 ),
 .UNSPECIFIED. ) 
 CURVE ( )  GEOMETRIC_REPRESENTATION_ITEM ( )  RATIONAL_B_SPLINE_CURVE ( ( 0.9330127018922194093, 0.9330127018922194093, 1.000000000000000000, 0.8660254037844387076, 1.000000000000000000, 0.8660254037844387076, 1.000000000000000000, 0.9330127018922191873, 0.9330127018922194093 ) ) 
 REPRESENTATION_ITEM ( '' )  );
#1455=SURFACE_SIDE_STYLE ('',( #19360 ) ) ;
#1456=CARTESIAN_POINT ( 'NONE',  ( 3.756430356250003655, 28.85312499938548569, 8.999999999999992895 ) ) ;
#1458=CARTESIAN_POINT ( 'NONE',  ( 1.071796769724494558, 28.63615380933863364, 4.999999999999992895 ) ) ;
#1460=CARTESIAN_POINT ( 'NONE',  ( -4.000000000000001776, -25.80624999877096926, 11.30940107675849760 ) ) ;
#1462=CARTESIAN_POINT ( 'NONE',  ( 18.87533163942939041, 21.70375876417550032, 5.535898384862237620 ) ) ;
#1463=CARTESIAN_POINT ( 'NONE',  ( 3.999999999999996003, -26.93124999877096926, 6.690598923241487306 ) ) ;
#1465=CYLINDRICAL_SURFACE ( 'NONE', #331, 4.000000000000000000 ) ;
#1468=ORIENTED_EDGE ( 'NONE', *, *, #14358, .T. ) ;
#1475=CARTESIAN_POINT ( 'NONE',  ( -3.756430356250002323, -27.91562499938548569, 11.16877607737301226 ) ) ;
#1484=CARTESIAN_POINT ( 'NONE',  ( 16.87327180006579752, 19.52946917802510285, 5.746835883940462963 ) ) ;
#1487=CARTESIAN_POINT ( 'NONE',  ( 4.000000000000003553, 26.83749999999999503, 6.690598923241489970 ) ) ;
#1488=CARTESIAN_POINT ( 'NONE',  ( 21.49396397007274473, 16.18156921415393157, 6.831223922626973533 ) ) ;
#1489=CARTESIAN_POINT ( 'NONE',  ( -3.137519842735244810E-15, 26.85624999877096641, 4.999999999999991118 ) ) ;
#1494=CARTESIAN_POINT ( 'NONE',  ( 3.756430356249997438, -29.45312499938548356, 11.16877607737301048 ) ) ;
#1504=EDGE_CURVE ( 'NONE', #11855, #2116, #230, .T. ) ;
#1505=CARTESIAN_POINT ( 'NONE',  ( 1.878215178124995832, -28.10312499938548569, 5.746835883940462963 ) ) ;
#1512=CARTESIAN_POINT ( 'NONE',  ( -1.878215178124998497, 29.49062499938548498, 12.25316411605951927 ) ) ;
#1515=CARTESIAN_POINT ( 'NONE',  ( 1.878215178125004048, 26.56562499938548427, 5.746835883940462963 ) ) ;
#1516=CARTESIAN_POINT ( 'NONE',  ( 4.000000000000003553, 25.00000000000000000, 8.999999999999992895 ) ) ;
#1517=CARTESIAN_POINT ( 'NONE',  ( 16.59933168835424411, 22.25618593784655630, 8.999999999999992895 ) ) ;
#1518=CARTESIAN_POINT ( 'NONE',  ( 21.04090992281141581, 18.38471254485196837, 12.25316411605952283 ) ) ;
#1520=CARTESIAN_POINT ( 'NONE',  ( -0.7500000000000001110, 9.184850993605150903E-17, 15.00000000000000178 ) ) ;
#1521=CARTESIAN_POINT ( 'NONE',  ( 23.52603154635960436, 18.61577656318150176, 6.996763648122161783 ) ) ;
#1522=CARTESIAN_POINT ( 'NONE',  ( 21.99777755166815751, 16.68538279574934435, 11.16877607737301403 ) ) ;
#1526=CARTESIAN_POINT ( 'NONE',  ( 3.999999999999996447, -26.57500000000000284, 8.999999999999992895 ) ) ;
#1530=CARTESIAN_POINT ( 'NONE',  ( 1.999999999999998224, -29.74374999877096926, 12.46410161513774639 ) ) ;
#1532=CARTESIAN_POINT ( 'NONE',  ( -3.756430356250003655, -27.84062499938548640, 8.999999999999992895 ) ) ;
#1534=PRODUCT_DEFINITION_SHAPE ( 'NONE', 'NONE',  #17976 ) ;
#1537=CARTESIAN_POINT ( 'NONE',  ( 19.74676196587764210, 22.58567065652198735, 12.46960170373642107 ) ) ;
#1550=CARTESIAN_POINT ( 'NONE',  ( 16.64794527869176122, 19.47637240343788179, 5.535898384862237620 ) ) ;
#1555=DIRECTION ( 'NONE',  ( 0.000000000000000000, -0.000000000000000000, 1.000000000000000000 ) ) ;
#1556=CARTESIAN_POINT ( 'NONE',  ( 3.834746474454188013E-15, 27.36250000000000426, 4.999999999999992006 ) ) ;
#1564=ORIENTED_EDGE ( 'NONE', *, *, #24964, .T. ) ;
#1574=CARTESIAN_POINT ( 'NONE',  ( 3.756430356250004099, 28.89062499938548356, 6.831223922626973533 ) ) ;
#1583=( BOUNDED_CURVE ( )  B_SPLINE_CURVE ( 2, ( #2616, #8892, #23007, #22623, #20520, #20913, #10828, #18822, #12408 ),
 .UNSPECIFIED., .F., .F. ) 
 B_SPLINE_CURVE_WITH_KNOTS ( ( 3, 2, 2, 2, 3 ),
 ( 0.8750000000000000000, 0.8833333333333333037, 0.9000000000000000222, 0.9166666666666666297, 0.9250000000000000444 ),
 .UNSPECIFIED. ) 
 CURVE ( )  GEOMETRIC_REPRESENTATION_ITEM ( )  RATIONAL_B_SPLINE_CURVE ( ( 0.9330127018922194093, 0.9330127018922194093, 1.000000000000000000, 0.8660254037844387076, 1.000000000000000000, 0.8660254037844387076, 1.000000000000000000, 0.9330127018922189652, 0.9330127018922194093 ) ) 
 REPRESENTATION_ITEM ( '' )  );
#1584=CARTESIAN_POINT ( 'NONE',  ( -4.000000000000003553, -26.33124999877097139, 6.690598923241489970 ) ) ;
#1585=CARTESIAN_POINT ( 'NONE',  ( 3.756430356250002323, 29.26562499938548356, 11.16877607737301226 ) ) ;
#1591=DIRECTION ( 'NONE',  ( 1.000000000000000000, 0.000000000000000000, -0.000000000000000000 ) ) ;
#1594=EDGE_LOOP ( 'NONE', ( #24309, #8224, #19587, #15571 ) ) ;
#1597=ORIENTED_EDGE ( 'NONE', *, *, #18674, .T. ) ;
#1598=CARTESIAN_POINT ( 'NONE',  ( -1.878215178125004048, -27.12812499938548783, 5.746835883940462963 ) ) ;
#1599=ORIENTED_EDGE ( 'NONE', *, *, #15919, .F. ) ;
#1600=ORIENTED_EDGE ( 'NONE', *, *, #24972, .T. ) ;
#1602=VERTEX_POINT ( 'NONE', #6000 ) ;
#1607=CARTESIAN_POINT ( 'NONE',  ( 19.60447174239884305, 22.26066912035814127, 12.25316411605951927 ) ) ;
#1610=CARTESIAN_POINT ( 'NONE',  ( -3.999999999999997335, 28.86250000000000071, 11.30940107675849404 ) ) ;
#1612=CARTESIAN_POINT ( 'NONE',  ( 23.08495422774248240, 17.77255947182365503, 6.831223922626973533 ) ) ;
#1614=VERTEX_POINT ( 'NONE', #16077 ) ;
#1619=CARTESIAN_POINT ( 'NONE',  ( -3.834746474454188013E-15, -27.81249999999999645, 4.999999999999992006 ) ) ;
#1620=AXIS2_PLACEMENT_3D ( 'NONE', #360, #1937, #4144 ) ;
#1623=ORIENTED_EDGE ( 'NONE', *, *, #8353, .F. ) ;
#1635=VECTOR ( 'NONE', #16499, 999.9999999999998863 ) ;
#1636=CARTESIAN_POINT ( 'NONE',  ( -3.756430356249996994, 28.96562499938548285, 8.999999999999992895 ) ) ;
#1637=ADVANCED_FACE ( 'NONE', ( #24301 ), #1015, .F. ) ;
#1638=LINE ( 'NONE', #17462, #24206 ) ;
#1641=CARTESIAN_POINT ( 'NONE',  ( -1.878215178124998497, 28.14062499938548356, 12.25316411605951927 ) ) ;
#1643=CARTESIAN_POINT ( 'NONE',  ( 3.878215178125003604, 29.82343749907822783, 8.999999999999992895 ) ) ;
#1644=CARTESIAN_POINT ( 'NONE',  ( 16.28113363682029657, 21.93798788631260877, 8.999999999999992895 ) ) ;
#1645=CARTESIAN_POINT ( 'NONE',  ( 22.13036007314063625, 16.81796531722181598, 6.831223922626973533 ) ) ;
#1648=CARTESIAN_POINT ( 'NONE',  ( 3.469446951953614189E-15, 30.00000000000000355, 8.999999999999992895 ) ) ;
#1649=CARTESIAN_POINT ( 'NONE',  ( 23.60239120520362022, 18.51856749399161473, 7.226316032987424975 ) ) ;
#1653=EDGE_LOOP ( 'NONE', ( #16304, #8249, #22495, #7437 ) ) ;
#1655=CARTESIAN_POINT ( 'NONE',  ( -3.752267015613588906E-15, -25.56250000000000000, 4.381197846482986158 ) ) ;
#1657=VERTEX_POINT ( 'NONE', #16220 ) ;
#1661=DIRECTION ( 'NONE',  ( 0.000000000000000000, -1.000000000000000000, 0.000000000000000000 ) ) ;
#1680=CARTESIAN_POINT ( 'NONE',  ( 20.75150184982686596, 15.43910709390805280, 8.999999999999992895 ) ) ;
#1685=CARTESIAN_POINT ( 'NONE',  ( 3.756430356249996994, -29.52812499938548640, 8.999999999999992895 ) ) ;
#1690=DIRECTION ( 'NONE',  ( 0.000000000000000000, 1.000000000000000000, 0.000000000000000000 ) ) ;
#1707=CLOSED_SHELL ( 'NONE', ( #20653, #11784, #20616, #2004, #13663, #21351, #1930, #21195, #2430, #23617, #4209, #4037, #21887, #11701, #10287, #9179, #24063, #13901, #21749, #1210, #17984, #25388, #6940, #22389, #10182, #2011, #24637, #20740, #8165, #15835, #14762, #17627, #23412, #16719, #4571, #6059, #1064, #3906, #4390, #16275, #15401, #13456, #9685, #11222, #5105, #18015, #16983, #19187, #13692, #1977, #5001, #19635, #17079, #20177, #1150, #5131, #3102, #676, #7145, #24903, #14109, #598, #13778, #20832, #14216, #713, #16143, #20555, #11466, #65, #12736, #9369, #6134, #426, #9609, #2958, #3530, #10783, #16931, #18200, #24170, #24494, #8665, #3823, #18770, #25765, #8141, #12180, #7903, #12881, #22087, #1905, #15163, #8674, #4136, #11422, #9408, #7262, #7190, #1637, #14444, #2194, #25555, #20558, #6885, #5485, #9859, #19759, #18095, #19399, #3559, #16200, #11747, #22253, #20841, #17559, #21319 ) ) ;
#1708=CARTESIAN_POINT ( 'NONE',  ( 23.80283954968513171, 18.26064280072889190, 9.928636277907715524 ) ) ;
#1712=FILL_AREA_STYLE_COLOUR ( '', #7654 ) ;
#1713=CARTESIAN_POINT ( 'NONE',  ( -1.878215178124998497, 29.15312499938548640, 12.25316411605951927 ) ) ;
#1721=CARTESIAN_POINT ( 'NONE',  ( -2.000000000000000888, -25.76874999877096784, 12.46410161513774817 ) ) ;
#1723=CARTESIAN_POINT ( 'NONE',  ( 1.878215178125000939, 27.42812499938548498, 12.25316411605952283 ) ) ;
#1726=CARTESIAN_POINT ( 'NONE',  ( 21.21320343559646915, 21.21320343559638744, 8.999999999999992895 ) ) ;
#1728=CARTESIAN_POINT ( 'NONE',  ( 3.834746474454188013E-15, 26.40624999877096357, 4.999999999999992006 ) ) ;
#1730=CARTESIAN_POINT ( 'NONE',  ( -2.000000000000003997, -29.12500000000000000, 5.535898384862238508 ) ) ;
#1731=ORIENTED_EDGE ( 'NONE', *, *, #9338, .T. ) ;
#1736=CARTESIAN_POINT ( 'NONE',  ( 3.756430356249996994, -27.72812499938548569, 8.999999999999992895 ) ) ;
#1738=ORIENTED_EDGE ( 'NONE', *, *, #1394, .F. ) ;
#1739=CARTESIAN_POINT ( 'NONE',  ( -3.999999999999996447, 28.82499999999999929, 8.999999999999992895 ) ) ;
#1740=EDGE_CURVE ( 'NONE', #19049, #20151, #10315, .T. ) ;
#1748=DIRECTION ( 'NONE',  ( 0.000000000000000000, 0.000000000000000000, -1.000000000000000000 ) ) ;
#1749=CARTESIAN_POINT ( 'NONE',  ( 21.14697593998939595, 18.49077856202994852, 5.746835883940462963 ) ) ;
#1754=CARTESIAN_POINT ( 'NONE',  ( -1.999999999999995781, 28.75000000000000000, 5.535898384862237620 ) ) ;
#1755=( BOUNDED_SURFACE ( )  B_SPLINE_SURFACE ( 1, 2, ( 
 ( #22911, #15204, #2653, #1193, #9174, #25135, #10614, #9695, #23676, #25264, #1721, #3664, #17416, #19369, #7464, #5253, #9553, #25767, #1338, #21336, #23423, #21471, #7344, #13619, #21717, #1584, #17542, #3801, #9312, #21202, #3418, #17679, #19488, #23558, #25648, #13231, #11395, #17297, #15321, #11518, #25515, #1463, #5639, #5510, #9435, #13500, #7728, #15713, #19235, #7603, #5753, #13740, #15588, #25379, #3545, #15454, #21584, #11642, #19617, #23289, #7847, #11781, #19758, #3280, #11253, #9816, #1855, #17801, #23172, #5374, #13364, #10449, #6409, #24330, #22095, #8243, #8123, #22357, #23805, #14399, #14270, #10068, #17922, #16362, #4441, #12414, #21852, #2101, #20381, #20261, #10314, #19998, #18444, #18069, #2479, #4051, #152, #15832, #23941, #22236, #2238, #275, #2358, #21976, #540, #12020, #3934, #4319, #14005, #5893, #13878, #7988, #16098, #13, #9937, #18308, #11903, #19871, #4184, #15977, #1971 ),
 ( #24062, #12160, #6024, #14129, #6145, #24189, #20136, #10195, #6279, #18191, #12294, #16219, #401, #8370, #4568, #18691, #6532, #17001, #20785, #20527, #22630, #4718, #11101, #12690, #6660, #6924, #2621, #24571, #15036, #24454, #12549, #8754, #23016, #14648, #10582, #16883, #20662, #14784, #24848, #7049, #12813, #2866, #5100, #18577, #14515, #2743, #12942, #4837, #8901, #20922, #16492, #661, #8630, #16608, #13080, #3006, #14909, #21055, #10705, #3134, #16744, #22759, #19078, #6802, #8512, #22879, #779, #24713, #4961, #10835, #10977, #18830, #22486, #919, #18960, #1046, #9018, #24966, #13469, #13202, #15291, #23258, #3766, #5344, #25234, #25481, #21173, #17267, #7698, #17129, #5223, #1433, #15679, #7314, #23144, #9521, #13326, #7431, #19202, #25101, #5724, #3245, #13705, #1298, #7187, #25349, #15175, #11219, #9280, #21436, #21681, #21302, #11360, #25614, #1685, #11744, #3382, #1159, #17503, #11488, #21555 ) ),
 .UNSPECIFIED., .F., .F., .F. ) 
 B_SPLINE_SURFACE_WITH_KNOTS ( ( 2, 2 ),
 ( 3, 2, 2, 2, 2, 2, 2, 2, 2, 2, 2, 2, 2, 2, 2, 2, 2, 2, 2, 2, 2, 2, 2, 2, 2, 2, 2, 2, 2, 2, 2, 2, 2, 2, 2, 2, 2, 2, 2, 2, 2, 2, 2, 2, 2, 2, 2, 2, 2, 2, 2, 2, 2, 2, 2, 2, 2, 2, 2, 2, 3 ),
 ( 0.000000000000000000, 1.000000000000000000 ),
 ( 0.000000000000000000, 0.01666666666666666644, 0.03333333333333333287, 0.05000000000000000278, 0.06666666666666666574, 0.08333333333333332871, 0.1000000000000000056, 0.1166666666666666685, 0.1333333333333333315, 0.1499999999999999944, 0.1666666666666666574, 0.1833333333333333204, 0.2000000000000000111, 0.2166666666666666741, 0.2333333333333333370, 0.2500000000000000000, 0.2666666666666666630, 0.2833333333333333259, 0.2999999999999999889, 0.3166666666666666519, 0.3333333333333333148, 0.3499999999999999778, 0.3666666666666666408, 0.3833333333333333592, 0.4000000000000000222, 0.4166666666666666852, 0.4333333333333333481, 0.4500000000000000111, 0.4666666666666666741, 0.4833333333333333370, 0.5000000000000000000, 0.5166666666666667185, 0.5333333333333333259, 0.5500000000000000444, 0.5666666666666666519, 0.5833333333333333703, 0.5999999999999999778, 0.6166666666666666963, 0.6333333333333333037, 0.6500000000000000222, 0.6666666666666666297, 0.6833333333333333481, 0.6999999999999999556, 0.7166666666666666741, 0.7333333333333332815, 0.7500000000000000000, 0.7666666666666667185, 0.7833333333333333259, 0.8000000000000000444, 0.8166666666666666519, 0.8333333333333333703, 0.8499999999999999778, 0.8666666666666666963, 0.8833333333333333037, 0.9000000000000000222, 0.9166666666666666297, 0.9333333333333333481, 0.9499999999999999556, 0.9666666666666666741, 0.9833333333333332815, 1.000000000000000000 ),
 .UNSPECIFIED. ) 
 GEOMETRIC_REPRESENTATION_ITEM ( )  RATIONAL_B_SPLINE_SURFACE ( (
 ( 1.000000000000000000, 0.8660254037844387076, 1.000000000000000000, 0.8660254037844387076, 1.000000000000000000, 0.8660254037844387076, 1.000000000000000000, 0.8660254037844387076, 1.000000000000000000, 0.8660254037844387076, 1.000000000000000000, 0.8660254037844387076, 1.000000000000000000, 0.8660254037844387076, 1.000000000000000000, 0.8660254037844387076, 1.000000000000000000, 0.8660254037844387076, 1.000000000000000000, 0.8660254037844387076, 1.000000000000000000, 0.8660254037844387076, 1.000000000000000000, 0.8660254037844387076, 1.000000000000000000, 0.8660254037844387076, 1.000000000000000000, 0.8660254037844387076, 1.000000000000000000, 0.8660254037844387076, 1.000000000000000000, 0.8660254037844387076, 1.000000000000000000, 0.8660254037844387076, 1.000000000000000000, 0.8660254037844387076, 1.000000000000000000, 0.8660254037844387076, 1.000000000000000000, 0.8660254037844387076, 1.000000000000000000, 0.8660254037844387076, 1.000000000000000000, 0.8660254037844387076, 1.000000000000000000, 0.8660254037844387076, 1.000000000000000000, 0.8660254037844387076, 1.000000000000000000, 0.8660254037844387076, 1.000000000000000000, 0.8660254037844387076, 1.000000000000000000, 0.8660254037844387076, 1.000000000000000000, 0.8660254037844387076, 1.000000000000000000, 0.8660254037844387076, 1.000000000000000000, 0.8660254037844387076, 1.000000000000000000, 0.8660254037844387076, 1.000000000000000000, 0.8660254037844387076, 1.000000000000000000, 0.8660254037844387076, 1.000000000000000000, 0.8660254037844387076, 1.000000000000000000, 0.8660254037844387076, 1.000000000000000000, 0.8660254037844387076, 1.000000000000000000, 0.8660254037844387076, 1.000000000000000000, 0.8660254037844387076, 1.000000000000000000, 0.8660254037844387076, 1.000000000000000000, 0.8660254037844387076, 1.000000000000000000, 0.8660254037844387076, 1.000000000000000000, 0.8660254037844387076, 1.000000000000000000, 0.8660254037844387076, 1.000000000000000000, 0.8660254037844387076, 1.000000000000000000, 0.8660254037844387076, 1.000000000000000000, 0.8660254037844387076, 1.000000000000000000, 0.8660254037844387076, 1.000000000000000000, 0.8660254037844387076, 1.000000000000000000, 0.8660254037844387076, 1.000000000000000000, 0.8660254037844387076, 1.000000000000000000, 0.8660254037844387076, 1.000000000000000000, 0.8660254037844387076, 1.000000000000000000, 0.8660254037844387076, 1.000000000000000000, 0.8660254037844387076, 1.000000000000000000, 0.8660254037844387076, 1.000000000000000000, 0.8660254037844387076, 1.000000000000000000, 0.8660254037844387076, 1.000000000000000000, 0.8660254037844387076, 1.000000000000000000, 0.8660254037844387076, 1.000000000000000000, 0.8660254037844387076, 1.000000000000000000),
 ( 1.000000000000000000, 0.8660254037844387076, 1.000000000000000000, 0.8660254037844387076, 1.000000000000000000, 0.8660254037844387076, 1.000000000000000000, 0.8660254037844387076, 1.000000000000000000, 0.8660254037844387076, 1.000000000000000000, 0.8660254037844387076, 1.000000000000000000, 0.8660254037844387076, 1.000000000000000000, 0.8660254037844387076, 1.000000000000000000, 0.8660254037844387076, 1.000000000000000000, 0.8660254037844387076, 1.000000000000000000, 0.8660254037844387076, 1.000000000000000000, 0.8660254037844387076, 1.000000000000000000, 0.8660254037844387076, 1.000000000000000000, 0.8660254037844387076, 1.000000000000000000, 0.8660254037844387076, 1.000000000000000000, 0.8660254037844387076, 1.000000000000000000, 0.8660254037844387076, 1.000000000000000000, 0.8660254037844387076, 1.000000000000000000, 0.8660254037844387076, 1.000000000000000000, 0.8660254037844387076, 1.000000000000000000, 0.8660254037844387076, 1.000000000000000000, 0.8660254037844387076, 1.000000000000000000, 0.8660254037844387076, 1.000000000000000000, 0.8660254037844387076, 1.000000000000000000, 0.8660254037844387076, 1.000000000000000000, 0.8660254037844387076, 1.000000000000000000, 0.8660254037844387076, 1.000000000000000000, 0.8660254037844387076, 1.000000000000000000, 0.8660254037844387076, 1.000000000000000000, 0.8660254037844387076, 1.000000000000000000, 0.8660254037844387076, 1.000000000000000000, 0.8660254037844387076, 1.000000000000000000, 0.8660254037844387076, 1.000000000000000000, 0.8660254037844387076, 1.000000000000000000, 0.8660254037844387076, 1.000000000000000000, 0.8660254037844387076, 1.000000000000000000, 0.8660254037844387076, 1.000000000000000000, 0.8660254037844387076, 1.000000000000000000, 0.8660254037844387076, 1.000000000000000000, 0.8660254037844387076, 1.000000000000000000, 0.8660254037844387076, 1.000000000000000000, 0.8660254037844387076, 1.000000000000000000, 0.8660254037844387076, 1.000000000000000000, 0.8660254037844387076, 1.000000000000000000, 0.8660254037844387076, 1.000000000000000000, 0.8660254037844387076, 1.000000000000000000, 0.8660254037844387076, 1.000000000000000000, 0.8660254037844387076, 1.000000000000000000, 0.8660254037844387076, 1.000000000000000000, 0.8660254037844387076, 1.000000000000000000, 0.8660254037844387076, 1.000000000000000000, 0.8660254037844387076, 1.000000000000000000, 0.8660254037844387076, 1.000000000000000000, 0.8660254037844387076, 1.000000000000000000, 0.8660254037844387076, 1.000000000000000000, 0.8660254037844387076, 1.000000000000000000, 0.8660254037844387076, 1.000000000000000000, 0.8660254037844387076, 1.000000000000000000, 0.8660254037844387076, 1.000000000000000000, 0.8660254037844387076, 1.000000000000000000) ) ) 
 REPRESENTATION_ITEM ( '' )  SURFACE ( )  );
#1757=CARTESIAN_POINT ( 'NONE',  ( 18.22334004483017011, 23.53573480074883761, 8.999999999999992895 ) ) ;
#1758=CARTESIAN_POINT ( 'NONE',  ( 1.057460391440397258E-14, -29.55624999877096926, 4.999999999999992006 ) ) ;
#1764=VECTOR ( 'NONE', #1067, 1000.000000000000000 ) ;
#1768=CARTESIAN_POINT ( 'NONE',  ( 16.36952198446861217, 19.19794910921473630, 5.535898384862237620 ) ) ;
#1769=ORIENTED_EDGE ( 'NONE', *, *, #24964, .F. ) ;
#1771=VECTOR ( 'NONE', #22592, 1000.000000000000000 ) ;
#1785=CARTESIAN_POINT ( 'NONE',  ( 15.98945208958084230, 21.64630633907315982, 11.30940107675849404 ) ) ;
#1786=CARTESIAN_POINT ( 'NONE',  ( 20.79998790990604718, 20.79998790990596902, 4.662447845253954171 ) ) ;
#1794=CARTESIAN_POINT ( 'NONE',  ( 3.999999999999996447, -27.02500000000000213, 8.999999999999992895 ) ) ;
#1799=CARTESIAN_POINT ( 'NONE',  ( 3.959305671612554781E-15, 30.00000000000000355, 12.99999999999999289 ) ) ;
#1800=CARTESIAN_POINT ( 'NONE',  ( 11.52193136556786257, 23.36965697125208052, 20.00001200000000168 ) ) ;
#1801=CARTESIAN_POINT ( 'NONE',  ( 4.000000000000003553, 26.33124999877097139, 6.690598923241489970 ) ) ;
#1804=EDGE_CURVE ( 'NONE', #17932, #25409, #2835, .T. ) ;
#1811=CARTESIAN_POINT ( 'NONE',  ( -1.057460391440397258E-14, 29.10624999877096641, 4.999999999999992006 ) ) ;
#1815=LINE ( 'NONE', #22055, #16365 ) ;
#1817=CARTESIAN_POINT ( 'NONE',  ( -3.999999999999995559, 26.93124999877096926, 6.690598923241487306 ) ) ;
#1818=CARTESIAN_POINT ( 'NONE',  ( 18.01575495898401513, 18.01575495898394408, 13.33755215474602984 ) ) ;
#1819=CARTESIAN_POINT ( 'NONE',  ( 16.21484237521500305, 21.87169662470731524, 6.690598923241487306 ) ) ;
#1821=CARTESIAN_POINT ( 'NONE',  ( -1.859271017917182139E-15, -29.78124999877096712, 12.99999999999999289 ) ) ;
#1847=( LENGTH_UNIT ( ) NAMED_UNIT ( * ) SI_UNIT ( .MILLI., .METRE. ) );
#1848=CARTESIAN_POINT ( 'NONE',  ( 3.756430356250003655, 28.40312499938548640, 8.999999999999992895 ) ) ;
#1849=CARTESIAN_POINT ( 'NONE',  ( -1.057460391440397258E-14, 28.71250000000000213, 4.999999999999992006 ) ) ;
#1855=CARTESIAN_POINT ( 'NONE',  ( 3.999999999999996447, -27.86874999877096570, 8.999999999999992895 ) ) ;
#1856=CARTESIAN_POINT ( 'NONE',  ( 2.672651547586948120E-15, 26.94062499938548783, 13.33755215474602984 ) ) ;
#1859=CARTESIAN_POINT ( 'NONE',  ( 1.999999999999998224, -26.14374999877096784, 12.46410161513774639 ) ) ;
#1863=ORIENTED_EDGE ( 'NONE', *, *, #5533, .F. ) ;
#1867=CARTESIAN_POINT ( 'NONE',  ( -3.756430356250003655, -27.95312499938548711, 8.999999999999992895 ) ) ;
#1877=CARTESIAN_POINT ( 'NONE',  ( 23.05843772344798381, 17.74604296752915999, 8.999999999999992895 ) ) ;
#1881=CARTESIAN_POINT ( 'NONE',  ( 3.752267015613588906E-15, 29.16250000000000142, 4.381197846482986158 ) ) ;
#1883=CARTESIAN_POINT ( 'NONE',  ( 20.48178985837210320, 20.48178985837202504, 4.662447845253954171 ) ) ;
#1885=ORIENTED_EDGE ( 'NONE', *, *, #23874, .T. ) ;
#1888=ORIENTED_EDGE ( 'NONE', *, *, #24958, .F. ) ;
#1890=CARTESIAN_POINT ( 'NONE',  ( -3.756430356249996994, 26.82812499938548711, 8.999999999999992895 ) ) ;
#1900=CYLINDRICAL_SURFACE ( 'NONE', #11777, 4.000000000000000000 ) ;
#1905=ADVANCED_FACE ( 'NONE', ( #13943 ), #13433, .F. ) ;
#1906=CARTESIAN_POINT ( 'NONE',  ( 1.878215178125000939, 25.96562499938548285, 12.25316411605952283 ) ) ;
#1910=DIRECTION ( 'NONE',  ( 0.8660254037844397068, 0.4999999999999983347, 0.000000000000000000 ) ) ;
#1911=CARTESIAN_POINT ( 'NONE',  ( 21.75237235625120036, 16.09551810675874961, 11.30940107675849760 ) ) ;
#1912=CARTESIAN_POINT ( 'NONE',  ( 17.93165849759071762, 23.24405325350938867, 11.16877607737301226 ) ) ;
#1913=CARTESIAN_POINT ( 'NONE',  ( -1.071796769724498999, -28.45134618820330275, 12.99999999999998757 ) ) ;
#1914=CARTESIAN_POINT ( 'NONE',  ( -1.878215178125004048, -26.11562499938548498, 5.746835883940462963 ) ) ;
#1915=CARTESIAN_POINT ( 'NONE',  ( 23.58876780933789519, 18.27637305341907492, 11.16877607737301403 ) ) ;
#1917=EDGE_LOOP ( 'NONE', ( #11967, #217, #10984, #17041 ) ) ;
#1919=CARTESIAN_POINT ( 'NONE',  ( 1.999999999999998224, -26.64999999999999858, 12.46410161513774639 ) ) ;
#1923=CARTESIAN_POINT ( 'NONE',  ( -1.859271017917182139E-15, -29.78124999877096712, 12.99999999999999289 ) ) ;
#1924=CARTESIAN_POINT ( 'NONE',  ( 15.85973458909325728, 20.67279826512042362, 20.00001200000000168 ) ) ;
#1925=CARTESIAN_POINT ( 'NONE',  ( 4.000000000000001776, 26.25624999877096855, 11.30940107675849760 ) ) ;
#1926=VERTEX_POINT ( 'NONE', #1520 ) ;
#1927=VERTEX_POINT ( 'NONE', #21404 ) ;
#1930=ADVANCED_FACE ( 'NONE', ( #3868 ), #25442, .F. ) ;
#1931=PLANE ( 'NONE',  #2503 ) ;
#1933=EDGE_CURVE ( 'NONE', #14528, #5581, #19396, .T. ) ;
#1934=CARTESIAN_POINT ( 'NONE',  ( 19.83756213693951764, 21.35331166479149090, 4.999999999999995559 ) ) ;
#1935=CARTESIAN_POINT ( 'NONE',  ( 19.96119519019960720, 18.44544566234749183, 12.99999999999999112 ) ) ;
#1937=DIRECTION ( 'NONE',  ( 0.000000000000000000, 1.000000000000000000, 0.000000000000000000 ) ) ;
#1938=CARTESIAN_POINT ( 'NONE',  ( 15.62472262396960154, 20.93711737988828503, 11.16877607737301226 ) ) ;
#1945=DIRECTION ( 'NONE',  ( 0.000000000000000000, 0.000000000000000000, -1.000000000000000000 ) ) ;
#1948=CARTESIAN_POINT ( 'NONE',  ( 1.859271017917182139E-15, 27.08124999877096784, 12.99999999999999289 ) ) ;
#1952=ORIENTED_EDGE ( 'NONE', *, *, #14569, .F. ) ;
#1953=ORIENTED_EDGE ( 'NONE', *, *, #17459, .F. ) ;
#1956=CARTESIAN_POINT ( 'NONE',  ( -4.000000000000003553, -28.09374999877097068, 8.999999999999992895 ) ) ;
#1963=CARTESIAN_POINT ( 'NONE',  ( 3.756430356250003655, 27.95312499938548711, 8.999999999999992895 ) ) ;
#1965=CARTESIAN_POINT ( 'NONE',  ( 19.66640735175089105, 19.66640735175081289, 4.999999999999992006 ) ) ;
#1966=DIRECTION ( 'NONE',  ( 0.000000000000000000, -1.000000000000000000, 0.000000000000000000 ) ) ;
#1970=EDGE_CURVE ( 'NONE', #13143, #2042, #5277, .T. ) ;
#1971=CARTESIAN_POINT ( 'NONE',  ( -4.000000000000003553, -29.89374999877096784, 8.999999999999992895 ) ) ;
#1972=CARTESIAN_POINT ( 'NONE',  ( 3.735045420075836212E-15, 27.16562499938548569, 4.662447845253954171 ) ) ;
#1973=CARTESIAN_POINT ( 'NONE',  ( 1.071796769724487230, -26.03259618943233278, 4.999999999999992006 ) ) ;
#1974=DIRECTION ( 'NONE',  ( -0.7071067811865487940, -0.7071067811865463515, 0.000000000000000000 ) ) ;
#1976=ORIENTED_EDGE ( 'NONE', *, *, #13413, .F. ) ;
#1977=ADVANCED_FACE ( 'NONE', ( #4376 ), #4639, .F. ) ;
#1979=CARTESIAN_POINT ( 'NONE',  ( 1.626862140677534194E-14, 28.03750000000000497, 12.99999999999999289 ) ) ;
#1980=EDGE_LOOP ( 'NONE', ( #9772, #7853, #12703, #18590 ) ) ;
#1984=CARTESIAN_POINT ( 'NONE',  ( -1.878215178125000939, -25.96562499938548285, 12.25316411605952283 ) ) ;
#1985=EDGE_LOOP ( 'NONE', ( #611, #6697, #5907, #16169 ) ) ;
#1989=CARTESIAN_POINT ( 'NONE',  ( 3.735045420075836212E-15, 27.16562499938547859, 4.662447845253954171 ) ) ;
#1991=DIRECTION ( 'NONE',  ( 0.000000000000000000, 0.000000000000000000, -1.000000000000000000 ) ) ;
#1992=CARTESIAN_POINT ( 'NONE',  ( 19.44764619088677549, 19.44764619088670088, 4.662447845253954171 ) ) ;
#1996=CARTESIAN_POINT ( 'NONE',  ( -3.999999999999996003, 26.98750000000000426, 6.690598923241487306 ) ) ;
#2001=EDGE_CURVE ( 'NONE', #23534, #2876, #6355, .T. ) ;
#2004=ADVANCED_FACE ( 'NONE', ( #12092 ), #24395, .F. ) ;
#2007=CARTESIAN_POINT ( 'NONE',  ( -3.999999999999996447, 29.66874999877096997, 8.999999999999992895 ) ) ;
#2011=ADVANCED_FACE ( 'NONE', ( #20068 ), #2296, .F. ) ;
#2013=CIRCLE ( 'NONE', #11178, 8.000000000000000000 ) ;
#2023=CARTESIAN_POINT ( 'NONE',  ( -3.756430356249997882, 26.75312499938548427, 11.16877607737301226 ) ) ;
#2028=LINE ( 'NONE', #15763, #18740 ) ;
#2029=CARTESIAN_POINT ( 'NONE',  ( 19.82550637751786482, 19.82550637751779377, 13.61880215351699874 ) ) ;
#2032=CARTESIAN_POINT ( 'NONE',  ( 1.999999999999995781, -27.79374999877096997, 5.535898384862237620 ) ) ;
#2034=CARTESIAN_POINT ( 'NONE',  ( 3.756430356249997438, -25.85312499938548569, 11.16877607737301048 ) ) ;
#2035=EDGE_CURVE ( 'NONE', #14487, #10748, #9232, .T. ) ;
#2036=CARTESIAN_POINT ( 'NONE',  ( 20.56133937125558830, 20.56133937125551370, 13.33755215474603162 ) ) ;
#2040=CARTESIAN_POINT ( 'NONE',  ( -4.000000000000003553, -27.73750000000000071, 6.690598923241489970 ) ) ;
#2042=VERTEX_POINT ( 'NONE', #10371 ) ;
#2044=LINE ( 'NONE', #1799, #1322 ) ;
#2052=EDGE_CURVE ( 'NONE', #22340, #17898, #23384, .T. ) ;
#2064=CARTESIAN_POINT ( 'NONE',  ( 17.48763458135079318, 23.14448883084309472, 6.690598923241487306 ) ) ;
#2065=ORIENTED_EDGE ( 'NONE', *, *, #10383, .F. ) ;
#2071=CARTESIAN_POINT ( 'NONE',  ( 3.834746474454188013E-15, 26.40624999877096357, 4.999999999999992006 ) ) ;
#2072=CARTESIAN_POINT ( 'NONE',  ( 2.000000000000000888, 28.91874999877096997, 12.46410161513774817 ) ) ;
#2074=CARTESIAN_POINT ( 'NONE',  ( 1.071796769724491227, 27.28615380933863577, 4.999999999999989342 ) ) ;
#2075=CARTESIAN_POINT ( 'NONE',  ( -3.999999999999997335, 26.10624999877096997, 11.30940107675849404 ) ) ;
#2089=EDGE_CURVE ( 'NONE', #25409, #23573, #13729, .T. ) ;
#2094=CARTESIAN_POINT ( 'NONE',  ( -3.756430356249996994, 25.36562499938548498, 8.999999999999992895 ) ) ;
#2095=CARTESIAN_POINT ( 'NONE',  ( 18.27871029367229383, 21.10713741841841085, 5.535898384862237620 ) ) ;
#2099=DIRECTION ( 'NONE',  ( 0.000000000000000000, 0.000000000000000000, 1.000000000000000000 ) ) ;
#2101=CARTESIAN_POINT ( 'NONE',  ( -3.752267015613588906E-15, -28.65624999877096712, 4.381197846482986158 ) ) ;
#2102=CARTESIAN_POINT ( 'NONE',  ( 3.756430356250004099, 27.54062499938548569, 6.831223922626973533 ) ) ;
#2105=CARTESIAN_POINT ( 'NONE',  ( -1.999999999999998224, 29.74374999877096926, 12.46410161513774639 ) ) ;
#2107=EDGE_LOOP ( 'NONE', ( #7495, #22644, #3467, #8386 ) ) ;
#2108=CARTESIAN_POINT ( 'NONE',  ( -1.878215178125004048, -28.81562499938548427, 5.746835883940462963 ) ) ;
#2116=VERTEX_POINT ( 'NONE', #5258 ) ;
#2124=CARTESIAN_POINT ( 'NONE',  ( 3.756430356250002323, 26.11562499938548498, 11.16877607737301403 ) ) ;
#2127=CARTESIAN_POINT ( 'NONE',  ( 16.55280027427694378, 21.86519503019561839, 8.999999999999992895 ) ) ;
#2135=CARTESIAN_POINT ( 'NONE',  ( -3.999999999999997335, 28.41249999999999787, 11.30940107675849404 ) ) ;
#2137=CARTESIAN_POINT ( 'NONE',  ( 3.756430356250003655, 28.29062499938548569, 8.999999999999992895 ) ) ;
#2139=CARTESIAN_POINT ( 'NONE',  ( 17.87862548900172399, 23.19102024492039504, 6.831223922626973533 ) ) ;
#2141=ORIENTED_EDGE ( 'NONE', *, *, #7653, .F. ) ;
#2147=CARTESIAN_POINT ( 'NONE',  ( 2.620986760973688460E-15, 29.33124999877096784, 13.61880215351699874 ) ) ;
#2149=CARTESIAN_POINT ( 'NONE',  ( 3.834746474454188013E-15, 26.01249999999999574, 4.999999999999992006 ) ) ;
#2152=CARTESIAN_POINT ( 'NONE',  ( -3.469446951953614189E-15, -30.00000000000000355, 8.999999999999992895 ) ) ;
#2158=DIRECTION ( 'NONE',  ( -0.7071067811865487940, -0.7071067811865463515, 0.000000000000000000 ) ) ;
#2163=CARTESIAN_POINT ( 'NONE',  ( -3.756430356249997882, 26.30312499938548498, 11.16877607737301226 ) ) ;
#2164=CIRCLE ( 'NONE', #24280, 8.000000000000000000 ) ;
#2168=CARTESIAN_POINT ( 'NONE',  ( 23.05168106668148553, 17.39482681718902768, 8.999999999999992895 ) ) ;
#2177=CARTESIAN_POINT ( 'NONE',  ( -2.000000000000003997, -28.67500000000000426, 5.535898384862238508 ) ) ;
#2188=CARTESIAN_POINT ( 'NONE',  ( 20.69613160098474580, 17.86770447623847957, 5.535898384862238508 ) ) ;
#2194=ADVANCED_FACE ( 'NONE', ( #2802 ), #19494, .T. ) ;
#2197=DIRECTION ( 'NONE',  ( 0.000000000000000000, 0.000000000000000000, -1.000000000000000000 ) ) ;
#2200=CARTESIAN_POINT ( 'NONE',  ( 19.46311415215975771, 16.63468702741349858, 5.535898384862238508 ) ) ;
#2202=CARTESIAN_POINT ( 'NONE',  ( 17.85665593321704137, 17.85665593321697742, 4.662447845253954171 ) ) ;
#2203=CARTESIAN_POINT ( 'NONE',  ( 19.46753356867311524, 19.46753356867304774, 13.61880215351699874 ) ) ;
#2210=CARTESIAN_POINT ( 'NONE',  ( 3.469446951953614189E-15, 30.00000000000000355, 4.999999999999992006 ) ) ;
#2212=CARTESIAN_POINT ( 'NONE',  ( 23.83066714524420249, 18.34604264253855987, 8.999999999999992895 ) ) ;
#2215=CARTESIAN_POINT ( 'NONE',  ( 3.752267015613588906E-15, 26.40624999877097068, 4.381197846482986158 ) ) ;
#2216=CARTESIAN_POINT ( 'NONE',  ( -2.672651547586948120E-15, -26.37812499938548427, 13.33755215474602984 ) ) ;
#2217=DIRECTION ( 'NONE',  ( -1.000000000000000000, 0.000000000000000000, 0.000000000000000000 ) ) ;
#2218=ORIENTED_EDGE ( 'NONE', *, *, #14683, .F. ) ;
#2229=CARTESIAN_POINT ( 'NONE',  ( -3.756430356249995661, 25.32812499938548356, 6.831223922626973533 ) ) ;
#2237=CARTESIAN_POINT ( 'NONE',  ( 18.07541709408115693, 18.07541709408108588, 4.999999999999992006 ) ) ;
#2238=CARTESIAN_POINT ( 'NONE',  ( 1.999999999999995781, -29.14374999877096784, 5.535898384862237620 ) ) ;
#2242=DIRECTION ( 'NONE',  ( 0.000000000000000000, 0.000000000000000000, 1.000000000000000000 ) ) ;
#2243=CARTESIAN_POINT ( 'NONE',  ( 3.595210675795415867, -29.78396494222454294, 7.227341970420264161 ) ) ;
#2252=CARTESIAN_POINT ( 'NONE',  ( 19.98460540328483859, 19.98460540328476398, 4.999999999999992006 ) ) ;
#2256=CARTESIAN_POINT ( 'NONE',  ( 3.756430356250003655, 25.25312499938548427, 8.999999999999992895 ) ) ;
#2260=CARTESIAN_POINT ( 'NONE',  ( 17.21571288163933389, 22.52810763755800849, 11.16877607737301226 ) ) ;
#2266=CARTESIAN_POINT ( 'NONE',  ( 1.878215178125000939, 28.66562499938548569, 12.25316411605952283 ) ) ;
#2269=CARTESIAN_POINT ( 'NONE',  ( 15.31328122920215229, 20.97013547869446626, 11.30940107675849404 ) ) ;
#2277=CARTESIAN_POINT ( 'NONE',  ( -1.071796769724485454, 27.51115380933863719, 12.99999999999999467 ) ) ;
#2281=ORIENTED_EDGE ( 'NONE', *, *, #6066, .F. ) ;
#2284=( BOUNDED_CURVE ( )  B_SPLINE_CURVE ( 2, ( #17493, #3372, #7421, #11350, #7306, #9395, #23514, #13578, #7178 ),
 .UNSPECIFIED., .F., .T. ) 
 B_SPLINE_CURVE_WITH_KNOTS ( ( 3, 2, 2, 2, 3 ),
 ( 0.4250000000000000444, 0.4333333333333333481, 0.4500000000000000111, 0.4666666666666666741, 0.4750000000000000333 ),
 .UNSPECIFIED. ) 
 CURVE ( )  GEOMETRIC_REPRESENTATION_ITEM ( )  RATIONAL_B_SPLINE_CURVE ( ( 0.9330127018922194093, 0.9330127018922196314, 1.000000000000000000, 0.8660254037844387076, 1.000000000000000000, 0.8660254037844387076, 1.000000000000000000, 0.9330127018922191873, 0.9330127018922194093 ) ) 
 REPRESENTATION_ITEM ( '' )  );
#2285=CARTESIAN_POINT ( 'NONE',  ( -1.057460391440397258E-14, 29.16249999999999787, 4.999999999999992006 ) ) ;
#2288=EDGE_CURVE ( 'NONE', #20963, #7544, #18242, .T. ) ;
#2292=CARTESIAN_POINT ( 'NONE',  ( 23.39639562250992810, 17.73954137301747380, 6.690598923241489970 ) ) ;
#2296=CYLINDRICAL_SURFACE ( 'NONE', #5713, 4.000000000000000000 ) ;
#2297=CARTESIAN_POINT ( 'NONE',  ( -1.878215178125004048, -25.21562499938548285, 5.746835883940462963 ) ) ;
#2298=DIRECTION ( 'NONE',  ( 0.000000000000000000, 0.000000000000000000, -1.000000000000000000 ) ) ;
#2301=CARTESIAN_POINT ( 'NONE',  ( -4.000000000000001776, -28.11250000000000426, 11.30940107675849760 ) ) ;
#2304=VERTEX_POINT ( 'NONE', #6030 ) ;
#2311=ORIENTED_EDGE ( 'NONE', *, *, #12991, .F. ) ;
#2312=CARTESIAN_POINT ( 'NONE',  ( -3.735045420075836212E-15, -26.71562499938548285, 4.662447845253954171 ) ) ;
#2317=DIRECTION ( 'NONE',  ( 0.000000000000000000, 0.000000000000000000, -1.000000000000000000 ) ) ;
#2318=CARTESIAN_POINT ( 'NONE',  ( 20.26302869750798408, 20.26302869750790947, 4.999999999999992006 ) ) ;
#2320=CARTESIAN_POINT ( 'NONE',  ( 1.071796769724495668, 26.65134618820330203, 12.99999999999999112 ) ) ;
#2322=CARTESIAN_POINT ( 'NONE',  ( 16.97933781724378122, 19.63553519520309010, 12.25316411605951927 ) ) ;
#2323=CARTESIAN_POINT ( 'NONE',  ( 18.34500155353947903, 21.17342867828559605, 12.46410161513774639 ) ) ;
#2328=CARTESIAN_POINT ( 'NONE',  ( -3.794751686895379894, 29.75919970560060079, 7.708599238039753665 ) ) ;
#2329=VERTEX_POINT ( 'NONE', #22103 ) ;
#2330=CARTESIAN_POINT ( 'NONE',  ( 15.62472262396960154, 20.93711737988828148, 11.16877607737301048 ) ) ;
#2331=CARTESIAN_POINT ( 'NONE',  ( 3.999999999999996447, -27.92500000000000071, 8.999999999999992895 ) ) ;
#2334=CARTESIAN_POINT ( 'NONE',  ( 4.000000000000001776, 25.80624999877096926, 11.30940107675849760 ) ) ;
#2335=CARTESIAN_POINT ( 'NONE',  ( -1.878215178125000939, -27.31562499938548427, 12.25316411605952283 ) ) ;
#2336=EDGE_CURVE ( 'NONE', #9154, #24945, #19904, .T. ) ;
#2351=CARTESIAN_POINT ( 'NONE',  ( -1.878215178124995832, 27.09062499938548640, 5.746835883940462963 ) ) ;
#2352=CARTESIAN_POINT ( 'NONE',  ( -3.834746474454188013E-15, -27.36250000000000071, 4.999999999999992006 ) ) ;
#2353=LINE ( 'NONE', #18303, #13470 ) ;
#2355=DIRECTION ( 'NONE',  ( 0.000000000000000000, 1.000000000000000000, 0.000000000000000000 ) ) ;
#2356=CARTESIAN_POINT ( 'NONE',  ( 22.19929630020171274, 20.18069571000422968, 12.74788474329069921 ) ) ;
#2358=CARTESIAN_POINT ( 'NONE',  ( 3.999999999999996447, -29.21874999877096712, 8.999999999999992895 ) ) ;
#2361=CARTESIAN_POINT ( 'NONE',  ( -3.999999999999997335, 29.70624999877096784, 11.30940107675849404 ) ) ;
#2362=DIRECTION ( 'NONE',  ( 0.000000000000000000, -0.000000000000000000, 1.000000000000000000 ) ) ;
#2366=ORIENTED_EDGE ( 'NONE', *, *, #1130, .F. ) ;
#2370=ORIENTED_EDGE ( 'NONE', *, *, #15295, .T. ) ;
#2377=CARTESIAN_POINT ( 'NONE',  ( 3.756430356250002323, 27.46562499938548640, 11.16877607737301403 ) ) ;
#2381=CARTESIAN_POINT ( 'NONE',  ( 22.02429405596265610, 16.71189930004383584, 8.999999999999992895 ) ) ;
#2382=CARTESIAN_POINT ( 'NONE',  ( 19.68981756483611889, 21.20556709268809570, 12.99999999999999289 ) ) ;
#2390=VERTEX_POINT ( 'NONE', #14138 ) ;
#2391=ORIENTED_EDGE ( 'NONE', *, *, #19509, .T. ) ;
#2393=ORIENTED_EDGE ( 'NONE', *, *, #5656, .T. ) ;
#2394=DIRECTION ( 'NONE',  ( 0.000000000000000000, -1.000000000000000000, 0.000000000000000000 ) ) ;
#2395=ORIENTED_EDGE ( 'NONE', *, *, #10863, .T. ) ;
#2404=DIRECTION ( 'NONE',  ( 0.000000000000000000, 0.000000000000000000, -1.000000000000000000 ) ) ;
#2407=CARTESIAN_POINT ( 'NONE',  ( 1.878215178125004048, 27.91562499938548569, 5.746835883940462963 ) ) ;
#2410=( BOUNDED_CURVE ( )  B_SPLINE_CURVE ( 2, ( #20214, #4657, #22577, #12110, #22187, #20086, #2188, #619, #14473 ),
 .UNSPECIFIED., .F., .F. ) 
 B_SPLINE_CURVE_WITH_KNOTS ( ( 3, 2, 2, 2, 3 ),
 ( 0.3750000000000000000, 0.3833333333333333592, 0.4000000000000000222, 0.4166666666666666852, 0.4250000000000000444 ),
 .UNSPECIFIED. ) 
 CURVE ( )  GEOMETRIC_REPRESENTATION_ITEM ( )  RATIONAL_B_SPLINE_CURVE ( ( 0.9330127018922194093, 0.9330127018922194093, 1.000000000000000000, 0.8660254037844387076, 1.000000000000000000, 0.8660254037844387076, 1.000000000000000000, 0.9330127018922191873, 0.9330127018922194093 ) ) 
 REPRESENTATION_ITEM ( '' )  );
#2411=CARTESIAN_POINT ( 'NONE',  ( 3.756430356249996105, -25.32812499938548356, 6.831223922626973533 ) ) ;
#2414=ORIENTED_EDGE ( 'NONE', *, *, #7302, .F. ) ;
#2416=CARTESIAN_POINT ( 'NONE',  ( 19.46753356867312235, 19.46753356867304063, 12.99999999999999112 ) ) ;
#2427=CARTESIAN_POINT ( 'NONE',  ( 1.878215178124995832, -26.30312499938548498, 5.746835883940462963 ) ) ;
#2430=ADVANCED_FACE ( 'NONE', ( #20535 ), #12301, .F. ) ;
#2432=EDGE_CURVE ( 'NONE', #6934, #23536, #16699, .T. ) ;
#2440=CARTESIAN_POINT ( 'NONE',  ( 19.46753356867312235, 19.46753356867304063, 12.99999999999999112 ) ) ;
#2443=CARTESIAN_POINT ( 'NONE',  ( 21.06742642710591440, 18.41122904914646341, 5.746835883940462963 ) ) ;
#2444=CARTESIAN_POINT ( 'NONE',  ( 21.96892380712053239, 19.14049668237426616, 5.535898384862238508 ) ) ;
#2445=CARTESIAN_POINT ( 'NONE',  ( -1.999999999999995781, 28.30000000000000071, 5.535898384862237620 ) ) ;
#2448=CARTESIAN_POINT ( 'NONE',  ( -0.5265545572341292502, 29.99647701088549923, 12.97381592328244082 ) ) ;
#2453=FACE_OUTER_BOUND ( 'NONE', #15004, .T. ) ;
#2455=CARTESIAN_POINT ( 'NONE',  ( 3.756430356249997882, -26.75312499938548427, 11.16877607737301226 ) ) ;
#2459=CARTESIAN_POINT ( 'NONE',  ( -3.756430356250002323, -29.71562499938548640, 11.16877607737301226 ) ) ;
#2464=VECTOR ( 'NONE', #11045, 1000.000000000000000 ) ;
#2466=DIRECTION ( 'NONE',  ( 0.000000000000000000, 0.000000000000000000, -1.000000000000000000 ) ) ;
#2470=CARTESIAN_POINT ( 'NONE',  ( -3.756430356249996994, 29.52812499938548640, 8.999999999999992895 ) ) ;
#2479=CARTESIAN_POINT ( 'NONE',  ( -2.000000000000000888, -28.91874999877096997, 12.46410161513774817 ) ) ;
#2486=CARTESIAN_POINT ( 'NONE',  ( 20.46970022635141362, 14.98507572364578699, 8.999999999999992895 ) ) ;
#2494=VERTEX_POINT ( 'NONE', #14405 ) ;
#2496=ORIENTED_EDGE ( 'NONE', *, *, #10513, .T. ) ;
#2502=CARTESIAN_POINT ( 'NONE',  ( -1.878215178124998497, 26.45312499938548711, 12.25316411605951927 ) ) ;
#2503=AXIS2_PLACEMENT_3D ( 'NONE', #6228, #11733, #22193 ) ;
#2508=CARTESIAN_POINT ( 'NONE',  ( 18.49305203628493288, 18.49305203628486183, 4.662447845253954171 ) ) ;
#2513=CARTESIAN_POINT ( 'NONE',  ( -1.999999999999995781, 27.79374999877096997, 5.535898384862237620 ) ) ;
#2517=CARTESIAN_POINT ( 'NONE',  ( 16.64794527869176122, 19.47637240343788179, 5.535898384862237620 ) ) ;
#2520=ORIENTED_EDGE ( 'NONE', *, *, #16662, .F. ) ;
#2532=ORIENTED_EDGE ( 'NONE', *, *, #3191, .F. ) ;
#2533=LINE ( 'NONE', #10122, #10134 ) ;
#2535=CARTESIAN_POINT ( 'NONE',  ( 1.071796769724492338, 28.95759618943233704, 12.99999999999999467 ) ) ;
#2542=CARTESIAN_POINT ( 'NONE',  ( 3.756430356250003655, 28.74062499938548498, 8.999999999999992895 ) ) ;
#2543=EDGE_CURVE ( 'NONE', #23953, #20546, #6287, .T. ) ;
#2544=CARTESIAN_POINT ( 'NONE',  ( 19.23778763078571430, 16.58159025282627397, 5.746835883940462963 ) ) ;
#2548=CARTESIAN_POINT ( 'NONE',  ( -3.999999999999995559, 29.18124999877096926, 6.690598923241487306 ) ) ;
#2550=CARTESIAN_POINT ( 'NONE',  ( -2.672651547586948120E-15, -28.62812499938548783, 13.33755215474603162 ) ) ;
#2555=CARTESIAN_POINT ( 'NONE',  ( 1.999999999999995781, -28.30000000000000071, 5.535898384862237620 ) ) ;
#2565=CARTESIAN_POINT ( 'NONE',  ( -2.672651547586948120E-15, -27.84062499938548640, 13.33755215474603162 ) ) ;
#2567=CARTESIAN_POINT ( 'NONE',  ( -4.000000000000003553, -29.03124999877096712, 6.690598923241489970 ) ) ;
#2571=CIRCLE ( 'NONE', #5914, 26.00000000000000355 ) ;
#2572=CARTESIAN_POINT ( 'NONE',  ( 20.42212772327495784, 20.42212772327488679, 12.99999999999999289 ) ) ;
#2575=CARTESIAN_POINT ( 'NONE',  ( -3.834746474454188013E-15, -28.26249999999999929, 4.999999999999992006 ) ) ;
#2576=VECTOR ( 'NONE', #24031, 1000.000000000000000 ) ;
#2581=CARTESIAN_POINT ( 'NONE',  ( 17.82786595466764012, 20.48406333262694190, 5.746835883940462963 ) ) ;
#2582=CARTESIAN_POINT ( 'NONE',  ( 22.34899370200829338, 16.69213945251583908, 11.30940107675849760 ) ) ;
#2583=CARTESIAN_POINT ( 'NONE',  ( -1.999999999999998224, 28.44999999999999929, 12.46410161513774639 ) ) ;
#2585=( BOUNDED_CURVE ( )  B_SPLINE_CURVE ( 2, ( #18288, #18174, #16471, #4543, #12523, #18044, #6510, #6633, #18418 ),
 .UNSPECIFIED., .F., .F. ) 
 B_SPLINE_CURVE_WITH_KNOTS ( ( 3, 2, 2, 2, 3 ),
 ( 0.2250000000000000056, 0.2333333333333333370, 0.2500000000000000000, 0.2666666666666666630, 0.2750000000000000222 ),
 .UNSPECIFIED. ) 
 CURVE ( )  GEOMETRIC_REPRESENTATION_ITEM ( )  RATIONAL_B_SPLINE_CURVE ( ( 0.9330127018922194093, 0.9330127018922194093, 1.000000000000000000, 0.8660254037844387076, 1.000000000000000000, 0.8660254037844387076, 1.000000000000000000, 0.9330127018922191873, 0.9330127018922194093 ) ) 
 REPRESENTATION_ITEM ( '' )  );
#2587=CARTESIAN_POINT ( 'NONE',  ( -1.039771317798496408, 29.98307469845295969, 12.87134967428165666 ) ) ;
#2591=CARTESIAN_POINT ( 'NONE',  ( 15.30652457243565046, 20.61891932835433394, 11.16877607737301048 ) ) ;
#2592=CARTESIAN_POINT ( 'NONE',  ( 20.41770830676159676, 17.58928118201533408, 5.535898384862238508 ) ) ;
#2594=CARTESIAN_POINT ( 'NONE',  ( 25.99307600111999150, 0.5999999999999998668, 19.00000000000000000 ) ) ;
#2596=CARTESIAN_POINT ( 'NONE',  ( -3.756430356250003655, -25.59062499938548285, 8.999999999999992895 ) ) ;
#2601=CYLINDRICAL_SURFACE ( 'NONE', #12898, 4.000000000000000000 ) ;
#2602=VECTOR ( 'NONE', #11902, 1000.000000000000000 ) ;
#2603=ORIENTED_EDGE ( 'NONE', *, *, #4982, .T. ) ;
#2604=CARTESIAN_POINT ( 'NONE',  ( 3.756430356249997882, -26.75312499938548427, 11.16877607737301226 ) ) ;
#2610=LINE ( 'NONE', #10434, #6412 ) ;
#2614=CARTESIAN_POINT ( 'NONE',  ( 3.735045420075836212E-15, 25.25312499938548783, 4.662447845253954171 ) ) ;
#2616=CARTESIAN_POINT ( 'NONE',  ( 20.46190248058575634, 20.46190248058568173, 12.99999999999999289 ) ) ;
#2621=CARTESIAN_POINT ( 'NONE',  ( -1.878215178125004048, -26.22812499938548569, 5.746835883940462963 ) ) ;
#2625=CARTESIAN_POINT ( 'NONE',  ( -1.071796769724487230, 27.83259618943233704, 4.999999999999992006 ) ) ;
#2628=DIRECTION ( 'NONE',  ( 0.000000000000000000, 0.000000000000000000, -1.000000000000000000 ) ) ;
#2629=ORIENTED_EDGE ( 'NONE', *, *, #8813, .F. ) ;
#2631=ORIENTED_EDGE ( 'NONE', *, *, #16128, .T. ) ;
#2635=ORIENTED_EDGE ( 'NONE', *, *, #1504, .T. ) ;
#2642=CARTESIAN_POINT ( 'NONE',  ( -1.878215178124998497, 28.25312499938548427, 12.25316411605951927 ) ) ;
#2643=VECTOR ( 'NONE', #17666, 1000.000000000000000 ) ;
#2645=CARTESIAN_POINT ( 'NONE',  ( 22.02202058170775345, 19.36582320374829891, 5.746835883940462963 ) ) ;
#2648=CARTESIAN_POINT ( 'NONE',  ( -26.00000000000000355, -1.592040838891558504E-15, 20.00000599999999906 ) ) ;
#2653=CARTESIAN_POINT ( 'NONE',  ( -2.000000000000003997, -25.46874999877096712, 5.535898384862238508 ) ) ;
#2659=ORIENTED_EDGE ( 'NONE', *, *, #5988, .T. ) ;
#2666=EDGE_CURVE ( 'NONE', #18977, #7736, #18968, .T. ) ;
#2675=CARTESIAN_POINT ( 'NONE',  ( 18.09530447186750024, 18.09530447186743629, 13.33755215474602984 ) ) ;
#2677=CARTESIAN_POINT ( 'NONE',  ( 3.756430356250003655, 28.29062499938548569, 8.999999999999992895 ) ) ;
#2682=CARTESIAN_POINT ( 'NONE',  ( -1.878215178125004048, -27.91562499938548569, 5.746835883940462963 ) ) ;
#2686=CARTESIAN_POINT ( 'NONE',  ( 19.62663259444009611, 19.62663259444001085, 4.999999999999992006 ) ) ;
#2695=CARTESIAN_POINT ( 'NONE',  ( -1.878215178125004048, -28.02812499938548640, 5.746835883940462963 ) ) ;
#2696=CARTESIAN_POINT ( 'NONE',  ( 1.071796769724494558, 25.99240381056766580, 4.999999999999992895 ) ) ;
#2704=CARTESIAN_POINT ( 'NONE',  ( 1.878215178125004048, 25.21562499938548285, 5.746835883940462963 ) ) ;
#2706=CARTESIAN_POINT ( 'NONE',  ( 17.16267987305034382, 22.47507462896901842, 6.831223922626973533 ) ) ;
#2707=CARTESIAN_POINT ( 'NONE',  ( 20.51285331117640709, 15.20045855525759393, 8.999999999999992895 ) ) ;
#2713=CARTESIAN_POINT ( 'NONE',  ( 16.87327180006579752, 19.52946917802510285, 5.746835883940462963 ) ) ;
#2714=CARTESIAN_POINT ( 'NONE',  ( 20.42212772327495784, 20.42212772327488679, 12.99999999999999289 ) ) ;
#2717=CARTESIAN_POINT ( 'NONE',  ( -1.999999999999995781, 26.89374999877097139, 5.535898384862237620 ) ) ;
#2718=CARTESIAN_POINT ( 'NONE',  ( 3.756430356249997882, -27.65312499938548640, 11.16877607737301226 ) ) ;
#2720=ORIENTED_EDGE ( 'NONE', *, *, #22691, .T. ) ;
#2722=VERTEX_POINT ( 'NONE', #22885 ) ;
#2723=CARTESIAN_POINT ( 'NONE',  ( 3.756430356249996994, -26.26562499938548711, 8.999999999999992895 ) ) ;
#2726=CARTESIAN_POINT ( 'NONE',  ( -8.831537335106614961E-15, -27.53124999877097068, 12.99999999999999112 ) ) ;
#2727=DIRECTION ( 'NONE',  ( 0.000000000000000000, 0.000000000000000000, -1.000000000000000000 ) ) ;
#2730=CARTESIAN_POINT ( 'NONE',  ( 1.071796769724498999, 27.60759618943233207, 12.99999999999998757 ) ) ;
#2733=CARTESIAN_POINT ( 'NONE',  ( -2.000000000000003997, -27.26874999877097139, 5.535898384862238508 ) ) ;
#2735=CARTESIAN_POINT ( 'NONE',  ( 1.878215178125000939, 29.56562499938548427, 12.25316411605952283 ) ) ;
#2736=CARTESIAN_POINT ( 'NONE',  ( 16.94404624418269023, 22.60090049367499532, 11.30940107675849404 ) ) ;
#2742=CARTESIAN_POINT ( 'NONE',  ( 17.46243120409849325, 18.97818073195047361, 12.99999999999999467 ) ) ;
#2743=CARTESIAN_POINT ( 'NONE',  ( -2.672651547586948120E-15, -26.94062499938548783, 13.33755215474602984 ) ) ;
#2745=CARTESIAN_POINT ( 'NONE',  ( -3.469446951953614189E-15, -30.00000000000000355, 8.999999999999992895 ) ) ;
#2747=CARTESIAN_POINT ( 'NONE',  ( -3.999999999999996447, 27.92500000000000071, 8.999999999999992895 ) ) ;
#2751=DIRECTION ( 'NONE',  ( -0.7071067811865487940, -0.7071067811865463515, 0.000000000000000000 ) ) ;
#2758=FACE_OUTER_BOUND ( 'NONE', #3165, .T. ) ;
#2761=CARTESIAN_POINT ( 'NONE',  ( 3.756430356250003655, 27.95312499938548711, 8.999999999999992895 ) ) ;
#2765=CARTESIAN_POINT ( 'NONE',  ( 23.32360276639294128, 18.01120801047411746, 6.831223922626973533 ) ) ;
#2767=CARTESIAN_POINT ( 'NONE',  ( 17.55392584295608316, 23.21078009244839180, 8.999999999999992895 ) ) ;
#2783=ORIENTED_EDGE ( 'NONE', *, *, #15065, .F. ) ;
#2784=CARTESIAN_POINT ( 'NONE',  ( 3.756430356249995661, -25.44062499938548427, 6.831223922626973533 ) ) ;
#2793=CARTESIAN_POINT ( 'NONE',  ( 15.99595368409253915, 21.30834844001121553, 8.999999999999992895 ) ) ;
#2794=EDGE_CURVE ( 'NONE', #22706, #23573, #3253, .T. ) ;
#2795=CARTESIAN_POINT ( 'NONE',  ( 3.756430356250004099, 27.87812499938548427, 6.831223922626973533 ) ) ;
#2802=FACE_OUTER_BOUND ( 'NONE', #6159, .T. ) ;
#2803=CARTESIAN_POINT ( 'NONE',  ( -3.756430356250002323, -28.25312499938548427, 11.16877607737301403 ) ) ;
#2811=CARTESIAN_POINT ( 'NONE',  ( -1.859271017917182139E-15, -29.33124999877096428, 12.99999999999999289 ) ) ;
#2815=CARTESIAN_POINT ( 'NONE',  ( -1.878215178125004048, -25.77812499938548640, 5.746835883940462963 ) ) ;
#2823=CARTESIAN_POINT ( 'NONE',  ( 3.756430356250003655, 25.25312499938548427, 8.999999999999992895 ) ) ;
#2827=CARTESIAN_POINT ( 'NONE',  ( 17.92073748482754780, 20.74916460957366127, 5.535898384862237620 ) ) ;
#2829=CARTESIAN_POINT ( 'NONE',  ( 17.18919637734483885, 22.50159113326351346, 8.999999999999992895 ) ) ;
#2830=CARTESIAN_POINT ( 'NONE',  ( 16.31415173562648491, 21.62654649154516306, 8.999999999999992895 ) ) ;
#2835=( BOUNDED_CURVE ( )  B_SPLINE_CURVE ( 2, ( #14910, #15176, #1047, #18961, #19203, #5345, #23145, #3383, #9282 ),
 .UNSPECIFIED., .F., .F. ) 
 B_SPLINE_CURVE_WITH_KNOTS ( ( 3, 2, 2, 2, 3 ),
 ( 0.6250000000000000000, 0.6333333333333333037, 0.6500000000000000222, 0.6666666666666666297, 0.6750000000000000444 ),
 .UNSPECIFIED. ) 
 CURVE ( )  GEOMETRIC_REPRESENTATION_ITEM ( )  RATIONAL_B_SPLINE_CURVE ( ( 0.9330127018922194093, 0.9330127018922194093, 1.000000000000000000, 0.8660254037844387076, 1.000000000000000000, 0.8660254037844387076, 1.000000000000000000, 0.9330127018922189652, 0.9330127018922194093 ) ) 
 REPRESENTATION_ITEM ( '' )  );
#2836=CARTESIAN_POINT ( 'NONE',  ( 20.72498534553237093, 15.41259058961355954, 11.16877607737301403 ) ) ;
#2839=CARTESIAN_POINT ( 'NONE',  ( 3.834746474454188013E-15, 27.81249999999999645, 4.999999999999992006 ) ) ;
#2840=CARTESIAN_POINT ( 'NONE',  ( 2.000000000000000888, 28.46874999877097068, 12.46410161513774817 ) ) ;
#2841=CARTESIAN_POINT ( 'NONE',  ( -3.756430356250004099, -28.77812499938548285, 6.831223922626973533 ) ) ;
#2847=CARTESIAN_POINT ( 'NONE',  ( -1.878215178125004048, -25.66562499938548569, 5.746835883940462963 ) ) ;
#2849=ORIENTED_EDGE ( 'NONE', *, *, #20421, .F. ) ;
#2856=CARTESIAN_POINT ( 'NONE',  ( 3.137519842735244810E-15, -27.30624999877096926, 4.999999999999991118 ) ) ;
#2857=CARTESIAN_POINT ( 'NONE',  ( -3.756430356249995661, 28.47812499938548569, 6.831223922626973533 ) ) ;
#2864=CARTESIAN_POINT ( 'NONE',  ( 4.000000000000003553, 25.84374999877096712, 8.999999999999992895 ) ) ;
#2866=CARTESIAN_POINT ( 'NONE',  ( 3.756430356249995661, -26.79062499938548925, 6.831223922626973533 ) ) ;
#2870=CARTESIAN_POINT ( 'NONE',  ( 1.289143957944685281, -29.97326948525437729, 12.79562863665509553 ) ) ;
#2876=VERTEX_POINT ( 'NONE', #13983 ) ;
#2879=VECTOR ( 'NONE', #23809, 1000.000000000000000 ) ;
#2882=ORIENTED_EDGE ( 'NONE', *, *, #11177, .F. ) ;
#2886=CARTESIAN_POINT ( 'NONE',  ( 2.672651547586948120E-15, 29.19062499938548427, 13.33755215474603162 ) ) ;
#2890=CARTESIAN_POINT ( 'NONE',  ( 4.000000000000001776, 29.46250000000000213, 11.30940107675849760 ) ) ;
#2891=CARTESIAN_POINT ( 'NONE',  ( 3.735045420075836212E-15, 26.71562499938548640, 4.662447845253954171 ) ) ;
#2892=CIRCLE ( 'NONE', #10395, 4.000000000000000000 ) ;
#2893=CARTESIAN_POINT ( 'NONE',  ( 17.18149551509901585, -19.58805710660145749, 20.00001200000000168 ) ) ;
#2897=DIRECTION ( 'NONE',  ( 0.000000000000000000, 0.000000000000000000, -1.000000000000000000 ) ) ;
#2898=CYLINDRICAL_SURFACE ( 'NONE', #16642, 4.000000000000000000 ) ;
#2902=CARTESIAN_POINT ( 'NONE',  ( 1.626862140677534194E-14, 27.98124999877096997, 12.99999999999999289 ) ) ;
#2913=ORIENTED_EDGE ( 'NONE', *, *, #13233, .T. ) ;
#2914=CARTESIAN_POINT ( 'NONE',  ( -3.756430356250003655, -26.60312499938548569, 8.999999999999992895 ) ) ;
#2916=ORIENTED_EDGE ( 'NONE', *, *, #3429, .T. ) ;
#2928=CARTESIAN_POINT ( 'NONE',  ( -1.999999999999998224, 28.39374999877096784, 12.46410161513774639 ) ) ;
#2929=CARTESIAN_POINT ( 'NONE',  ( 22.13036007314063625, 16.81796531722181598, 6.831223922626973533 ) ) ;
#2932=CARTESIAN_POINT ( 'NONE',  ( 1.878215178125004048, 27.46562499938548640, 5.746835883940462963 ) ) ;
#2934=CARTESIAN_POINT ( 'NONE',  ( 15.67775563255858984, 20.99015038847727155, 8.999999999999992895 ) ) ;
#2936=EDGE_LOOP ( 'NONE', ( #14382, #3286, #21484, #21600 ) ) ;
#2938=CARTESIAN_POINT ( 'NONE',  ( -3.999999999999997335, 29.31250000000000000, 11.30940107675849404 ) ) ;
#2939=CARTESIAN_POINT ( 'NONE',  ( 3.756430356249996105, -26.67812499938548498, 6.831223922626973533 ) ) ;
#2954=CARTESIAN_POINT ( 'NONE',  ( -1.878215178125004048, -28.92812499938548854, 5.746835883940462963 ) ) ;
#2955=CARTESIAN_POINT ( 'NONE',  ( 1.071796769724492338, 25.80759618943233491, 12.99999999999999467 ) ) ;
#2958=ADVANCED_FACE ( 'NONE', ( #25742 ), #21757, .F. ) ;
#2962=LINE ( 'NONE', #1003, #6270 ) ;
#2964=VECTOR ( 'NONE', #10548, 1000.000000000000000 ) ;
#2967=CARTESIAN_POINT ( 'NONE',  ( 1.071796769724494558, 25.54240381056766651, 4.999999999999992895 ) ) ;
#2968=CARTESIAN_POINT ( 'NONE',  ( 23.61528431363239022, 18.30288955771356640, 8.999999999999992895 ) ) ;
#2969=CARTESIAN_POINT ( 'NONE',  ( 21.78564551731219723, 16.47325076139337696, 8.999999999999992895 ) ) ;
#2970=CARTESIAN_POINT ( 'NONE',  ( -1.071796769724487230, 28.28259618943233988, 4.999999999999992006 ) ) ;
#2974=CARTESIAN_POINT ( 'NONE',  ( 19.92494326818769323, 19.92494326818762218, 13.33755215474603162 ) ) ;
#2978=CARTESIAN_POINT ( 'NONE',  ( 2.620986760973688460E-15, 27.08124999877096784, 13.61880215351699874 ) ) ;
#2979=CARTESIAN_POINT ( 'NONE',  ( -1.878215178125004048, -28.81562499938548427, 5.746835883940462963 ) ) ;
#2980=CARTESIAN_POINT ( 'NONE',  ( -1.071796769724487230, 25.52634618820330559, 4.999999999999992006 ) ) ;
#2981=EDGE_LOOP ( 'NONE', ( #7500, #17396, #15813, #10815 ) ) ;
#2982=DIRECTION ( 'NONE',  ( 0.000000000000000000, 0.000000000000000000, -1.000000000000000000 ) ) ;
#2985=EDGE_CURVE ( 'NONE', #256, #20149, #3675, .T. ) ;
#2986=CARTESIAN_POINT ( 'NONE',  ( 3.756430356249996994, -28.51562499938548356, 8.999999999999992895 ) ) ;
#2990=AXIS2_PLACEMENT_3D ( 'NONE', #6251, #22211, #18285 ) ;
#2994=VECTOR ( 'NONE', #13283, 1000.000000000000000 ) ;
#2998=CARTESIAN_POINT ( 'NONE',  ( 3.756430356250004099, 27.42812499938548143, 6.831223922626973533 ) ) ;
#3003=DIRECTION ( 'NONE',  ( -1.000000000000000000, 0.000000000000000000, 0.000000000000000000 ) ) ;
#3006=CARTESIAN_POINT ( 'NONE',  ( 3.756430356249997882, -27.31562499938548427, 11.16877607737301226 ) ) ;
#3011=CARTESIAN_POINT ( 'NONE',  ( -3.369928719974892281E-15, -25.11250000000000426, 4.999999999999992006 ) ) ;
#3013=ORIENTED_EDGE ( 'NONE', *, *, #24748, .F. ) ;
#3016=ORIENTED_EDGE ( 'NONE', *, *, #24073, .F. ) ;
#3020=EDGE_LOOP ( 'NONE', ( #7483, #3106, #5006, #12106 ) ) ;
#3023=FACE_OUTER_BOUND ( 'NONE', #12961, .T. ) ;
#3027=CARTESIAN_POINT ( 'NONE',  ( -1.878215178124998497, 27.80312499938548498, 12.25316411605951927 ) ) ;
#3033=CARTESIAN_POINT ( 'NONE',  ( 22.63417365473605614, 17.32177889881723587, 11.16877607737301226 ) ) ;
#3034=CARTESIAN_POINT ( 'NONE',  ( 3.735045420075836212E-15, 25.81562499938548783, 4.662447845253954171 ) ) ;
#3035=EDGE_CURVE ( 'NONE', #24788, #6934, #13017, .T. ) ;
#3036=CARTESIAN_POINT ( 'NONE',  ( -26.00000000000000355, -1.701696020694477784, 20.00001200000000523 ) ) ;
#3044=CARTESIAN_POINT ( 'NONE',  ( -4.000000000000003553, -25.44999999999999929, 8.999999999999992895 ) ) ;
#3045=ORIENTED_EDGE ( 'NONE', *, *, #13540, .F. ) ;
#3047=CIRCLE ( 'NONE', #9302, 0.7500000000000001110 ) ;
#3050=ORIENTED_EDGE ( 'NONE', *, *, #16961, .F. ) ;
#3051=CARTESIAN_POINT ( 'NONE',  ( -3.756430356250004099, -25.29062499938548569, 6.831223922626973533 ) ) ;
#3061=CARTESIAN_POINT ( 'NONE',  ( 16.95282131294928263, 19.60901869090858796, 5.746835883940462963 ) ) ;
#3065=CARTESIAN_POINT ( 'NONE',  ( -3.999999999999996003, 25.18750000000000000, 6.690598923241487306 ) ) ;
#3066=CARTESIAN_POINT ( 'NONE',  ( 21.78564551731219723, 16.47325076139337696, 8.999999999999992895 ) ) ;
#3067=LINE ( 'NONE', #17197, #6170 ) ;
#3071=CARTESIAN_POINT ( 'NONE',  ( -2.672651547586948120E-15, -26.37812499938548427, 13.33755215474603162 ) ) ;
#3082=EDGE_CURVE ( 'NONE', #25535, #3881, #18056, .T. ) ;
#3083=CARTESIAN_POINT ( 'NONE',  ( 1.878215178124998497, -29.15312499938548640, 12.25316411605951927 ) ) ;
#3087=CARTESIAN_POINT ( 'NONE',  ( -3.834746474454188013E-15, -26.40624999877096357, 4.999999999999992006 ) ) ;
#3089=EDGE_CURVE ( 'NONE', #25106, #25535, #15412, .T. ) ;
#3092=EDGE_CURVE ( 'NONE', #22272, #24945, #987, .T. ) ;
#3094=DIRECTION ( 'NONE',  ( 0.000000000000000000, 1.000000000000000000, 0.000000000000000000 ) ) ;
#3095=CARTESIAN_POINT ( 'NONE',  ( 1.878215178125000939, 26.41562499938548214, 12.25316411605952283 ) ) ;
#3097=CARTESIAN_POINT ( 'NONE',  ( 16.68772003600256326, 19.51614716074868028, 5.535898384862237620 ) ) ;
#3098=CARTESIAN_POINT ( 'NONE',  ( 21.46744746577824969, 16.15505270985943298, 8.999999999999992895 ) ) ;
#3102=ADVANCED_FACE ( 'NONE', ( #7126 ), #10771, .F. ) ;
#3104=CARTESIAN_POINT ( 'NONE',  ( 16.55280027427694378, 21.86519503019561839, 8.999999999999992895 ) ) ;
#3106=ORIENTED_EDGE ( 'NONE', *, *, #10429, .T. ) ;
#3108=CARTESIAN_POINT ( 'NONE',  ( -3.999999999999996447, 28.31874999877096855, 8.999999999999992895 ) ) ;
#3109=CARTESIAN_POINT ( 'NONE',  ( 1.878215178124998497, -29.04062499938548569, 12.25316411605951927 ) ) ;
#3111=EDGE_LOOP ( 'NONE', ( #11503, #18488, #17315, #16475 ) ) ;
#3114=CARTESIAN_POINT ( 'NONE',  ( -1.878215178125004048, -29.26562499938548356, 5.746835883940462963 ) ) ;
#3117=CARTESIAN_POINT ( 'NONE',  ( 18.21587718922017984, 23.83662110555050617, 8.477544402765669673 ) ) ;
#3123=CARTESIAN_POINT ( 'NONE',  ( 3.756430356250003655, 29.19062499938548072, 8.999999999999992895 ) ) ;
#3134=CARTESIAN_POINT ( 'NONE',  ( -3.756430356250002323, -27.46562499938548640, 11.16877607737301226 ) ) ;
#3138=CARTESIAN_POINT ( 'NONE',  ( -1.999999999999998224, 26.14374999877096784, 12.46410161513774639 ) ) ;
#3139=CARTESIAN_POINT ( 'NONE',  ( 3.015186248472646824, -29.84868090056883716, 11.64163568064553544 ) ) ;
#3143=ORIENTED_EDGE ( 'NONE', *, *, #12221, .T. ) ;
#3147=EDGE_LOOP ( 'NONE', ( #22884, #22206 ) ) ;
#3151=CARTESIAN_POINT ( 'NONE',  ( -3.756430356249996994, 28.62812499938548427, 8.999999999999992895 ) ) ;
#3154=CARTESIAN_POINT ( 'NONE',  ( 3.756430356250002323, 26.56562499938548427, 11.16877607737301226 ) ) ;
#3155=CARTESIAN_POINT ( 'NONE',  ( -22.56362157461193618, -13.02991752792603641, 20.00001200000000168 ) ) ;
#3157=CYLINDRICAL_SURFACE ( 'NONE', #25471, 4.000000000000000000 ) ;
#3159=CARTESIAN_POINT ( 'NONE',  ( -2.000000000000000888, -29.42500000000000071, 12.46410161513774817 ) ) ;
#3165=EDGE_LOOP ( 'NONE', ( #2913, #12994, #16862, #15874 ) ) ;
#3171=CARTESIAN_POINT ( 'NONE',  ( -3.735045420075836212E-15, -26.26562499938548356, 4.662447845253954171 ) ) ;
#3172=ORIENTED_EDGE ( 'NONE', *, *, #12772, .F. ) ;
#3174=EDGE_CURVE ( 'NONE', #12039, #2722, #14972, .T. ) ;
#3175=ORIENTED_EDGE ( 'NONE', *, *, #10574, .T. ) ;
#3181=CARTESIAN_POINT ( 'NONE',  ( 18.89079960070236908, 18.89079960070229802, 4.662447845253954171 ) ) ;
#3182=CARTESIAN_POINT ( 'NONE',  ( 0.000000000000000000, 10.00000000000000000, 15.00000000000000178 ) ) ;
#3183=CARTESIAN_POINT ( 'NONE',  ( 2.620986760973688460E-15, 25.78750000000000142, 13.61880215351699874 ) ) ;
#3184=CARTESIAN_POINT ( 'NONE',  ( 19.87418373385361292, 17.21798635589416548, 5.746835883940462963 ) ) ;
#3189=DIRECTION ( 'NONE',  ( 0.000000000000000000, 1.000000000000000000, 0.000000000000000000 ) ) ;
#3191=EDGE_CURVE ( 'NONE', #19876, #939, #20714, .T. ) ;
#3199=CARTESIAN_POINT ( 'NONE',  ( 3.756430356249996105, -28.59062499938548640, 6.831223922626973533 ) ) ;
#3209=CARTESIAN_POINT ( 'NONE',  ( -3.756430356249997438, 27.65312499938548640, 11.16877607737301048 ) ) ;
#3210=CARTESIAN_POINT ( 'NONE',  ( -3.795382382264993915, -29.75912104221810495, 7.710170883190207824 ) ) ;
#3211=CARTESIAN_POINT ( 'NONE',  ( 18.23451611984813070, 18.23451611984806320, 13.61880215351699874 ) ) ;
#3212=CARTESIAN_POINT ( 'NONE',  ( 19.23778763078571430, 16.58159025282627397, 5.746835883940462963 ) ) ;
#3213=CARTESIAN_POINT ( 'NONE',  ( 19.24094079118243528, 20.75669031903440143, 4.999999999999992006 ) ) ;
#3216=CARTESIAN_POINT ( 'NONE',  ( 18.25213002337956780, 20.90832740133887313, 12.25316411605951927 ) ) ;
#3218=ORIENTED_EDGE ( 'NONE', *, *, #9576, .T. ) ;
#3219=CARTESIAN_POINT ( 'NONE',  ( 21.48720731330624645, 15.83035306381379748, 6.690598923241489970 ) ) ;
#3220=CARTESIAN_POINT ( 'NONE',  ( 4.000000000000003553, 27.23124999877096997, 6.690598923241489970 ) ) ;
#3221=CARTESIAN_POINT ( 'NONE',  ( -2.672651547586948120E-15, -29.07812499938548001, 13.33755215474602984 ) ) ;
#3226=ORIENTED_EDGE ( 'NONE', *, *, #16093, .T. ) ;
#3227=CARTESIAN_POINT ( 'NONE',  ( -1.878215178125004048, -27.46562499938548640, 5.746835883940462963 ) ) ;
#3231=CARTESIAN_POINT ( 'NONE',  ( 19.92166635246234563, 22.43180781836643689, 5.405792698933812979 ) ) ;
#3238=FACE_OUTER_BOUND ( 'NONE', #21154, .T. ) ;
#3239=CARTESIAN_POINT ( 'NONE',  ( 3.469446951953614189E-15, 30.00000000000000355, 8.999999999999992895 ) ) ;
#3244=CARTESIAN_POINT ( 'NONE',  ( -1.999999999999998224, 27.55000000000000071, 12.46410161513774639 ) ) ;
#3245=CARTESIAN_POINT ( 'NONE',  ( 3.756430356249995661, -29.04062499938548569, 6.831223922626973533 ) ) ;
#3247=DIRECTION ( 'NONE',  ( -0.000000000000000000, -1.000000000000000000, -0.000000000000000000 ) ) ;
#3249=CARTESIAN_POINT ( 'NONE',  ( 5.577813053751546416E-15, 25.73124999877096997, 12.99999999999999289 ) ) ;
#3253=LINE ( 'NONE', #20931, #8786 ) ;
#3257=ORIENTED_EDGE ( 'NONE', *, *, #16568, .T. ) ;
#3261=CARTESIAN_POINT ( 'NONE',  ( 21.21320343559646915, 21.21320343559638744, 8.999999999999992895 ) ) ;
#3262=( BOUNDED_CURVE ( )  B_SPLINE_CURVE ( 2, ( #24709, #8751, #14781, #12546, #16879, #7183, #4715, #6799, #4833 ),
 .UNSPECIFIED., .F., .F. ) 
 B_SPLINE_CURVE_WITH_KNOTS ( ( 3, 2, 2, 2, 3 ),
 ( 0.5250000000000000222, 0.5333333333333333259, 0.5500000000000000444, 0.5666666666666666519, 0.5750000000000000666 ),
 .UNSPECIFIED. ) 
 CURVE ( )  GEOMETRIC_REPRESENTATION_ITEM ( )  RATIONAL_B_SPLINE_CURVE ( ( 0.9330127018922194093, 0.9330127018922194093, 1.000000000000000000, 0.8660254037844387076, 1.000000000000000000, 0.8660254037844387076, 1.000000000000000000, 0.9330127018922189652, 0.9330127018922194093 ) ) 
 REPRESENTATION_ITEM ( '' )  );
#3270=SURFACE_STYLE_USAGE ( .BOTH. , #1455 ) ;
#3271=CARTESIAN_POINT ( 'NONE',  ( 3.756430356250003655, 26.15312499938548640, 8.999999999999992895 ) ) ;
#3280=CARTESIAN_POINT ( 'NONE',  ( -3.752267015613588906E-15, -27.75624999877096855, 4.381197846482986158 ) ) ;
#3282=AXIS2_PLACEMENT_3D ( 'NONE', #23179, #20968, #8801 ) ;
#3286=ORIENTED_EDGE ( 'NONE', *, *, #20421, .T. ) ;
#3287=CARTESIAN_POINT ( 'NONE',  ( -1.859271017917182139E-15, -28.93749999999999645, 12.99999999999999289 ) ) ;
#3289=ORIENTED_EDGE ( 'NONE', *, *, #3082, .F. ) ;
#3291=VERTEX_POINT ( 'NONE', #23465 ) ;
#3292=CARTESIAN_POINT ( 'NONE',  ( 3.756430356249997882, -28.66562499938548569, 11.16877607737301226 ) ) ;
#3297=VERTEX_POINT ( 'NONE', #17715 ) ;
#3301=EDGE_CURVE ( 'NONE', #4358, #4649, #25300, .T. ) ;
#3305=CARTESIAN_POINT ( 'NONE',  ( 15.96943717979804056, 21.28183193571671694, 6.831223922626973533 ) ) ;
#3307=CARTESIAN_POINT ( 'NONE',  ( -3.756430356249996994, 29.41562499938548569, 8.999999999999992895 ) ) ;
#3310=CARTESIAN_POINT ( 'NONE',  ( 17.05888733012726632, 19.71508470808657520, 12.25316411605951927 ) ) ;
#3325=VECTOR ( 'NONE', #6932, 1000.000000000000000 ) ;
#3327=CARTESIAN_POINT ( 'NONE',  ( -2.672651547586948120E-15, -28.74062499938548854, 13.33755215474603162 ) ) ;
#3328=EDGE_CURVE ( 'NONE', #23126, #8456, #20923, .T. ) ;
#3333=CARTESIAN_POINT ( 'NONE',  ( -4.000000000000003553, -26.33124999877097139, 6.690598923241489970 ) ) ;
#3335=EDGE_CURVE ( 'NONE', #23467, #22705, #5522, .T. ) ;
#3341=CARTESIAN_POINT ( 'NONE',  ( 1.878215178125000939, 25.96562499938548285, 12.25316411605952283 ) ) ;
#3344=CARTESIAN_POINT ( 'NONE',  ( 17.82559248041273037, 23.13798723633140142, 8.999999999999992895 ) ) ;
#3345=CARTESIAN_POINT ( 'NONE',  ( 19.18020767368691182, 21.83640505164621004, 5.746835883940462963 ) ) ;
#3350=VECTOR ( 'NONE', #7404, 1000.000000000000000 ) ;
#3351=CARTESIAN_POINT ( 'NONE',  ( 17.48087792458429135, 22.79327268050296240, 6.831223922626973533 ) ) ;
#3352=CARTESIAN_POINT ( 'NONE',  ( 21.22646168687465007, 18.39803456212839450, 12.46410161513774817 ) ) ;
#3355=CARTESIAN_POINT ( 'NONE',  ( -3.999999999999996447, 29.21874999877096712, 8.999999999999992895 ) ) ;
#3356=CARTESIAN_POINT ( 'NONE',  ( 3.756430356249995661, -28.47812499938548569, 6.831223922626973533 ) ) ;
#3361=CARTESIAN_POINT ( 'NONE',  ( -3.756430356250003655, -28.29062499938548569, 8.999999999999992895 ) ) ;
#3372=CARTESIAN_POINT ( 'NONE',  ( 1.071796769724490117, -27.32634618820330630, 4.999999999999992895 ) ) ;
#3382=CARTESIAN_POINT ( 'NONE',  ( 1.878215178124998497, -29.60312499938548569, 12.25316411605951927 ) ) ;
#3383=CARTESIAN_POINT ( 'NONE',  ( 19.33184475599137642, 20.84759428384334612, 12.99999999999999645 ) ) ;
#3384=FACE_OUTER_BOUND ( 'NONE', #17340, .T. ) ;
#3389=LINE ( 'NONE', #25356, #15108 ) ;
#3404=AXIS2_PLACEMENT_3D ( 'NONE', #10880, #15085, #20428 ) ;
#3407=( LENGTH_UNIT ( ) NAMED_UNIT ( * ) SI_UNIT ( .MILLI., .METRE. ) );
#3408=CARTESIAN_POINT ( 'NONE',  ( 1.878215178125000939, 26.07812499938548356, 12.25316411605952283 ) ) ;
#3410=CARTESIAN_POINT ( 'NONE',  ( 2.000000000000000888, 28.46874999877097068, 12.46410161513774817 ) ) ;
#3412=CIRCLE ( 'NONE', #21782, 24.00000000000000355 ) ;
#3414=CYLINDRICAL_SURFACE ( 'NONE', #19130, 24.00000000000000355 ) ;
#3418=CARTESIAN_POINT ( 'NONE',  ( 3.999999999999996447, -26.51874999877097139, 8.999999999999992895 ) ) ;
#3423=CARTESIAN_POINT ( 'NONE',  ( -1.859271017917182139E-15, -25.78750000000000142, 12.99999999999999289 ) ) ;
#3427=VERTEX_POINT ( 'NONE', #584 ) ;
#3428=( BOUNDED_CURVE ( )  B_SPLINE_CURVE ( 2, ( #11248, #23167, #3410, #17157, #19612, #3540, #19228, #1458, #9429 ),
 .UNSPECIFIED., .F., .F. ) 
 B_SPLINE_CURVE_WITH_KNOTS ( ( 3, 2, 2, 2, 3 ),
 ( 0.6750000000000000444, 0.6833333333333333481, 0.6999999999999999556, 0.7166666666666666741, 0.7249999999999999778 ),
 .UNSPECIFIED. ) 
 CURVE ( )  GEOMETRIC_REPRESENTATION_ITEM ( )  RATIONAL_B_SPLINE_CURVE ( ( 0.9330127018922194093, 0.9330127018922198534, 1.000000000000000000, 0.8660254037844387076, 1.000000000000000000, 0.8660254037844387076, 1.000000000000000000, 0.9330127018922194093, 0.9330127018922194093 ) ) 
 REPRESENTATION_ITEM ( '' )  );
#3429=EDGE_CURVE ( 'NONE', #3297, #4579, #8394, .T. ) ;
#3432=CYLINDRICAL_SURFACE ( 'NONE', #11683, 8.000000000000000000 ) ;
#3434=CARTESIAN_POINT ( 'NONE',  ( -2.672651547586948120E-15, -28.29062499938548569, 13.33755215474602984 ) ) ;
#3444=CARTESIAN_POINT ( 'NONE',  ( 3.469446951953614189E-15, 30.00000000000000355, 8.999999999999992895 ) ) ;
#3445=CARTESIAN_POINT ( 'NONE',  ( 19.47643616943617317, 16.82023879147673284, 5.746835883940462963 ) ) ;
#3447=CARTESIAN_POINT ( 'NONE',  ( -3.999999999999997335, 26.61250000000000071, 11.30940107675849404 ) ) ;
#3449=CARTESIAN_POINT ( 'NONE',  ( 16.02247018838703241, 21.33486494430571412, 11.16877607737301048 ) ) ;
#3453=ORIENTED_EDGE ( 'NONE', *, *, #12991, .T. ) ;
#3455=CARTESIAN_POINT ( 'NONE',  ( -3.735045420075836212E-15, -29.30312499938548498, 4.662447845253954171 ) ) ;
#3463=CARTESIAN_POINT ( 'NONE',  ( 18.35384038830430597, 18.35384038830423492, 4.999999999999992006 ) ) ;
#3467=ORIENTED_EDGE ( 'NONE', *, *, #2794, .T. ) ;
#3468=CARTESIAN_POINT ( 'NONE',  ( -1.071796769724487230, 25.58259618943233704, 4.999999999999992006 ) ) ;
#3478=CARTESIAN_POINT ( 'NONE',  ( 3.735045420075836212E-15, 27.50312499938548427, 4.662447845253954171 ) ) ;
#3479=DIRECTION ( 'NONE',  ( 0.8660254037844397068, 0.4999999999999983347, -0.000000000000000000 ) ) ;
#3480=CARTESIAN_POINT ( 'NONE',  ( 18.78246010926947918, 21.43865748722877740, 5.746835883940462963 ) ) ;
#3481=CARTESIAN_POINT ( 'NONE',  ( 16.97706434298888212, 22.28945909890755317, 11.16877607737301226 ) ) ;
#3484=DIRECTION ( 'NONE',  ( 0.000000000000000000, -1.000000000000000000, 0.000000000000000000 ) ) ;
#3485=CARTESIAN_POINT ( 'NONE',  ( 21.21320343559646915, 21.21320343559638744, 4.999999999999992006 ) ) ;
#3487=CARTESIAN_POINT ( 'NONE',  ( 17.16267987305034382, 22.47507462896901842, 6.831223922626973533 ) ) ;
#3488=DIRECTION ( 'NONE',  ( 0.000000000000000000, 1.000000000000000000, 0.000000000000000000 ) ) ;
#3491=CARTESIAN_POINT ( 'NONE',  ( 1.878215178125004048, 26.67812499938548498, 5.746835883940462963 ) ) ;
#3492=CARTESIAN_POINT ( 'NONE',  ( -4.000000000000003553, -25.93750000000000000, 6.690598923241489970 ) ) ;
#3495=CARTESIAN_POINT ( 'NONE',  ( -1.859271017917182139E-15, -28.93749999999999645, 12.99999999999999289 ) ) ;
#3497=CARTESIAN_POINT ( 'NONE',  ( -17.18149551509903361, 19.58805710660143973, 20.00001200000000168 ) ) ;
#3498=CARTESIAN_POINT ( 'NONE',  ( 1.878215178124995832, -28.89062499938548356, 5.746835883940462963 ) ) ;
#3499=ORIENTED_EDGE ( 'NONE', *, *, #8418, .F. ) ;
#3501=CARTESIAN_POINT ( 'NONE',  ( 18.51824573262021190, 23.60264142991855252, 7.227341970420264161 ) ) ;
#3508=B_SPLINE_CURVE_WITH_KNOTS ( 'NONE', 3,
 ( #25594, #11336, #5705, #21657, #5454, #25457, #9638, #13822, #15661, #25334, #1924, #21416, #1800, #17871, #11724, #9769, #23746, #9502, #5835, #13569, #9885, #25843, #11469, #21278, #3497, #5323, #9387, #13304, #7541, #17617, #15535, #23502, #5589, #21534 ),
 .UNSPECIFIED., .F., .F.,
 ( 4, 2, 2, 2, 2, 2, 2, 2, 2, 2, 2, 2, 2, 2, 2, 2, 4 ),
 ( 0.000000000000000000, 0.03124999999999998612, 0.06249999999999995837, 0.09374999999999993061, 0.1249999999999999029, 0.1562499999999998890, 0.1874999999999998890, 0.2187499999999998890, 0.2499999999999998890, 0.2812499999999998890, 0.3124999999999998890, 0.3437499999999998335, 0.3749999999999998335, 0.4062499999999998335, 0.4374999999999998335, 0.4687499999999998890, 0.5000000000000000000 ),
 .UNSPECIFIED. ) ;
#3511=CARTESIAN_POINT ( 'NONE',  ( 4.000000000000003553, 28.63749999999999929, 6.690598923241489970 ) ) ;
#3514=CARTESIAN_POINT ( 'NONE',  ( 18.67203843983824996, 18.67203843983817890, 4.381197846482986158 ) ) ;
#3515=ORIENTED_EDGE ( 'NONE', *, *, #10429, .F. ) ;
#3516=FACE_BOUND ( 'NONE', #24979, .T. ) ;
#3520=CARTESIAN_POINT ( 'NONE',  ( 4.000000000000003553, 27.28749999999999787, 6.690598923241489970 ) ) ;
#3521=CARTESIAN_POINT ( 'NONE',  ( 4.000000000000001776, 28.95624999877097494, 11.30940107675849760 ) ) ;
#3522=ORIENTED_EDGE ( 'NONE', *, *, #3035, .F. ) ;
#3525=CARTESIAN_POINT ( 'NONE',  ( -4.000000000000003553, -26.35000000000000142, 8.999999999999992895 ) ) ;
#3530=ADVANCED_FACE ( 'NONE', ( #5147 ), #11696, .F. ) ;
#3538=CARTESIAN_POINT ( 'NONE',  ( -3.756430356249995661, 27.24062499938548498, 6.831223922626973533 ) ) ;
#3540=CARTESIAN_POINT ( 'NONE',  ( 4.000000000000003553, 28.58124999877096784, 6.690598923241489970 ) ) ;
#3542=DIRECTION ( 'NONE',  ( 0.000000000000000000, 0.000000000000000000, 1.000000000000000000 ) ) ;
#3543=FACE_OUTER_BOUND ( 'NONE', #14525, .T. ) ;
#3544=LINE ( 'NONE', #9552, #2602 ) ;
#3545=CARTESIAN_POINT ( 'NONE',  ( 3.999999999999996447, -27.41874999877096641, 8.999999999999992895 ) ) ;
#3549=ORIENTED_EDGE ( 'NONE', *, *, #4219, .T. ) ;
#3554=CARTESIAN_POINT ( 'NONE',  ( 21.21320343559646915, 21.21320343559638744, 8.999999999999992895 ) ) ;
#3556=CARTESIAN_POINT ( 'NONE',  ( 3.756430356249996994, -28.62812499938548427, 8.999999999999992895 ) ) ;
#3558=CARTESIAN_POINT ( 'NONE',  ( 1.859271017917182139E-15, 28.93749999999999645, 12.99999999999999289 ) ) ;
#3559=ADVANCED_FACE ( 'NONE', ( #10014 ), #8070, .T. ) ;
#3561=EDGE_CURVE ( 'NONE', #11048, #8528, #9033, .T. ) ;
#3566=DIRECTION ( 'NONE',  ( 0.000000000000000000, -1.000000000000000000, 0.000000000000000000 ) ) ;
#3567=AXIS2_PLACEMENT_3D ( 'NONE', #14925, #8529, #12829 ) ;
#3568=CARTESIAN_POINT ( 'NONE',  ( 18.22334004483017011, 23.53573480074883761, 8.999999999999992895 ) ) ;
#3572=CARTESIAN_POINT ( 'NONE',  ( -1.999999999999995781, 26.50000000000000355, 5.535898384862237620 ) ) ;
#3574=CARTESIAN_POINT ( 'NONE',  ( 17.56042743746777646, 22.87282219338644751, 6.831223922626973533 ) ) ;
#3575=CARTESIAN_POINT ( 'NONE',  ( -1.859271017917182139E-15, -29.33124999877096428, 12.99999999999999289 ) ) ;
#3581=CARTESIAN_POINT ( 'NONE',  ( 0.5000000000000001110, 10.00000000000000000, 15.00000000000000178 ) ) ;
#3586=PLANE ( 'NONE',  #14418 ) ;
#3595=CARTESIAN_POINT ( 'NONE',  ( -3.756430356249996994, 29.41562499938548569, 8.999999999999992895 ) ) ;
#3599=CARTESIAN_POINT ( 'NONE',  ( 3.756430356250003211, 27.87812499938548427, 6.831223922626973533 ) ) ;
#3600=CARTESIAN_POINT ( 'NONE',  ( -3.472074595960224386, -29.79875828571876184, 6.996763648122163559 ) ) ;
#3601=CARTESIAN_POINT ( 'NONE',  ( 16.57281518405975262, 22.22966943355206126, 6.690598923241487306 ) ) ;
#3602=CARTESIAN_POINT ( 'NONE',  ( 23.03192121915348878, 17.71952646323466496, 11.16877607737301226 ) ) ;
#3605=CARTESIAN_POINT ( 'NONE',  ( 21.21320343559646915, 21.21320343559638744, 8.999999999999992895 ) ) ;
#3607=DIRECTION ( 'NONE',  ( 1.000000000000000000, 0.000000000000000000, -0.000000000000000000 ) ) ;
#3611=CARTESIAN_POINT ( 'NONE',  ( 1.999999999999995781, -26.95000000000000284, 5.535898384862237620 ) ) ;
#3613=EDGE_LOOP ( 'NONE', ( #2635, #3782, #17874, #5164, #7758, #2631, #11486, #4361 ) ) ;
#3617=CARTESIAN_POINT ( 'NONE',  ( -2.672651547586948120E-15, -29.52812499938548285, 13.33755215474602984 ) ) ;
#3630=CARTESIAN_POINT ( 'NONE',  ( -1.427366165835751044, -29.96717973704832261, 12.74788474329069921 ) ) ;
#3639=CARTESIAN_POINT ( 'NONE',  ( 1.071796769724492338, 28.90134618820330203, 12.99999999999999467 ) ) ;
#3644=ORIENTED_EDGE ( 'NONE', *, *, #8016, .T. ) ;
#3647=VERTEX_POINT ( 'NONE', #5836 ) ;
#3656=CARTESIAN_POINT ( 'NONE',  ( 3.735045420075836212E-15, 28.96562499938548640, 4.662447845253954171 ) ) ;
#3657=EDGE_CURVE ( 'NONE', #10871, #19250, #13823, .T. ) ;
#3658=CARTESIAN_POINT ( 'NONE',  ( -8.831537335106614961E-15, -26.63124999877096855, 12.99999999999999112 ) ) ;
#3661=CARTESIAN_POINT ( 'NONE',  ( -2.000000000000003997, -25.91874999877096997, 5.535898384862238508 ) ) ;
#3662=CARTESIAN_POINT ( 'NONE',  ( -3.469446951953614189E-15, -25.00000000000000000, 8.999999999999992895 ) ) ;
#3664=CARTESIAN_POINT ( 'NONE',  ( -4.000000000000001776, -25.80624999877096926, 11.30940107675849760 ) ) ;
#3665=CARTESIAN_POINT ( 'NONE',  ( 3.735045420075836212E-15, 28.06562499938548427, 4.662447845253954171 ) ) ;
#3675=( BOUNDED_CURVE ( )  B_SPLINE_CURVE ( 2, ( #2416, #8691, #10378, #4260, #8309, #18641, #20600, #4381, #2686 ),
 .UNSPECIFIED., .F., .F. ) 
 B_SPLINE_CURVE_WITH_KNOTS ( ( 3, 2, 2, 2, 3 ),
 ( 0.4750000000000000333, 0.4833333333333333370, 0.5000000000000000000, 0.5166666666666667185, 0.5250000000000000222 ),
 .UNSPECIFIED. ) 
 CURVE ( )  GEOMETRIC_REPRESENTATION_ITEM ( )  RATIONAL_B_SPLINE_CURVE ( ( 0.9330127018922194093, 0.9330127018922196314, 1.000000000000000000, 0.8660254037844387076, 1.000000000000000000, 0.8660254037844387076, 1.000000000000000000, 0.9330127018922194093, 0.9330127018922194093 ) ) 
 REPRESENTATION_ITEM ( '' )  );
#3678=CARTESIAN_POINT ( 'NONE',  ( -3.756430356250002323, -27.46562499938548640, 11.16877607737301226 ) ) ;
#3687=CARTESIAN_POINT ( 'NONE',  ( 18.64987758779700044, 21.30607496575630222, 12.25316411605951927 ) ) ;
#3688=CARTESIAN_POINT ( 'NONE',  ( -3.878215178125003604, -29.57031249969274356, 8.999999999999992895 ) ) ;
#3691=CARTESIAN_POINT ( 'NONE',  ( 2.000000000000000888, 28.97500000000000142, 12.46410161513774817 ) ) ;
#3694=CARTESIAN_POINT ( 'NONE',  ( 23.40315227927642283, 18.09075752335759901, 6.831223922626973533 ) ) ;
#3706=ORIENTED_EDGE ( 'NONE', *, *, #670, .F. ) ;
#3710=CARTESIAN_POINT ( 'NONE',  ( -3.469446951953614189E-15, -30.00000000000000355, 4.999999999999992006 ) ) ;
#3711=FACE_OUTER_BOUND ( 'NONE', #15993, .T. ) ;
#3713=DIRECTION ( 'NONE',  ( 0.000000000000000000, 1.000000000000000000, 0.000000000000000000 ) ) ;
#3715=( BOUNDED_SURFACE ( )  B_SPLINE_SURFACE ( 1, 2, ( 
 ( #17727, #8049, #23994, #4244, #23866, #13665, #25698, #12223, #203, #16030, #20190, #7779, #10246, #5951, #17988, #21636, #17850, #20058, #22024, #15759, #23724, #4106, #1906, #12084, #9991, #23606, #5812, #3861, #25821, #11834, #76, #2163, #19804, #9868, #7905, #18241, #13937, #21904, #24114, #3985, #11952, #323, #19922, #2023, #6197, #15641, #14453, #4372, #16664, #22413, #14570, #465, #24250, #12865, #22690, #22814, #24506, #22553, #6587, #22296, #20314, #14331, #2932, #4494, #18510, #20445, #6857, #8820, #20843, #12350, #10893, #24632, #18630, #2795, #2407, #18893, #8435, #10365, #8295, #12469, #14840, #10510, #4773, #24389, #2677, #6467, #10637, #715, #596, #16282, #8681, #16547, #4633, #6337, #18366, #12613, #2542, #8563, #6720, #16422, #20589, #12745, #4889, #14711, #20716, #10761, #16810, #18749, #839, #24774, #19012, #16933, #1095, #25405, #3307, #25166, #5024, #25024, #1223, #7247, #5542 ),
 ( #7491, #13005, #24902, #13254, #11283, #3065, #19264, #9340, #15483, #9204, #6980, #11033, #23452, #21369, #1366, #13525, #9070, #21495, #17194, #17324, #14961, #3183, #5403, #25287, #17055, #7115, #7368, #13140, #15345, #21225, #8959, #20986, #22937, #11150, #15101, #23315, #13390, #23076, #21105, #5160, #3572, #19131, #15227, #3447, #23193, #5278, #11544, #11421, #19395, #1487, #978, #9459, #17438, #1996, #25674, #25794, #11671, #9583, #24089, #8018, #8148, #9843, #7877, #17825, #7630, #5663, #25546, #14160, #7754, #3831, #5783, #18099, #20031, #6172, #15615, #22128, #9967, #3963, #14034, #23582, #4216, #19648, #13643, #19510, #15738, #177, #21748, #16003, #17958, #21611, #4078, #2135, #16127, #45, #17706, #17570, #23970, #5923, #11928, #6051, #1754, #22001, #12051, #1610, #10099, #23700, #3691, #9724, #13769, #11810, #19784, #1881, #15865, #23834, #13909, #21879, #19897, #10733, #8270, #24221, #18606 ) ),
 .UNSPECIFIED., .F., .F., .T. ) 
 B_SPLINE_SURFACE_WITH_KNOTS ( ( 2, 2 ),
 ( 3, 2, 2, 2, 2, 2, 2, 2, 2, 2, 2, 2, 2, 2, 2, 2, 2, 2, 2, 2, 2, 2, 2, 2, 2, 2, 2, 2, 2, 2, 2, 2, 2, 2, 2, 2, 2, 2, 2, 2, 2, 2, 2, 2, 2, 2, 2, 2, 2, 2, 2, 2, 2, 2, 2, 2, 2, 2, 2, 2, 3 ),
 ( 0.000000000000000000, 1.000000000000000000 ),
 ( 0.000000000000000000, 0.01666666666666666644, 0.03333333333333333287, 0.05000000000000000278, 0.06666666666666666574, 0.08333333333333332871, 0.1000000000000000056, 0.1166666666666666685, 0.1333333333333333315, 0.1499999999999999944, 0.1666666666666666574, 0.1833333333333333204, 0.2000000000000000111, 0.2166666666666666741, 0.2333333333333333370, 0.2500000000000000000, 0.2666666666666666630, 0.2833333333333333259, 0.2999999999999999889, 0.3166666666666666519, 0.3333333333333333148, 0.3499999999999999778, 0.3666666666666666408, 0.3833333333333333592, 0.4000000000000000222, 0.4166666666666666852, 0.4333333333333333481, 0.4500000000000000111, 0.4666666666666666741, 0.4833333333333333370, 0.5000000000000000000, 0.5166666666666667185, 0.5333333333333333259, 0.5500000000000000444, 0.5666666666666666519, 0.5833333333333333703, 0.5999999999999999778, 0.6166666666666666963, 0.6333333333333333037, 0.6500000000000000222, 0.6666666666666666297, 0.6833333333333333481, 0.6999999999999999556, 0.7166666666666666741, 0.7333333333333332815, 0.7500000000000000000, 0.7666666666666667185, 0.7833333333333333259, 0.8000000000000000444, 0.8166666666666666519, 0.8333333333333333703, 0.8499999999999999778, 0.8666666666666666963, 0.8833333333333333037, 0.9000000000000000222, 0.9166666666666666297, 0.9333333333333333481, 0.9499999999999999556, 0.9666666666666666741, 0.9833333333333332815, 1.000000000000000000 ),
 .UNSPECIFIED. ) 
 GEOMETRIC_REPRESENTATION_ITEM ( )  RATIONAL_B_SPLINE_SURFACE ( (
 ( 1.000000000000000000, 0.8660254037844387076, 1.000000000000000000, 0.8660254037844387076, 1.000000000000000000, 0.8660254037844387076, 1.000000000000000000, 0.8660254037844387076, 1.000000000000000000, 0.8660254037844387076, 1.000000000000000000, 0.8660254037844387076, 1.000000000000000000, 0.8660254037844387076, 1.000000000000000000, 0.8660254037844387076, 1.000000000000000000, 0.8660254037844387076, 1.000000000000000000, 0.8660254037844387076, 1.000000000000000000, 0.8660254037844387076, 1.000000000000000000, 0.8660254037844387076, 1.000000000000000000, 0.8660254037844387076, 1.000000000000000000, 0.8660254037844387076, 1.000000000000000000, 0.8660254037844387076, 1.000000000000000000, 0.8660254037844387076, 1.000000000000000000, 0.8660254037844387076, 1.000000000000000000, 0.8660254037844387076, 1.000000000000000000, 0.8660254037844387076, 1.000000000000000000, 0.8660254037844387076, 1.000000000000000000, 0.8660254037844387076, 1.000000000000000000, 0.8660254037844387076, 1.000000000000000000, 0.8660254037844387076, 1.000000000000000000, 0.8660254037844387076, 1.000000000000000000, 0.8660254037844387076, 1.000000000000000000, 0.8660254037844387076, 1.000000000000000000, 0.8660254037844387076, 1.000000000000000000, 0.8660254037844387076, 1.000000000000000000, 0.8660254037844387076, 1.000000000000000000, 0.8660254037844387076, 1.000000000000000000, 0.8660254037844387076, 1.000000000000000000, 0.8660254037844387076, 1.000000000000000000, 0.8660254037844387076, 1.000000000000000000, 0.8660254037844387076, 1.000000000000000000, 0.8660254037844387076, 1.000000000000000000, 0.8660254037844387076, 1.000000000000000000, 0.8660254037844387076, 1.000000000000000000, 0.8660254037844387076, 1.000000000000000000, 0.8660254037844387076, 1.000000000000000000, 0.8660254037844387076, 1.000000000000000000, 0.8660254037844387076, 1.000000000000000000, 0.8660254037844387076, 1.000000000000000000, 0.8660254037844387076, 1.000000000000000000, 0.8660254037844387076, 1.000000000000000000, 0.8660254037844387076, 1.000000000000000000, 0.8660254037844387076, 1.000000000000000000, 0.8660254037844387076, 1.000000000000000000, 0.8660254037844387076, 1.000000000000000000, 0.8660254037844387076, 1.000000000000000000, 0.8660254037844387076, 1.000000000000000000, 0.8660254037844387076, 1.000000000000000000, 0.8660254037844387076, 1.000000000000000000, 0.8660254037844387076, 1.000000000000000000, 0.8660254037844387076, 1.000000000000000000, 0.8660254037844387076, 1.000000000000000000, 0.8660254037844387076, 1.000000000000000000, 0.8660254037844387076, 1.000000000000000000, 0.8660254037844387076, 1.000000000000000000, 0.8660254037844387076, 1.000000000000000000, 0.8660254037844387076, 1.000000000000000000),
 ( 1.000000000000000000, 0.8660254037844387076, 1.000000000000000000, 0.8660254037844387076, 1.000000000000000000, 0.8660254037844387076, 1.000000000000000000, 0.8660254037844387076, 1.000000000000000000, 0.8660254037844387076, 1.000000000000000000, 0.8660254037844387076, 1.000000000000000000, 0.8660254037844387076, 1.000000000000000000, 0.8660254037844387076, 1.000000000000000000, 0.8660254037844387076, 1.000000000000000000, 0.8660254037844387076, 1.000000000000000000, 0.8660254037844387076, 1.000000000000000000, 0.8660254037844387076, 1.000000000000000000, 0.8660254037844387076, 1.000000000000000000, 0.8660254037844387076, 1.000000000000000000, 0.8660254037844387076, 1.000000000000000000, 0.8660254037844387076, 1.000000000000000000, 0.8660254037844387076, 1.000000000000000000, 0.8660254037844387076, 1.000000000000000000, 0.8660254037844387076, 1.000000000000000000, 0.8660254037844387076, 1.000000000000000000, 0.8660254037844387076, 1.000000000000000000, 0.8660254037844387076, 1.000000000000000000, 0.8660254037844387076, 1.000000000000000000, 0.8660254037844387076, 1.000000000000000000, 0.8660254037844387076, 1.000000000000000000, 0.8660254037844387076, 1.000000000000000000, 0.8660254037844387076, 1.000000000000000000, 0.8660254037844387076, 1.000000000000000000, 0.8660254037844387076, 1.000000000000000000, 0.8660254037844387076, 1.000000000000000000, 0.8660254037844387076, 1.000000000000000000, 0.8660254037844387076, 1.000000000000000000, 0.8660254037844387076, 1.000000000000000000, 0.8660254037844387076, 1.000000000000000000, 0.8660254037844387076, 1.000000000000000000, 0.8660254037844387076, 1.000000000000000000, 0.8660254037844387076, 1.000000000000000000, 0.8660254037844387076, 1.000000000000000000, 0.8660254037844387076, 1.000000000000000000, 0.8660254037844387076, 1.000000000000000000, 0.8660254037844387076, 1.000000000000000000, 0.8660254037844387076, 1.000000000000000000, 0.8660254037844387076, 1.000000000000000000, 0.8660254037844387076, 1.000000000000000000, 0.8660254037844387076, 1.000000000000000000, 0.8660254037844387076, 1.000000000000000000, 0.8660254037844387076, 1.000000000000000000, 0.8660254037844387076, 1.000000000000000000, 0.8660254037844387076, 1.000000000000000000, 0.8660254037844387076, 1.000000000000000000, 0.8660254037844387076, 1.000000000000000000, 0.8660254037844387076, 1.000000000000000000, 0.8660254037844387076, 1.000000000000000000, 0.8660254037844387076, 1.000000000000000000, 0.8660254037844387076, 1.000000000000000000, 0.8660254037844387076, 1.000000000000000000, 0.8660254037844387076, 1.000000000000000000, 0.8660254037844387076, 1.000000000000000000, 0.8660254037844387076, 1.000000000000000000, 0.8660254037844387076, 1.000000000000000000) ) ) 
 REPRESENTATION_ITEM ( '' )  SURFACE ( )  );
#3724=CARTESIAN_POINT ( 'NONE',  ( 22.38876845931909187, 16.73191420982663757, 11.30940107675849760 ) ) ;
#3725=CARTESIAN_POINT ( 'NONE',  ( 23.05843772344798381, 17.74604296752915999, 8.999999999999992895 ) ) ;
#3726=DIRECTION ( 'NONE',  ( 0.000000000000000000, 0.000000000000000000, 1.000000000000000000 ) ) ;
#3729=CARTESIAN_POINT ( 'NONE',  ( 23.00540471485899019, 17.69300995894016992, 6.831223922626973533 ) ) ;
#3730=AXIS2_PLACEMENT_3D ( 'NONE', #6727, #9441, #1591 ) ;
#3731=CARTESIAN_POINT ( 'NONE',  ( 18.03564233677035489, 18.03564233677029094, 4.999999999999992006 ) ) ;
#3734=CARTESIAN_POINT ( 'NONE',  ( -4.000000000000003553, -26.38750000000000284, 6.690598923241489970 ) ) ;
#3736=DIRECTION ( 'NONE',  ( -0.9659258262890673130, 0.2588190451025242922, 0.000000000000000000 ) ) ;
#3744=CARTESIAN_POINT ( 'NONE',  ( 1.859271017917182139E-15, 26.18124999877096570, 12.99999999999999289 ) ) ;
#3746=EDGE_LOOP ( 'NONE', ( #10352, #14248, #7120, #2218 ) ) ;
#3763=CARTESIAN_POINT ( 'NONE',  ( 15.94967733227004558, 21.60653158176235777, 11.30940107675849404 ) ) ;
#3764=ORIENTED_EDGE ( 'NONE', *, *, #24587, .T. ) ;
#3766=CARTESIAN_POINT ( 'NONE',  ( -1.878215178125000939, -28.32812499938548711, 12.25316411605952283 ) ) ;
#3776=CARTESIAN_POINT ( 'NONE',  ( 3.999999999999995559, -26.48124999877096641, 6.690598923241487306 ) ) ;
#3782=ORIENTED_EDGE ( 'NONE', *, *, #12659, .T. ) ;
#3793=CARTESIAN_POINT ( 'NONE',  ( -3.756430356249997882, 29.11562499938548143, 11.16877607737301226 ) ) ;
#3801=CARTESIAN_POINT ( 'NONE',  ( -3.752267015613588906E-15, -26.40624999877097068, 4.381197846482986158 ) ) ;
#3803=CARTESIAN_POINT ( 'NONE',  ( 2.672651547586948120E-15, 29.19062499938548783, 13.33755215474602984 ) ) ;
#3815=CARTESIAN_POINT ( 'NONE',  ( 1.878215178124998497, -28.70312499938548356, 12.25316411605951927 ) ) ;
#3823=ADVANCED_FACE ( 'NONE', ( #5665 ), #16130, .T. ) ;
#3825=LINE ( 'NONE', #5917, #14627 ) ;
#3826=CARTESIAN_POINT ( 'NONE',  ( 22.10157009459123856, 19.44537271663178757, 5.746835883940462963 ) ) ;
#3831=CARTESIAN_POINT ( 'NONE',  ( 2.620986760973688460E-15, 27.58750000000000213, 13.61880215351699874 ) ) ;
#3833=CARTESIAN_POINT ( 'NONE',  ( 20.00449278107117834, 20.00449278107111439, 13.33755215474603162 ) ) ;
#3842=CARTESIAN_POINT ( 'NONE',  ( -3.137519842735244810E-15, 26.46249999999999858, 4.999999999999991118 ) ) ;
#3856=CARTESIAN_POINT ( 'NONE',  ( -3.959305671612554781E-15, -30.00000000000000355, 12.99999999999999289 ) ) ;
#3859=AXIS2_PLACEMENT_3D ( 'NONE', #471, #14196, #24256 ) ;
#3861=CARTESIAN_POINT ( 'NONE',  ( 3.735045420075836212E-15, 26.15312499938548285, 4.662447845253954171 ) ) ;
#3863=CARTESIAN_POINT ( 'NONE',  ( 1.999999999999998224, -28.84374999877096712, 12.46410161513774639 ) ) ;
#3865=CARTESIAN_POINT ( 'NONE',  ( 16.94404624418269023, 22.60090049367499532, 11.30940107675849404 ) ) ;
#3866=CARTESIAN_POINT ( 'NONE',  ( 21.46517399152334704, 18.80897661356389605, 5.746835883940462963 ) ) ;
#3867=FACE_OUTER_BOUND ( 'NONE', #9675, .T. ) ;
#3868=FACE_OUTER_BOUND ( 'NONE', #8136, .T. ) ;
#3872=CARTESIAN_POINT ( 'NONE',  ( 20.81103645292755289, 15.15418220343510392, 6.690598923241489970 ) ) ;
#3876=CARTESIAN_POINT ( 'NONE',  ( -2.620986760973688460E-15, -25.78750000000000142, 13.61880215351699874 ) ) ;
#3880=CARTESIAN_POINT ( 'NONE',  ( 3.999999999999995559, -29.63124999877096855, 6.690598923241487306 ) ) ;
#3881=VERTEX_POINT ( 'NONE', #5512 ) ;
#3897=CARTESIAN_POINT ( 'NONE',  ( 1.071796769724492338, 28.50759618943233775, 12.99999999999999467 ) ) ;
#3899=CARTESIAN_POINT ( 'NONE',  ( 15.28000806814115720, 20.59240282405983535, 8.999999999999992895 ) ) ;
#3900=CARTESIAN_POINT ( 'NONE',  ( 18.03564233677035844, 18.03564233677029094, 4.381197846482986158 ) ) ;
#3905=CARTESIAN_POINT ( 'NONE',  ( 19.00660103559776459, 17.49085150774564923, 12.99999999999999112 ) ) ;
#3906=ADVANCED_FACE ( 'NONE', ( #19237 ), #5254, .F. ) ;
#3911=CARTESIAN_POINT ( 'NONE',  ( 2.000000000000000888, 27.11874999877096926, 12.46410161513774817 ) ) ;
#3926=CARTESIAN_POINT ( 'NONE',  ( 1.878215178125004048, 27.57812499938548711, 5.746835883940462963 ) ) ;
#3934=CARTESIAN_POINT ( 'NONE',  ( -2.000000000000000888, -29.36874999877096926, 12.46410161513774817 ) ) ;
#3936=CARTESIAN_POINT ( 'NONE',  ( -3.756430356249997882, 27.76562499938549067, 11.16877607737301226 ) ) ;
#3943=CARTESIAN_POINT ( 'NONE',  ( 1.071796769724494558, 28.24240381056766580, 4.999999999999992895 ) ) ;
#3949=CARTESIAN_POINT ( 'NONE',  ( -3.756430356250003655, -29.30312499938548498, 8.999999999999992895 ) ) ;
#3955=CARTESIAN_POINT ( 'NONE',  ( 2.672651547586948120E-15, 26.04062499938548925, 13.33755215474603162 ) ) ;
#3958=CARTESIAN_POINT ( 'NONE',  ( 17.90514199329621903, 23.21753674921489008, 8.999999999999992895 ) ) ;
#3963=CARTESIAN_POINT ( 'NONE',  ( -3.999999999999996003, 27.88750000000000284, 6.690598923241487306 ) ) ;
#3971=ORIENTED_EDGE ( 'NONE', *, *, #17605, .T. ) ;
#3973=CARTESIAN_POINT ( 'NONE',  ( 2.000000000000000888, 29.81874999877096855, 12.46410161513774817 ) ) ;
#3974=CARTESIAN_POINT ( 'NONE',  ( 17.61017577620189556, 19.12592530405386526, 4.999999999999991118 ) ) ;
#3975=CARTESIAN_POINT ( 'NONE',  ( 17.91631806831418317, 17.91631806831411566, 12.99999999999999289 ) ) ;
#3979=ORIENTED_EDGE ( 'NONE', *, *, #18962, .T. ) ;
#3983=CARTESIAN_POINT ( 'NONE',  ( 21.21320343559646915, 21.21320343559638744, 8.999999999999992895 ) ) ;
#3985=CARTESIAN_POINT ( 'NONE',  ( 3.735045420075836212E-15, 26.60312499938547859, 4.662447845253954171 ) ) ;
#3990=CARTESIAN_POINT ( 'NONE',  ( 18.59690834520624136, 21.42533546995235838, 5.535898384862237620 ) ) ;
#3991=CARTESIAN_POINT ( 'NONE',  ( 23.66831732222138740, 18.35592256630256003, 11.16877607737301226 ) ) ;
#3992=DIRECTION ( 'NONE',  ( 1.000000000000000000, 0.000000000000000000, 0.000000000000000000 ) ) ;
#3996=ORIENTED_EDGE ( 'NONE', *, *, #11092, .F. ) ;
#3998=CARTESIAN_POINT ( 'NONE',  ( -2.000000000000000888, -27.62500000000000000, 12.46410161513774817 ) ) ;
#4004=CARTESIAN_POINT ( 'NONE',  ( 3.834746474454188013E-15, 28.26249999999999929, 4.999999999999992006 ) ) ;
#4005=CARTESIAN_POINT ( 'NONE',  ( 2.000000000000003997, 26.36874999877096926, 5.535898384862238508 ) ) ;
#4006=ORIENTED_EDGE ( 'NONE', *, *, #13171, .T. ) ;
#4007=ORIENTED_EDGE ( 'NONE', *, *, #4182, .F. ) ;
#4008=CARTESIAN_POINT ( 'NONE',  ( -3.756430356250003211, -25.29062499938548569, 6.831223922626973533 ) ) ;
#4012=EDGE_CURVE ( 'NONE', #7798, #1111, #22606, .T. ) ;
#4018=CARTESIAN_POINT ( 'NONE',  ( 17.89864039878452928, 23.55549464827683437, 11.30940107675849404 ) ) ;
#4019=CARTESIAN_POINT ( 'NONE',  ( 20.45982030258741702, 15.14742554666860208, 6.831223922626973533 ) ) ;
#4020=CARTESIAN_POINT ( 'NONE',  ( 15.92316082797555055, 21.58001507746786274, 8.999999999999992895 ) ) ;
#4030=CARTESIAN_POINT ( 'NONE',  ( 4.000000000000003553, 25.88124999877096499, 6.690598923241489970 ) ) ;
#4037=ADVANCED_FACE ( 'NONE', ( #11917 ), #12827, .F. ) ;
#4044=CARTESIAN_POINT ( 'NONE',  ( -3.756430356249996994, 25.81562499938548427, 8.999999999999992895 ) ) ;
#4049=CARTESIAN_POINT ( 'NONE',  ( 1.999999999999998224, -25.69374999877097210, 12.46410161513774639 ) ) ;
#4051=CARTESIAN_POINT ( 'NONE',  ( -4.000000000000001776, -28.95624999877097494, 11.30940107675849760 ) ) ;
#4052=CARTESIAN_POINT ( 'NONE',  ( -1.878215178124998497, 28.25312499938548427, 12.25316411605951927 ) ) ;
#4058=CARTESIAN_POINT ( 'NONE',  ( 2.000000000000000888, 28.07500000000000284, 12.46410161513774817 ) ) ;
#4060=ORIENTED_EDGE ( 'NONE', *, *, #5161, .F. ) ;
#4064=ORIENTED_EDGE ( 'NONE', *, *, #20094, .T. ) ;
#4066=CARTESIAN_POINT ( 'NONE',  ( 22.70696651085303941, 17.05011226136058866, 11.30940107675849760 ) ) ;
#4068=ORIENTED_EDGE ( 'NONE', *, *, #7872, .F. ) ;
#4070=CARTESIAN_POINT ( 'NONE',  ( -3.756430356249996105, 25.89062499938548356, 6.831223922626973533 ) ) ;
#4073=CARTESIAN_POINT ( 'NONE',  ( 17.19146985159974150, 19.84766722955904683, 5.746835883940462963 ) ) ;
#4078=CARTESIAN_POINT ( 'NONE',  ( -3.999999999999996447, 28.37500000000000000, 8.999999999999992895 ) ) ;
#4081=CARTESIAN_POINT ( 'NONE',  ( 22.74023967191403628, 17.42784491599521601, 8.999999999999992895 ) ) ;
#4083=ORIENTED_EDGE ( 'NONE', *, *, #24665, .F. ) ;
#4089=CARTESIAN_POINT ( 'NONE',  ( 2.672651547586948120E-15, 26.04062499938548925, 13.33755215474602984 ) ) ;
#4092=VERTEX_POINT ( 'NONE', #4732 ) ;
#4095=CARTESIAN_POINT ( 'NONE',  ( -1.859271017917182139E-15, -25.78750000000000142, 12.99999999999999289 ) ) ;
#4097=DIRECTION ( 'NONE',  ( 0.000000000000000000, -1.000000000000000000, 0.000000000000000000 ) ) ;
#4099=( BOUNDED_CURVE ( )  B_SPLINE_CURVE ( 2, ( #3575, #17709, #11546, #21753, #19513, #15618, #9586, #50, #1758 ),
 .UNSPECIFIED., .F., .F. ) 
 B_SPLINE_CURVE_WITH_KNOTS ( ( 3, 2, 2, 2, 3 ),
 ( 0.8750000000000000000, 0.8833333333333333037, 0.9000000000000000222, 0.9166666666666666297, 0.9250000000000000444 ),
 .UNSPECIFIED. ) 
 CURVE ( )  GEOMETRIC_REPRESENTATION_ITEM ( )  RATIONAL_B_SPLINE_CURVE ( ( 0.9330127018922194093, 0.9330127018922194093, 1.000000000000000000, 0.8660254037844387076, 1.000000000000000000, 0.8660254037844387076, 1.000000000000000000, 0.9330127018922189652, 0.9330127018922194093 ) ) 
 REPRESENTATION_ITEM ( '' )  );
#4105=EDGE_CURVE ( 'NONE', #4358, #20170, #4738, .T. ) ;
#4106=CARTESIAN_POINT ( 'NONE',  ( 2.672651547586948120E-15, 25.92812499938548498, 13.33755215474602984 ) ) ;
#4115=CARTESIAN_POINT ( 'NONE',  ( -2.672651547586948120E-15, -25.47812499938548569, 13.33755215474603162 ) ) ;
#4116=CARTESIAN_POINT ( 'NONE',  ( 22.95237170627000367, 17.63997695035117985, 11.16877607737301403 ) ) ;
#4118=ORIENTED_EDGE ( 'NONE', *, *, #9299, .F. ) ;
#4120=CARTESIAN_POINT ( 'NONE',  ( -2.620986760973688460E-15, -28.93750000000000000, 13.61880215351699874 ) ) ;
#4122=VERTEX_POINT ( 'NONE', #796 ) ;
#4129=CARTESIAN_POINT ( 'NONE',  ( 3.756430356249997438, -25.51562499938548356, 11.16877607737301048 ) ) ;
#4131=LINE ( 'NONE', #8196, #11782 ) ;
#4136=ADVANCED_FACE ( 'NONE', ( #3023 ), #18976, .T. ) ;
#4141=CARTESIAN_POINT ( 'NONE',  ( 17.80583263288473717, 23.46268688237703870, 6.690598923241487306 ) ) ;
#4143=CARTESIAN_POINT ( 'NONE',  ( 19.63547142920491595, 16.80704430445866393, 12.46410161513774817 ) ) ;
#4144=DIRECTION ( 'NONE',  ( 0.000000000000000000, 0.000000000000000000, -1.000000000000000000 ) ) ;
#4146=CARTESIAN_POINT ( 'NONE',  ( 17.85886564147372724, 23.51571989096603232, 11.30940107675849404 ) ) ;
#4148=CARTESIAN_POINT ( 'NONE',  ( 1.071796769724485454, -27.11740381056766580, 12.99999999999999467 ) ) ;
#4158=CARTESIAN_POINT ( 'NONE',  ( 4.000000000000003553, 26.29374999877096997, 8.999999999999992895 ) ) ;
#4159=CARTESIAN_POINT ( 'NONE',  ( -3.756430356250003655, -25.14062499938548356, 8.999999999999992895 ) ) ;
#4175=CARTESIAN_POINT ( 'NONE',  ( 3.756430356250002323, 25.55312499938548143, 11.16877607737301226 ) ) ;
#4181=CARTESIAN_POINT ( 'NONE',  ( -3.063240906311874401, -29.84319947910909931, 11.57226653943512851 ) ) ;
#4182=EDGE_CURVE ( 'NONE', #2494, #5410, #20544, .T. ) ;
#4183=CARTESIAN_POINT ( 'NONE',  ( -3.999999999999995559, 28.73124999877096997, 6.690598923241487306 ) ) ;
#4184=CARTESIAN_POINT ( 'NONE',  ( -2.000000000000000888, -29.81874999877096855, 12.46410161513774817 ) ) ;
#4185=CARTESIAN_POINT ( 'NONE',  ( -1.878215178124998497, 29.15312499938548640, 12.25316411605951927 ) ) ;
#4204=CARTESIAN_POINT ( 'NONE',  ( 3.756430356250003655, 26.15312499938548640, 8.999999999999992895 ) ) ;
#4208=CARTESIAN_POINT ( 'NONE',  ( 16.89751483010538990, 22.20990958602406451, 11.16877607737301226 ) ) ;
#4209=ADVANCED_FACE ( 'NONE', ( #2758 ), #22504, .F. ) ;
#4216=CARTESIAN_POINT ( 'NONE',  ( -1.999999999999998224, 28.00000000000000000, 12.46410161513774639 ) ) ;
#4217=CARTESIAN_POINT ( 'NONE',  ( 3.756430356250003655, 29.19062499938548072, 8.999999999999992895 ) ) ;
#4219=EDGE_CURVE ( 'NONE', #1228, #12953, #25497, .T. ) ;
#4221=CARTESIAN_POINT ( 'NONE',  ( 3.834746474454188013E-15, 27.36250000000000426, 4.999999999999992006 ) ) ;
#4222=CARTESIAN_POINT ( 'NONE',  ( -3.834746474454188013E-15, -28.26249999999999929, 4.999999999999992006 ) ) ;
#4235=CARTESIAN_POINT ( 'NONE',  ( 21.21320343559646915, 21.21320343559638744, 8.999999999999992895 ) ) ;
#4237=CARTESIAN_POINT ( 'NONE',  ( 2.000000000000000888, 28.97500000000000142, 12.46410161513774817 ) ) ;
#4244=CARTESIAN_POINT ( 'NONE',  ( 3.735045420075836212E-15, 25.25312499938548783, 4.662447845253954171 ) ) ;
#4248=DIRECTION ( 'NONE',  ( 0.000000000000000000, 0.000000000000000000, -1.000000000000000000 ) ) ;
#4254=CARTESIAN_POINT ( 'NONE',  ( 20.26302869750798408, 20.26302869750790947, 4.999999999999992006 ) ) ;
#4255=CIRCLE ( 'NONE', #12189, 24.00000000000000355 ) ;
#4256=CARTESIAN_POINT ( 'NONE',  ( 3.756430356249996994, -25.81562499938548427, 8.999999999999992895 ) ) ;
#4260=CARTESIAN_POINT ( 'NONE',  ( 22.34899370200828983, 16.69213945251583908, 11.30940107675849760 ) ) ;
#4265=( BOUNDED_CURVE ( )  B_SPLINE_CURVE ( 2, ( #6860, #22197, #21937, #22816, #6107, #843, #2200, #11868, #11983 ),
 .UNSPECIFIED., .F., .F. ) 
 B_SPLINE_CURVE_WITH_KNOTS ( ( 3, 2, 2, 2, 3 ),
 ( 0.07500000000000001110, 0.08333333333333332871, 0.1000000000000000056, 0.1166666666666666685, 0.1249999999999999861 ),
 .UNSPECIFIED. ) 
 CURVE ( )  GEOMETRIC_REPRESENTATION_ITEM ( )  RATIONAL_B_SPLINE_CURVE ( ( 0.9330127018922192983, 0.9330127018922194093, 1.000000000000000000, 0.8660254037844387076, 1.000000000000000000, 0.8660254037844387076, 1.000000000000000000, 0.9330127018922195203, 0.9330127018922194093 ) ) 
 REPRESENTATION_ITEM ( '' )  );
#4271=CARTESIAN_POINT ( 'NONE',  ( -1.878215178125004048, -26.22812499938548569, 5.746835883940462963 ) ) ;
#4274=CARTESIAN_POINT ( 'NONE',  ( 1.626862140677534194E-14, 27.98124999877096997, 12.99999999999999289 ) ) ;
#4286=CARTESIAN_POINT ( 'NONE',  ( 15.88988766691455368, 21.20228242283322828, 6.831223922626973533 ) ) ;
#4287=CARTESIAN_POINT ( 'NONE',  ( 18.98139765660737055, 21.80982478135348757, 12.46410161513774639 ) ) ;
#4298=PLANE ( 'NONE',  #2990 ) ;
#4299=CARTESIAN_POINT ( 'NONE',  ( -3.999999999999996447, 25.61874999877096926, 8.999999999999992895 ) ) ;
#4300=CARTESIAN_POINT ( 'NONE',  ( 3.756430356249997882, -25.40312499938548285, 11.16877607737301226 ) ) ;
#4313=CARTESIAN_POINT ( 'NONE',  ( 3.756430356250004099, 26.97812499938548569, 6.831223922626973533 ) ) ;
#4319=CARTESIAN_POINT ( 'NONE',  ( -4.000000000000001776, -29.40624999877096357, 11.30940107675849760 ) ) ;
#4322=CARTESIAN_POINT ( 'NONE',  ( -1.071796769724493448, 29.57634618820329564, 4.999999999999995559 ) ) ;
#4323=CARTESIAN_POINT ( 'NONE',  ( -3.999999999999997335, 27.96250000000000213, 11.30940107675849404 ) ) ;
#4325=EDGE_LOOP ( 'NONE', ( #4981, #18199, #3226, #14200 ) ) ;
#4326=DIRECTION ( 'NONE',  ( 0.000000000000000000, -1.000000000000000000, 0.000000000000000000 ) ) ;
#4338=CARTESIAN_POINT ( 'NONE',  ( -3.756430356249996994, 27.27812499938548640, 8.999999999999992895 ) ) ;
#4342=CARTESIAN_POINT ( 'NONE',  ( 17.82786595466764012, 20.48406333262694190, 5.746835883940462963 ) ) ;
#4347=CARTESIAN_POINT ( 'NONE',  ( 3.735045420075836212E-15, 29.30312499938548498, 4.662447845253954171 ) ) ;
#4358=VERTEX_POINT ( 'NONE', #5118 ) ;
#4361=ORIENTED_EDGE ( 'NONE', *, *, #24990, .T. ) ;
#4362=CYLINDRICAL_SURFACE ( 'NONE', #20278, 4.000000000000000000 ) ;
#4370=CARTESIAN_POINT ( 'NONE',  ( 3.918924903856942255, 29.74337361029841276, 9.928636277907717300 ) ) ;
#4372=CARTESIAN_POINT ( 'NONE',  ( 3.756430356250002323, 26.90312499938548640, 11.16877607737301226 ) ) ;
#4376=FACE_OUTER_BOUND ( 'NONE', #15472, .T. ) ;
#4381=CARTESIAN_POINT ( 'NONE',  ( 20.37029720654250298, 18.85454767869038051, 4.999999999999992895 ) ) ;
#4390=ADVANCED_FACE ( 'NONE', ( #15189 ), #5238, .F. ) ;
#4391=CARTESIAN_POINT ( 'NONE',  ( -3.756430356250002323, -27.46562499938548640, 11.16877607737301403 ) ) ;
#4393=CARTESIAN_POINT ( 'NONE',  ( -2.000000000000000888, -28.91874999877096997, 12.46410161513774817 ) ) ;
#4400=( BOUNDED_CURVE ( )  B_SPLINE_CURVE ( 2, ( #14060, #12086, #9616, #9869, #205, #25573, #3863, #14191, #22161 ),
 .UNSPECIFIED., .F., .F. ) 
 B_SPLINE_CURVE_WITH_KNOTS ( ( 3, 2, 2, 2, 3 ),
 ( 0.7249999999999999778, 0.7333333333333332815, 0.7500000000000000000, 0.7666666666666667185, 0.7750000000000000222 ),
 .UNSPECIFIED. ) 
 CURVE ( )  GEOMETRIC_REPRESENTATION_ITEM ( )  RATIONAL_B_SPLINE_CURVE ( ( 0.9330127018922194093, 0.9330127018922194093, 1.000000000000000000, 0.8660254037844387076, 1.000000000000000000, 0.8660254037844387076, 1.000000000000000000, 0.9330127018922194093, 0.9330127018922194093 ) ) 
 REPRESENTATION_ITEM ( '' )  );
#4404=CARTESIAN_POINT ( 'NONE',  ( 19.87733689425031613, 21.39308642210229294, 4.999999999999995559 ) ) ;
#4405=CARTESIAN_POINT ( 'NONE',  ( 18.25213002337956780, 20.90832740133887313, 12.25316411605951927 ) ) ;
#4406=CARTESIAN_POINT ( 'NONE',  ( 23.03842281366518208, 17.38156856417272067, 6.690598923241489970 ) ) ;
#4410=( BOUNDED_CURVE ( )  B_SPLINE_CURVE ( 2, ( #18135, #1913, #18246, #9873, #14195, #11840, #25829, #23614, #5820 ),
 .UNSPECIFIED., .F., .F. ) 
 B_SPLINE_CURVE_WITH_KNOTS ( ( 3, 2, 2, 2, 3 ),
 ( 0.6750000000000000444, 0.6833333333333333481, 0.6999999999999999556, 0.7166666666666666741, 0.7249999999999999778 ),
 .UNSPECIFIED. ) 
 CURVE ( )  GEOMETRIC_REPRESENTATION_ITEM ( )  RATIONAL_B_SPLINE_CURVE ( ( 0.9330127018922194093, 0.9330127018922198534, 1.000000000000000000, 0.8660254037844387076, 1.000000000000000000, 0.8660254037844387076, 1.000000000000000000, 0.9330127018922194093, 0.9330127018922194093 ) ) 
 REPRESENTATION_ITEM ( '' )  );
#4412=CARTESIAN_POINT ( 'NONE',  ( -3.974466138550253103, 29.73560671006806899, 8.477544402765669673 ) ) ;
#4417=CARTESIAN_POINT ( 'NONE',  ( 0.000000000000000000, 0.000000000000000000, 0.000000000000000000 ) ) ;
#4419=CARTESIAN_POINT ( 'NONE',  ( -3.735045420075836212E-15, -26.15312499938548285, 4.662447845253954171 ) ) ;
#4424=CARTESIAN_POINT ( 'NONE',  ( -3.756430356250004099, -25.62812499938548072, 6.831223922626973533 ) ) ;
#4433=CARTESIAN_POINT ( 'NONE',  ( 3.756430356250002323, 29.71562499938548640, 11.16877607737301226 ) ) ;
#4441=CARTESIAN_POINT ( 'NONE',  ( -4.000000000000003553, -28.54374999877096997, 8.999999999999992895 ) ) ;
#4444=CARTESIAN_POINT ( 'NONE',  ( 3.999999999999997335, -25.26249999999999929, 11.30940107675849404 ) ) ;
#4446=CARTESIAN_POINT ( 'NONE',  ( -3.469446951953614189E-15, -30.00000000000000355, 4.999999999999992006 ) ) ;
#4449=CARTESIAN_POINT ( 'NONE',  ( -3.878215178125003604, -29.57031249969274356, 8.999999999999992895 ) ) ;
#4456=CARTESIAN_POINT ( 'NONE',  ( -1.071796769724494558, -27.79240381056766651, 4.999999999999992895 ) ) ;
#4457=ORIENTED_EDGE ( 'NONE', *, *, #9338, .F. ) ;
#4459=CARTESIAN_POINT ( 'NONE',  ( 3.756430356250002323, 25.66562499938548569, 11.16877607737301403 ) ) ;
#4463=CARTESIAN_POINT ( 'NONE',  ( 18.97034911358585418, 18.97034911358578668, 13.33755215474602984 ) ) ;
#4484=CARTESIAN_POINT ( 'NONE',  ( -3.469446951953614189E-15, -30.00000000000000355, 8.999999999999992895 ) ) ;
#4492=CARTESIAN_POINT ( 'NONE',  ( 4.000000000000003553, 29.73213749463701561, 8.999999999999992895 ) ) ;
#4494=CARTESIAN_POINT ( 'NONE',  ( 3.735045420075836212E-15, 27.50312499938548783, 4.662447845253954171 ) ) ;
#4497=CARTESIAN_POINT ( 'NONE',  ( 23.36987911821542951, 17.71302486872297166, 8.999999999999992895 ) ) ;
#4500=CARTESIAN_POINT ( 'NONE',  ( -1.999999999999995781, 29.14374999877096784, 5.535898384862237620 ) ) ;
#4505=CARTESIAN_POINT ( 'NONE',  ( -2.000000000000000888, -28.07500000000000284, 12.46410161513774817 ) ) ;
#4510=FACE_OUTER_BOUND ( 'NONE', #13924, .T. ) ;
#4514=CARTESIAN_POINT ( 'NONE',  ( 1.878215178124998497, -27.80312499938548498, 12.25316411605951927 ) ) ;
#4518=VECTOR ( 'NONE', #6281, 1000.000000000000000 ) ;
#4527=CARTESIAN_POINT ( 'NONE',  ( 4.000000000000003553, 25.44999999999999929, 8.999999999999992895 ) ) ;
#4528=CARTESIAN_POINT ( 'NONE',  ( 21.09621640565530853, 15.78382164973649537, 6.831223922626973533 ) ) ;
#4529=CARTESIAN_POINT ( 'NONE',  ( 17.80583263288473717, 23.46268688237704225, 6.690598923241487306 ) ) ;
#4532=CARTESIAN_POINT ( 'NONE',  ( 24.00000000000000355, 0.000000000000000000, 19.00000000000000000 ) ) ;
#4539=ORIENTED_EDGE ( 'NONE', *, *, #15626, .F. ) ;
#4542=CARTESIAN_POINT ( 'NONE',  ( -2.672651547586948120E-15, -26.82812499938548356, 13.33755215474602984 ) ) ;
#4543=CARTESIAN_POINT ( 'NONE',  ( 15.61822102945791002, 21.27507527895022221, 6.690598923241487306 ) ) ;
#4544=VERTEX_POINT ( 'NONE', #21836 ) ;
#4547=CARTESIAN_POINT ( 'NONE',  ( 3.756430356249995661, -26.67812499938548498, 6.831223922626973533 ) ) ;
#4557=CARTESIAN_POINT ( 'NONE',  ( 22.49925389301043666, 19.67082676826417398, 12.46410161513774817 ) ) ;
#4558=( BOUNDED_CURVE ( )  B_SPLINE_CURVE ( 2, ( #16190, #24427, #18666, #6504, #22456, #12518, #2592, #10554, #18553 ),
 .UNSPECIFIED., .F., .F. ) 
 B_SPLINE_CURVE_WITH_KNOTS ( ( 3, 2, 2, 2, 3 ),
 ( 0.3750000000000000000, 0.3833333333333333592, 0.4000000000000000222, 0.4166666666666666852, 0.4250000000000000444 ),
 .UNSPECIFIED. ) 
 CURVE ( )  GEOMETRIC_REPRESENTATION_ITEM ( )  RATIONAL_B_SPLINE_CURVE ( ( 0.9330127018922194093, 0.9330127018922194093, 1.000000000000000000, 0.8660254037844387076, 1.000000000000000000, 0.8660254037844387076, 1.000000000000000000, 0.9330127018922191873, 0.9330127018922194093 ) ) 
 REPRESENTATION_ITEM ( '' )  );
#4559=CARTESIAN_POINT ( 'NONE',  ( -3.756430356249995661, 25.77812499938548640, 6.831223922626973533 ) ) ;
#4565=DIRECTION ( 'NONE',  ( -0.7071067811865487940, -0.7071067811865463515, 0.000000000000000000 ) ) ;
#4568=CARTESIAN_POINT ( 'NONE',  ( -1.878215178125004048, -25.77812499938548640, 5.746835883940462963 ) ) ;
#4569=CARTESIAN_POINT ( 'NONE',  ( 3.756430356250004099, 29.34062499938548640, 6.831223922626973533 ) ) ;
#4571=ADVANCED_FACE ( 'NONE', ( #21698 ), #19740, .F. ) ;
#4573=AXIS2_PLACEMENT_3D ( 'NONE', #19906, #13651, #23980 ) ;
#4575=CARTESIAN_POINT ( 'NONE',  ( 1.774938052278379752, -29.94842879300231075, 5.405792698933810314 ) ) ;
#4576=ORIENTED_EDGE ( 'NONE', *, *, #5304, .F. ) ;
#4579=VERTEX_POINT ( 'NONE', #25749 ) ;
#4585=EDGE_LOOP ( 'NONE', ( #10350, #12454, #16439, #4083 ) ) ;
#4586=CARTESIAN_POINT ( 'NONE',  ( 3.469446951953614189E-15, 30.00000000000000355, 8.999999999999992895 ) ) ;
#4589=ORIENTED_EDGE ( 'NONE', *, *, #6278, .F. ) ;
#4591=CARTESIAN_POINT ( 'NONE',  ( 3.756430356250002323, 27.91562499938548569, 11.16877607737301403 ) ) ;
#4595=CARTESIAN_POINT ( 'NONE',  ( 15.62472262396960154, 20.93711737988828503, 11.16877607737301226 ) ) ;
#4596=CARTESIAN_POINT ( 'NONE',  ( -25.83240171513484285, -3.403349963601435935, 20.00001200000000168 ) ) ;
#4607=CARTESIAN_POINT ( 'NONE',  ( 4.000000000000003553, 27.68124999877096926, 6.690598923241489970 ) ) ;
#4608=ORIENTED_EDGE ( 'NONE', *, *, #21958, .T. ) ;
#4614=LINE ( 'NONE', #24373, #7874 ) ;
#4616=CARTESIAN_POINT ( 'NONE',  ( -1.999999999999995781, 26.05000000000000071, 5.535898384862237620 ) ) ;
#4624=CARTESIAN_POINT ( 'NONE',  ( 19.03001124868299243, 19.03001124868293559, 4.999999999999991118 ) ) ;
#4633=CARTESIAN_POINT ( 'NONE',  ( -1.878215178124998497, 28.59062499938548285, 12.25316411605951927 ) ) ;
#4635=AXIS2_PLACEMENT_3D ( 'NONE', #3983, #2158, #13661 ) ;
#4636=CARTESIAN_POINT ( 'NONE',  ( 17.58044234725058175, 23.23729659674288683, 11.30940107675849404 ) ) ;
#4639=CYLINDRICAL_SURFACE ( 'NONE', #3859, 26.00000000000000355 ) ;
#4641=CARTESIAN_POINT ( 'NONE',  ( -3.756430356250003655, -27.39062499938548356, 8.999999999999992895 ) ) ;
#4647=CARTESIAN_POINT ( 'NONE',  ( 1.999999999999998224, -29.35000000000000142, 12.46410161513774639 ) ) ;
#4649=VERTEX_POINT ( 'NONE', #2726 ) ;
#4650=VERTEX_POINT ( 'NONE', #12676 ) ;
#4655=CARTESIAN_POINT ( 'NONE',  ( -3.756430356250003211, -27.99062499938548498, 6.831223922626973533 ) ) ;
#4657=CARTESIAN_POINT ( 'NONE',  ( 19.92142043288880160, 18.40567090503668979, 12.99999999999999467 ) ) ;
#4663=DIRECTION ( 'NONE',  ( 0.000000000000000000, -1.000000000000000000, 0.000000000000000000 ) ) ;
#4668=CARTESIAN_POINT ( 'NONE',  ( 23.65168074169088186, 18.16705623898524280, 8.999999999999992895 ) ) ;
#4669=CARTESIAN_POINT ( 'NONE',  ( 16.58607343533794065, 22.24292768483024574, 11.30940107675849404 ) ) ;
#4671=CARTESIAN_POINT ( 'NONE',  ( 18.97034911358585418, 18.97034911358578668, 13.33755215474602984 ) ) ;
#4673=CARTESIAN_POINT ( 'NONE',  ( 19.78573162020705922, 19.78573162020699172, 13.61880215351699874 ) ) ;
#4680=( BOUNDED_CURVE ( )  B_SPLINE_CURVE ( 2, ( #13278, #13159, #23476, #21250, #19154, #3333, #9090, #10923, #3087 ),
 .UNSPECIFIED., .F., .F. ) 
 B_SPLINE_CURVE_WITH_KNOTS ( ( 3, 2, 2, 2, 3 ),
 ( 0.1749999999999999889, 0.1833333333333333204, 0.2000000000000000111, 0.2166666666666666741, 0.2250000000000000056 ),
 .UNSPECIFIED. ) 
 CURVE ( )  GEOMETRIC_REPRESENTATION_ITEM ( )  RATIONAL_B_SPLINE_CURVE ( ( 0.9330127018922194093, 0.9330127018922194093, 1.000000000000000000, 0.8660254037844387076, 1.000000000000000000, 0.8660254037844387076, 1.000000000000000000, 0.9330127018922194093, 0.9330127018922194093 ) ) 
 REPRESENTATION_ITEM ( '' )  );
#4681=CARTESIAN_POINT ( 'NONE',  ( 18.01575495898401513, 18.01575495898394763, 13.33755215474603162 ) ) ;
#4683=ORIENTED_EDGE ( 'NONE', *, *, #25754, .F. ) ;
#4685=CARTESIAN_POINT ( 'NONE',  ( -3.999999999999996447, 28.76874999877096784, 8.999999999999992895 ) ) ;
#4686=CARTESIAN_POINT ( 'NONE',  ( -1.878215178125004048, -27.46562499938548640, 5.746835883940462963 ) ) ;
#4690=CARTESIAN_POINT ( 'NONE',  ( 18.83113746560522728, 18.83113746560514912, 12.99999999999999112 ) ) ;
#4694=CARTESIAN_POINT ( 'NONE',  ( -3.756430356250003655, -26.94062499938548427, 8.999999999999992895 ) ) ;
#4697=ORIENTED_EDGE ( 'NONE', *, *, #21958, .F. ) ;
#4701=DIRECTION ( 'NONE',  ( -0.7071067811865487940, -0.7071067811865463515, 0.000000000000000000 ) ) ;
#4702=B_SPLINE_CURVE_WITH_KNOTS ( 'NONE', 3,
 ( #9619, #1124, #19164, #23224, #3210, #21137, #3600, #11180, #17598, #15376, #1257, #25576, #9241, #13286, #13669, #21400, #21262, #17466 ),
 .UNSPECIFIED., .F., .F.,
 ( 4, 2, 2, 2, 2, 2, 2, 2, 4 ),
 ( 0.01878087663358380885, 0.01956282976579720376, 0.02034478289801060213, 0.02112673603022399704, 0.02190868916243739195, 0.02269064229465078686, 0.02347259542686418177, 0.02425454855907758014, 0.02503650169129097505 ),
 .UNSPECIFIED. ) ;
#4708=CARTESIAN_POINT ( 'NONE',  ( 2.672651547586948120E-15, 29.52812499938548285, 13.33755215474602984 ) ) ;
#4713=UNCERTAINTY_MEASURE_WITH_UNIT (LENGTH_MEASURE( 1.000000000000000082E-05 ), #3407, 'distance_accuracy_value', 'NONE');
#4715=CARTESIAN_POINT ( 'NONE',  ( 18.34500155353947903, 21.17342867828559605, 12.46410161513774639 ) ) ;
#4718=CARTESIAN_POINT ( 'NONE',  ( -2.672651547586948120E-15, -26.04062499938548925, 13.33755215474602984 ) ) ;
#4719=CARTESIAN_POINT ( 'NONE',  ( -1.878215178124998497, 29.60312499938548569, 12.25316411605951927 ) ) ;
#4722=CARTESIAN_POINT ( 'NONE',  ( 2.644755406393140440, -29.88376691385261097, 5.987824696368042154 ) ) ;
#4732=CARTESIAN_POINT ( 'NONE',  ( -5.577813053751546416E-15, -25.33750000000000213, 12.99999999999999289 ) ) ;
#4737=CARTESIAN_POINT ( 'NONE',  ( 3.756430356250002323, 28.36562499938548854, 11.16877607737301403 ) ) ;
#4738=( BOUNDED_CURVE ( )  B_SPLINE_CURVE ( 2, ( #10994, #1059, #16762, #12430, #22774, #555, #16897, #4456, #24861 ),
 .UNSPECIFIED., .F., .F. ) 
 B_SPLINE_CURVE_WITH_KNOTS ( ( 3, 2, 2, 2, 3 ),
 ( 0.5750000000000000666, 0.5833333333333333703, 0.5999999999999999778, 0.6166666666666666963, 0.6250000000000000000 ),
 .UNSPECIFIED. ) 
 CURVE ( )  GEOMETRIC_REPRESENTATION_ITEM ( )  RATIONAL_B_SPLINE_CURVE ( ( 0.9330127018922194093, 0.9330127018922198534, 1.000000000000000000, 0.8660254037844387076, 1.000000000000000000, 0.8660254037844387076, 1.000000000000000000, 0.9330127018922194093, 0.9330127018922194093 ) ) 
 REPRESENTATION_ITEM ( '' )  );
#4742=CARTESIAN_POINT ( 'NONE',  ( 18.78246010926947918, 21.43865748722877740, 5.746835883940462963 ) ) ;
#4746=EDGE_CURVE ( 'NONE', #16889, #17313, #10902, .T. ) ;
#4757=ORIENTED_EDGE ( 'NONE', *, *, #20870, .F. ) ;
#4763=CARTESIAN_POINT ( 'NONE',  ( 3.756430356249995661, -25.89062499938548356, 6.831223922626973533 ) ) ;
#4772=CARTESIAN_POINT ( 'NONE',  ( 18.25440349763447756, 18.25440349763440295, 4.662447845253954171 ) ) ;
#4773=CARTESIAN_POINT ( 'NONE',  ( 1.878215178125000939, 28.21562499938548640, 12.25316411605952283 ) ) ;
#4776=CARTESIAN_POINT ( 'NONE',  ( 2.000000000000000888, 26.66874999877096641, 12.46410161513774817 ) ) ;
#4780=CARTESIAN_POINT ( 'NONE',  ( 1.878215178124995832, -27.99062499938548143, 5.746835883940462963 ) ) ;
#4783=CARTESIAN_POINT ( 'NONE',  ( 2.665892461326258456, 29.88220662469441891, 11.99618178085344056 ) ) ;
#4786=ORIENTED_EDGE ( 'NONE', *, *, #18920, .T. ) ;
#4788=PRODUCT_DEFINITION_FORMATION_WITH_SPECIFIED_SOURCE ( 'ANY', '', #7169, .NOT_KNOWN. ) ;
#4791=CARTESIAN_POINT ( 'NONE',  ( -3.756430356250003655, -27.05312499938548498, 8.999999999999992895 ) ) ;
#4798=CARTESIAN_POINT ( 'NONE',  ( 23.35662086519912606, 17.69976661570667176, 6.690598923241489970 ) ) ;
#4803=CARTESIAN_POINT ( 'NONE',  ( 18.83113746560522728, 18.83113746560514912, 12.99999999999999112 ) ) ;
#4804=CARTESIAN_POINT ( 'NONE',  ( 22.02429405596265610, 16.71189930004383584, 8.999999999999992895 ) ) ;
#4805=CARTESIAN_POINT ( 'NONE',  ( 15.33304107673014727, 20.64543583264882542, 6.831223922626973533 ) ) ;
#4810=CARTESIAN_POINT ( 'NONE',  ( 21.09621640565530853, 15.78382164973649537, 6.831223922626973533 ) ) ;
#4814=CARTESIAN_POINT ( 'NONE',  ( -1.999999999999998224, 27.94374999877096855, 12.46410161513774639 ) ) ;
#4815=CARTESIAN_POINT ( 'NONE',  ( 1.878215178124995832, -25.74062499938548498, 5.746835883940462963 ) ) ;
#4817=CARTESIAN_POINT ( 'NONE',  ( 15.89664432368105551, 21.55349857317336415, 6.690598923241487306 ) ) ;
#4818=EDGE_LOOP ( 'NONE', ( #15663, #3549, #7018, #4869 ) ) ;
#4819=CARTESIAN_POINT ( 'NONE',  ( -3.756430356250003655, -25.59062499938548285, 8.999999999999992895 ) ) ;
#4826=LINE ( 'NONE', #909, #1352 ) ;
#4827=CARTESIAN_POINT ( 'NONE',  ( -1.878215178124995832, 27.54062499938548214, 5.746835883940462963 ) ) ;
#4830=CARTESIAN_POINT ( 'NONE',  ( 3.999999999999996447, -28.82499999999999929, 8.999999999999992895 ) ) ;
#4833=CARTESIAN_POINT ( 'NONE',  ( 19.78573162020706988, 19.78573162020698462, 12.99999999999999289 ) ) ;
#4837=CARTESIAN_POINT ( 'NONE',  ( -3.756430356250002323, -27.01562499938548356, 11.16877607737301226 ) ) ;
#4844=CARTESIAN_POINT ( 'NONE',  ( -3.959305671612554781E-15, -30.00000000000000355, 12.99999999999999289 ) ) ;
#4848=MANIFOLD_SOLID_BREP ( 'CirPattern3', #1707 ) ;
#4855=CARTESIAN_POINT ( 'NONE',  ( 3.756430356250003655, 29.30312499938548498, 8.999999999999992895 ) ) ;
#4859=CARTESIAN_POINT ( 'NONE',  ( 3.756430356250004099, 25.74062499938548143, 6.831223922626973533 ) ) ;
#4860=CARTESIAN_POINT ( 'NONE',  ( -6.741346781237202102, -25.16843286583315731, 20.00001200000000168 ) ) ;
#4865=CARTESIAN_POINT ( 'NONE',  ( 3.369928719974892281E-15, 25.11250000000000426, 4.999999999999992006 ) ) ;
#4869=ORIENTED_EDGE ( 'NONE', *, *, #4942, .F. ) ;
#4875=LINE ( 'NONE', #7231, #16229 ) ;
#4877=CARTESIAN_POINT ( 'NONE',  ( 1.878215178124998497, -25.55312499938548854, 12.25316411605951927 ) ) ;
#4886=CARTESIAN_POINT ( 'NONE',  ( -1.999999999999995781, 28.24374999877096570, 5.535898384862237620 ) ) ;
#4887=CARTESIAN_POINT ( 'NONE',  ( 18.33167953626305646, 20.98787691422236179, 12.25316411605951927 ) ) ;
#4889=CARTESIAN_POINT ( 'NONE',  ( -3.756430356249996994, 28.96562499938548285, 8.999999999999992895 ) ) ;
#4892=EDGE_CURVE ( 'NONE', #9493, #2390, #19718, .T. ) ;
#4894=CARTESIAN_POINT ( 'NONE',  ( 26.00000000000000355, 1.592040838891558898E-15, 20.00000599999999906 ) ) ;
#4896=CARTESIAN_POINT ( 'NONE',  ( -1.878215178125004048, -26.56562499938548427, 5.746835883940462963 ) ) ;
#4907=CARTESIAN_POINT ( 'NONE',  ( -3.756430356250002323, -29.26562499938548356, 11.16877607737301403 ) ) ;
#4915=CARTESIAN_POINT ( 'NONE',  ( 16.59933168835424411, 22.25618593784655630, 8.999999999999992895 ) ) ;
#4919=CARTESIAN_POINT ( 'NONE',  ( 23.32360276639294128, 18.01120801047411746, 6.831223922626973533 ) ) ;
#4920=CARTESIAN_POINT ( 'NONE',  ( 19.04989862646933929, 19.04989862646927534, 13.33755215474602984 ) ) ;
#4921=CARTESIAN_POINT ( 'NONE',  ( -3.469446951953614189E-15, -30.00000000000000355, 8.999999999999992895 ) ) ;
#4922=EDGE_CURVE ( 'NONE', #22272, #17660, #22392, .T. ) ;
#4926=CARTESIAN_POINT ( 'NONE',  ( 18.57032807491351178, 21.22652545287281356, 12.25316411605951927 ) ) ;
#4927=DIRECTION ( 'NONE',  ( 0.000000000000000000, -1.000000000000000000, 0.000000000000000000 ) ) ;
#4931=CARTESIAN_POINT ( 'NONE',  ( -1.999999999999998224, 27.04374999877096641, 12.46410161513774639 ) ) ;
#4932=CARTESIAN_POINT ( 'NONE',  ( 3.756430356249997882, -28.10312499938548569, 11.16877607737301226 ) ) ;
#4938=CARTESIAN_POINT ( 'NONE',  ( -3.756430356250004099, -28.77812499938548285, 6.831223922626973533 ) ) ;
#4942=EDGE_CURVE ( 'NONE', #10748, #19630, #7511, .T. ) ;
#4945=( BOUNDED_CURVE ( )  B_SPLINE_CURVE ( 2, ( #19190, #17119, #13458, #15670, #1288, #21292, #9650, #19572, #23638 ),
 .UNSPECIFIED., .F., .T. ) 
 B_SPLINE_CURVE_WITH_KNOTS ( ( 3, 2, 2, 2, 3 ),
 ( 0.4750000000000000333, 0.4833333333333333370, 0.5000000000000000000, 0.5166666666666667185, 0.5250000000000000222 ),
 .UNSPECIFIED. ) 
 CURVE ( )  GEOMETRIC_REPRESENTATION_ITEM ( )  RATIONAL_B_SPLINE_CURVE ( ( 0.9330127018922194093, 0.9330127018922196314, 1.000000000000000000, 0.8660254037844387076, 1.000000000000000000, 0.8660254037844387076, 1.000000000000000000, 0.9330127018922194093, 0.9330127018922194093 ) ) 
 REPRESENTATION_ITEM ( '' )  );
#4951=CARTESIAN_POINT ( 'NONE',  ( 3.735045420075836212E-15, 27.95312499938548001, 4.662447845253954171 ) ) ;
#4958=CARTESIAN_POINT ( 'NONE',  ( 0.000000000000000000, 0.000000000000000000, 19.59999999999999787 ) ) ;
#4961=CARTESIAN_POINT ( 'NONE',  ( 1.878215178124998497, -27.80312499938548498, 12.25316411605951927 ) ) ;
#4966=CARTESIAN_POINT ( 'NONE',  ( 21.69050051289738690, 18.86207338815112067, 5.535898384862238508 ) ) ;
#4967=AXIS2_PLACEMENT_3D ( 'NONE', #23011, #14780, #6798 ) ;
#4975=VECTOR ( 'NONE', #6768, 1000.000000000000000 ) ;
#4978=ORIENTED_EDGE ( 'NONE', *, *, #25575, .T. ) ;
#4981=ORIENTED_EDGE ( 'NONE', *, *, #3174, .F. ) ;
#4982=EDGE_CURVE ( 'NONE', #933, #9293, #9862, .T. ) ;
#4984=CARTESIAN_POINT ( 'NONE',  ( 2.672651547586948120E-15, 29.64062499938548356, 13.33755215474603162 ) ) ;
#4987=CARTESIAN_POINT ( 'NONE',  ( 23.00540471485899374, 17.69300995894016992, 6.831223922626973533 ) ) ;
#4989=CARTESIAN_POINT ( 'NONE',  ( 2.672651547586948120E-15, 26.04062499938548925, 13.33755215474602984 ) ) ;
#4994=CYLINDRICAL_SURFACE ( 'NONE', #14141, 4.000000000000000000 ) ;
#4999=DIRECTION ( 'NONE',  ( 0.000000000000000000, 0.000000000000000000, 1.000000000000000000 ) ) ;
#5000=ORIENTED_EDGE ( 'NONE', *, *, #17756, .F. ) ;
#5001=ADVANCED_FACE ( 'NONE', ( #25813 ), #15505, .F. ) ;
#5005=CYLINDRICAL_SURFACE ( 'NONE', #3282, 4.000000000000000000 ) ;
#5006=ORIENTED_EDGE ( 'NONE', *, *, #9966, .T. ) ;
#5007=CARTESIAN_POINT ( 'NONE',  ( 3.756430356249996994, -25.47812499938548569, 8.999999999999992895 ) ) ;
#5013=CARTESIAN_POINT ( 'NONE',  ( 1.999999999999995781, -29.19999999999999929, 5.535898384862237620 ) ) ;
#5018=CARTESIAN_POINT ( 'NONE',  ( 18.09882730716638832, 19.61457683501836868, 12.99999999999999289 ) ) ;
#5019=CARTESIAN_POINT ( 'NONE',  ( 17.37708538166121386, 20.03328275962052274, 12.25316411605951927 ) ) ;
#5024=CARTESIAN_POINT ( 'NONE',  ( -1.878215178124998497, 29.49062499938548498, 12.25316411605951927 ) ) ;
#5026=CARTESIAN_POINT ( 'NONE',  ( 15.65123912826409480, 20.96363388418276941, 6.831223922626973533 ) ) ;
#5027=LINE ( 'NONE', #17057, #15360 ) ;
#5028=ORIENTED_EDGE ( 'NONE', *, *, #25754, .T. ) ;
#5030=CARTESIAN_POINT ( 'NONE',  ( 3.756430356249997438, -27.20312499938548356, 11.16877607737301048 ) ) ;
#5037=ORIENTED_EDGE ( 'NONE', *, *, #6083, .F. ) ;
#5038=PLANE ( 'NONE',  #9151 ) ;
#5039=AXIS2_PLACEMENT_3D ( 'NONE', #10832, #9133, #658 ) ;
#5055=CARTESIAN_POINT ( 'NONE',  ( 3.959305671612554781E-15, 30.00000000000000355, 12.99999999999999289 ) ) ;
#5060=CARTESIAN_POINT ( 'NONE',  ( 3.756430356250003655, 27.39062499938548356, 8.999999999999992895 ) ) ;
#5062=CARTESIAN_POINT ( 'NONE',  ( 21.91595456452976975, 19.25975718657032232, 12.25316411605952283 ) ) ;
#5063=CARTESIAN_POINT ( 'NONE',  ( 17.58921741601718125, 20.24541479397648303, 5.746835883940462963 ) ) ;
#5068=CARTESIAN_POINT ( 'NONE',  ( 22.05081056025715114, 16.73841580433833442, 6.831223922626973533 ) ) ;
#5072=CARTESIAN_POINT ( 'NONE',  ( 3.752267015613588906E-15, 27.75624999877096855, 4.381197846482986158 ) ) ;
#5073=CARTESIAN_POINT ( 'NONE',  ( -2.620986760973688460E-15, -25.33750000000000568, 13.61880215351699874 ) ) ;
#5079=CARTESIAN_POINT ( 'NONE',  ( -3.756430356250002323, -29.15312499938548640, 11.16877607737301226 ) ) ;
#5082=CARTESIAN_POINT ( 'NONE',  ( 19.26289903505010415, 22.99947435013303476, 12.01472878375390962 ) ) ;
#5091=CARTESIAN_POINT ( 'NONE',  ( -1.071796769724491227, -27.28615380933863577, 4.999999999999989342 ) ) ;
#5092=CARTESIAN_POINT ( 'NONE',  ( 1.878215178125004048, 29.26562499938548356, 5.746835883940462963 ) ) ;
#5099=CARTESIAN_POINT ( 'NONE',  ( 15.28676472490765548, 20.94361897439997122, 8.999999999999992895 ) ) ;
#5100=CARTESIAN_POINT ( 'NONE',  ( 3.756430356249996994, -26.82812499938548711, 8.999999999999992895 ) ) ;
#5103=CIRCLE ( 'NONE', #18047, 0.7500000000000001110 ) ;
#5105=ADVANCED_FACE ( 'NONE', ( #18121 ), #16656, .F. ) ;
#5112=( BOUNDED_CURVE ( )  B_SPLINE_CURVE ( 2, ( #8075, #10656, #4393, #6487, #10149, #2567, #6222, #16565, #20337 ),
 .UNSPECIFIED., .F., .F. ) 
 B_SPLINE_CURVE_WITH_KNOTS ( ( 3, 2, 2, 2, 3 ),
 ( 0.7750000000000000222, 0.7833333333333333259, 0.8000000000000000444, 0.8166666666666666519, 0.8250000000000000666 ),
 .UNSPECIFIED. ) 
 CURVE ( )  GEOMETRIC_REPRESENTATION_ITEM ( )  RATIONAL_B_SPLINE_CURVE ( ( 0.9330127018922194093, 0.9330127018922194093, 1.000000000000000000, 0.8660254037844387076, 1.000000000000000000, 0.8660254037844387076, 1.000000000000000000, 0.9330127018922189652, 0.9330127018922194093 ) ) 
 REPRESENTATION_ITEM ( '' )  );
#5114=ORIENTED_EDGE ( 'NONE', *, *, #15479, .F. ) ;
#5118=CARTESIAN_POINT ( 'NONE',  ( -1.626862140677534194E-14, -27.58750000000000213, 12.99999999999999289 ) ) ;
#5119=( BOUNDED_CURVE ( )  B_SPLINE_CURVE ( 2, ( #22478, #6650, #4557, #12541, #10965 ),
 .UNSPECIFIED., .F., .F. ) 
 B_SPLINE_CURVE_WITH_KNOTS ( ( 3, 2, 3 ),
 ( 0.9749999999999999778, 0.9833333333333332815, 0.9889400238386636399 ),
 .UNSPECIFIED. ) 
 CURVE ( )  GEOMETRIC_REPRESENTATION_ITEM ( )  RATIONAL_B_SPLINE_CURVE ( ( 0.9330127018922194093, 0.9330127018922194093, 1.000000000000000000, 0.9549307542065648136, 0.9401842259098239785 ) ) 
 REPRESENTATION_ITEM ( '' )  );
#5122=CARTESIAN_POINT ( 'NONE',  ( 3.735045420075836212E-15, 28.06562499938548427, 4.662447845253954171 ) ) ;
#5127=CARTESIAN_POINT ( 'NONE',  ( 23.61528431363239022, 18.30288955771356640, 8.999999999999992895 ) ) ;
#5128=CARTESIAN_POINT ( 'NONE',  ( 1.878215178125000939, 26.52812499938548285, 12.25316411605952283 ) ) ;
#5129=CARTESIAN_POINT ( 'NONE',  ( 8.831537335106614961E-15, 26.23749999999999716, 12.99999999999999112 ) ) ;
#5131=ADVANCED_FACE ( 'NONE', ( #590 ), #10357, .F. ) ;
#5134=CARTESIAN_POINT ( 'NONE',  ( -1.071796769724492338, -29.40759618943233278, 12.99999999999999467 ) ) ;
#5137=CARTESIAN_POINT ( 'NONE',  ( 3.137519842735244810E-15, -26.46249999999999858, 4.999999999999991118 ) ) ;
#5147=FACE_OUTER_BOUND ( 'NONE', #22184, .T. ) ;
#5154=CARTESIAN_POINT ( 'NONE',  ( 3.999999999999996447, -27.47499999999999787, 8.999999999999992895 ) ) ;
#5157=CARTESIAN_POINT ( 'NONE',  ( 1.626862140677534194E-14, 28.43124999877096570, 12.99999999999999289 ) ) ;
#5158=CARTESIAN_POINT ( 'NONE',  ( 16.60583328286593741, 21.91822803878461201, 6.831223922626973533 ) ) ;
#5160=CARTESIAN_POINT ( 'NONE',  ( 3.752267015613588906E-15, 26.46250000000000213, 4.381197846482986158 ) ) ;
#5161=EDGE_CURVE ( 'NONE', #2304, #22503, #2533, .T. ) ;
#5162=CARTESIAN_POINT ( 'NONE',  ( 17.37708538166121386, 20.03328275962052274, 12.25316411605951927 ) ) ;
#5164=ORIENTED_EDGE ( 'NONE', *, *, #10213, .T. ) ;
#5169=CARTESIAN_POINT ( 'NONE',  ( 3.756430356249997438, -28.55312499938548498, 11.16877607737301048 ) ) ;
#5180=CARTESIAN_POINT ( 'NONE',  ( 3.756430356249996994, -29.52812499938548640, 8.999999999999992895 ) ) ;
#5181=CARTESIAN_POINT ( 'NONE',  ( 20.78451994863305430, 15.12766569914060888, 8.999999999999992895 ) ) ;
#5184=DIRECTION ( 'NONE',  ( -0.7071067811865487940, -0.7071067811865463515, 0.000000000000000000 ) ) ;
#5187=CARTESIAN_POINT ( 'NONE',  ( -3.999999999999996447, 27.02500000000000213, 8.999999999999992895 ) ) ;
#5188=CARTESIAN_POINT ( 'NONE',  ( 4.000000000000003553, 29.69687499938548569, 8.999999999999992895 ) ) ;
#5189=CARTESIAN_POINT ( 'NONE',  ( -3.756430356249997438, 27.20312499938548356, 11.16877607737301048 ) ) ;
#5191=CARTESIAN_POINT ( 'NONE',  ( 16.47558800164659587, 19.30401512639272354, 12.46410161513774639 ) ) ;
#5192=CARTESIAN_POINT ( 'NONE',  ( 19.61779375967526562, 22.44622088442137908, 12.46410161513774639 ) ) ;
#5193=CARTESIAN_POINT ( 'NONE',  ( 20.14370442905180525, 20.14370442905174130, 12.99999999999999289 ) ) ;
#5196=CARTESIAN_POINT ( 'NONE',  ( 22.36900861179109867, 17.05661385587227841, 6.831223922626973533 ) ) ;
#5198=EDGE_LOOP ( 'NONE', ( #22280, #15953, #21884, #8577 ) ) ;
#5200=CARTESIAN_POINT ( 'NONE',  ( -3.999999999999997335, 28.35624999877096997, 11.30940107675849404 ) ) ;
#5201=CARTESIAN_POINT ( 'NONE',  ( -3.756430356250003655, -28.29062499938548569, 8.999999999999992895 ) ) ;
#5208=CARTESIAN_POINT ( 'NONE',  ( 3.756430356249995661, -29.37812499938548427, 6.831223922626973533 ) ) ;
#5211=CARTESIAN_POINT ( 'NONE',  ( 21.21320343559646915, 21.21320343559638744, 12.99999999999999289 ) ) ;
#5223=CARTESIAN_POINT ( 'NONE',  ( 3.756430356249996994, -28.62812499938548427, 8.999999999999992895 ) ) ;
#5226=CARTESIAN_POINT ( 'NONE',  ( -1.071796769724488563, 26.16115380933863221, 12.99999999999999289 ) ) ;
#5228=CARTESIAN_POINT ( 'NONE',  ( 23.07819757097597702, 17.42134332148352627, 6.690598923241489970 ) ) ;
#5234=ORIENTED_EDGE ( 'NONE', *, *, #2985, .T. ) ;
#5238=CYLINDRICAL_SURFACE ( 'NONE', #13046, 4.000000000000000000 ) ;
#5240=CARTESIAN_POINT ( 'NONE',  ( 23.36385188462466900, 18.81896140916762050, 11.39306173506717457 ) ) ;
#5244=CARTESIAN_POINT ( 'NONE',  ( 20.08404229395466700, 20.08404229395459240, 4.662447845253954171 ) ) ;
#5245=CARTESIAN_POINT ( 'NONE',  ( 3.756430356250003655, 26.60312499938548569, 8.999999999999992895 ) ) ;
#5250=CARTESIAN_POINT ( 'NONE',  ( 18.55271417138208179, 18.55271417138200363, 12.99999999999999112 ) ) ;
#5251=CARTESIAN_POINT ( 'NONE',  ( 17.54066758993977970, 23.19752183943208479, 11.30940107675849404 ) ) ;
#5253=CARTESIAN_POINT ( 'NONE',  ( -3.752267015613588906E-15, -25.95624999877096784, 4.381197846482986158 ) ) ;
#5254=CYLINDRICAL_SURFACE ( 'NONE', #24252, 4.000000000000000000 ) ;
#5258=CARTESIAN_POINT ( 'NONE',  ( -25.99307600111999150, 0.5999999999999998668, 19.00000000000000000 ) ) ;
#5260=( BOUNDED_CURVE ( )  B_SPLINE_CURVE ( 2, ( #2575, #8983, #18540, #10398, #10790, #20477, #22842, #22320, #22443 ),
 .UNSPECIFIED., .F., .F. ) 
 B_SPLINE_CURVE_WITH_KNOTS ( ( 3, 2, 2, 2, 3 ),
 ( 0.7249999999999999778, 0.7333333333333332815, 0.7500000000000000000, 0.7666666666666667185, 0.7750000000000000222 ),
 .UNSPECIFIED. ) 
 CURVE ( )  GEOMETRIC_REPRESENTATION_ITEM ( )  RATIONAL_B_SPLINE_CURVE ( ( 0.9330127018922194093, 0.9330127018922194093, 1.000000000000000000, 0.8660254037844387076, 1.000000000000000000, 0.8660254037844387076, 1.000000000000000000, 0.9330127018922194093, 0.9330127018922194093 ) ) 
 REPRESENTATION_ITEM ( '' )  );
#5266=ORIENTED_EDGE ( 'NONE', *, *, #10513, .F. ) ;
#5267=LINE ( 'NONE', #23304, #13034 ) ;
#5275=CARTESIAN_POINT ( 'NONE',  ( 21.49396397007274473, 16.18156921415393157, 6.831223922626973533 ) ) ;
#5277=CIRCLE ( 'NONE', #696, 30.00000000000000355 ) ;
#5278=CARTESIAN_POINT ( 'NONE',  ( 2.620986760973688460E-15, 26.68750000000000000, 13.61880215351699874 ) ) ;
#5279=CARTESIAN_POINT ( 'NONE',  ( 19.04989862646933929, 19.04989862646927534, 13.33755215474603162 ) ) ;
#5281=EDGE_LOOP ( 'NONE', ( #17331, #17655, #14630, #10678 ) ) ;
#5288=DIRECTION ( 'NONE',  ( -0.000000000000000000, -1.000000000000000000, -0.000000000000000000 ) ) ;
#5294=VERTEX_POINT ( 'NONE', #19121 ) ;
#5295=CARTESIAN_POINT ( 'NONE',  ( -3.735045420075836212E-15, -28.51562499938548356, 4.662447845253954171 ) ) ;
#5304=EDGE_CURVE ( 'NONE', #7798, #8491, #22805, .T. ) ;
#5305=CARTESIAN_POINT ( 'NONE',  ( -3.999999999999997335, 27.06250000000000000, 11.30940107675849404 ) ) ;
#5306=CARTESIAN_POINT ( 'NONE',  ( -8.831537335106614961E-15, -27.13750000000000284, 12.99999999999999112 ) ) ;
#5307=CARTESIAN_POINT ( 'NONE',  ( 2.672651547586948120E-15, 25.92812499938548498, 13.33755215474603162 ) ) ;
#5308=DIRECTION ( 'NONE',  ( 1.000000000000000000, 0.000000000000000000, -0.000000000000000000 ) ) ;
#5309=CARTESIAN_POINT ( 'NONE',  ( 20.24314131972164432, 20.24314131972156972, 13.33755215474602984 ) ) ;
#5310=CARTESIAN_POINT ( 'NONE',  ( 20.82877788845545552, 18.17258051049600454, 5.746835883940462963 ) ) ;
#5313=CARTESIAN_POINT ( 'NONE',  ( 22.43212701321220948, 19.92128553278266878, 5.406171146378998316 ) ) ;
#5314=CARTESIAN_POINT ( 'NONE',  ( 17.61573392031167273, 20.27193129827097806, 12.25316411605951927 ) ) ;
#5317=CARTESIAN_POINT ( 'NONE',  ( 18.71181319714904490, 18.71181319714897384, 4.999999999999991118 ) ) ;
#5318=CARTESIAN_POINT ( 'NONE',  ( -1.878215178124998497, 26.45312499938548711, 12.25316411605951927 ) ) ;
#5319=CARTESIAN_POINT ( 'NONE',  ( -2.672651547586948120E-15, -29.52812499938548285, 13.33755215474602984 ) ) ;
#5320=CARTESIAN_POINT ( 'NONE',  ( -3.999999999999997335, 25.26249999999999929, 11.30940107675849404 ) ) ;
#5323=CARTESIAN_POINT ( 'NONE',  ( -19.58805710660148236, 17.18149551509898743, 20.00001200000000523 ) ) ;
#5324=CARTESIAN_POINT ( 'NONE',  ( 3.756430356249995661, -27.12812499938548427, 6.831223922626973533 ) ) ;
#5327=CARTESIAN_POINT ( 'NONE',  ( 18.29810693902837571, 23.77355554533980353, 10.03836643961819419 ) ) ;
#5334=EDGE_CURVE ( 'NONE', #7544, #17713, #21548, .T. ) ;
#5342=CARTESIAN_POINT ( 'NONE',  ( 3.878215178125003604, 25.07031249969274356, 8.999999999999992895 ) ) ;
#5344=CARTESIAN_POINT ( 'NONE',  ( -3.756430356250002323, -28.36562499938548854, 11.16877607737301226 ) ) ;
#5345=CARTESIAN_POINT ( 'NONE',  ( 17.22246953840583572, 22.87932378789814436, 11.30940107675849404 ) ) ;
#5346=DIRECTION ( 'NONE',  ( -0.7071067811865487940, -0.7071067811865463515, 0.000000000000000000 ) ) ;
#5348=ORIENTED_EDGE ( 'NONE', *, *, #25333, .F. ) ;
#5351=CARTESIAN_POINT ( 'NONE',  ( 18.23451611984813425, 18.23451611984805609, 12.99999999999999112 ) ) ;
#5364=( NAMED_UNIT ( * ) SI_UNIT ( $, .STERADIAN. ) SOLID_ANGLE_UNIT ( ) );
#5365=CARTESIAN_POINT ( 'NONE',  ( -3.756430356249997882, 25.96562499938548640, 11.16877607737301226 ) ) ;
#5368=CYLINDRICAL_SURFACE ( 'NONE', #16811, 4.000000000000000000 ) ;
#5372=DIRECTION ( 'NONE',  ( 0.000000000000000000, 0.000000000000000000, -1.000000000000000000 ) ) ;
#5374=CARTESIAN_POINT ( 'NONE',  ( -2.620986760973688460E-15, -27.98124999877096997, 13.61880215351699874 ) ) ;
#5377=VECTOR ( 'NONE', #25776, 999.9999999999998863 ) ;
#5378=CARTESIAN_POINT ( 'NONE',  ( 1.999999999999998224, -26.64999999999999858, 12.46410161513774639 ) ) ;
#5379=DIRECTION ( 'NONE',  ( 0.000000000000000000, 0.000000000000000000, 1.000000000000000000 ) ) ;
#5381=CARTESIAN_POINT ( 'NONE',  ( -4.000000000000003553, -25.93750000000000000, 6.690598923241489970 ) ) ;
#5386=CARTESIAN_POINT ( 'NONE',  ( 0.000000000000000000, 0.000000000000000000, 17.00000000000000000 ) ) ;
#5388=CARTESIAN_POINT ( 'NONE',  ( 3.756430356249995661, -27.24062499938548498, 6.831223922626973533 ) ) ;
#5389=ORIENTED_EDGE ( 'NONE', *, *, #11775, .T. ) ;
#5398=CARTESIAN_POINT ( 'NONE',  ( 18.19682354053567153, 23.50921829645433903, 6.831223922626973533 ) ) ;
#5403=CARTESIAN_POINT ( 'NONE',  ( 2.000000000000000888, 25.82499999999999929, 12.46410161513774817 ) ) ;
#5404=( BOUNDED_CURVE ( )  B_SPLINE_CURVE ( 2, ( #17429, #7743, #25277, #15470, #1739, #17180, #19118, #5527, #3558 ),
 .UNSPECIFIED., .F., .F. ) 
 B_SPLINE_CURVE_WITH_KNOTS ( ( 3, 2, 2, 2, 3 ),
 ( 0.8250000000000000666, 0.8333333333333333703, 0.8499999999999999778, 0.8666666666666666963, 0.8750000000000000000 ),
 .UNSPECIFIED. ) 
 CURVE ( )  GEOMETRIC_REPRESENTATION_ITEM ( )  RATIONAL_B_SPLINE_CURVE ( ( 0.9330127018922194093, 0.9330127018922198534, 1.000000000000000000, 0.8660254037844387076, 1.000000000000000000, 0.8660254037844387076, 1.000000000000000000, 0.9330127018922194093, 0.9330127018922194093 ) ) 
 REPRESENTATION_ITEM ( '' )  );
#5406=CARTESIAN_POINT ( 'NONE',  ( 22.42204162038009230, 17.10964686446126848, 8.999999999999992895 ) ) ;
#5410=VERTEX_POINT ( 'NONE', #5878 ) ;
#5413=CARTESIAN_POINT ( 'NONE',  ( 21.21320343559646915, 21.21320343559638744, 12.99999999999999289 ) ) ;
#5416=CARTESIAN_POINT ( 'NONE',  ( 19.50730832598392084, 19.50730832598383913, 12.99999999999999289 ) ) ;
#5422=CYLINDRICAL_SURFACE ( 'NONE', #7466, 4.000000000000000000 ) ;
#5434=CARTESIAN_POINT ( 'NONE',  ( 3.756430356250002323, 26.00312499938548427, 11.16877607737301403 ) ) ;
#5436=AXIS2_PLACEMENT_3D ( 'NONE', #18762, #1234, #21114 ) ;
#5438=CARTESIAN_POINT ( 'NONE',  ( 18.17030703624117294, 23.48270179215984754, 11.16877607737301226 ) ) ;
#5439=CARTESIAN_POINT ( 'NONE',  ( 19.52719570377026415, 19.52719570377018599, 4.662447845253954171 ) ) ;
#5444=CARTESIAN_POINT ( 'NONE',  ( 17.29753586877772520, 19.95373324673703408, 12.25316411605951927 ) ) ;
#5446=ORIENTED_EDGE ( 'NONE', *, *, #10740, .T. ) ;
#5448=CARTESIAN_POINT ( 'NONE',  ( -1.878215178124998497, 25.55312499938548854, 12.25316411605951927 ) ) ;
#5449=CARTESIAN_POINT ( 'NONE',  ( 1.878215178124995832, -28.44062499938548427, 5.746835883940462963 ) ) ;
#5454=CARTESIAN_POINT ( 'NONE',  ( 24.67207871933482011, 8.377607117416825844, 20.00001200000000168 ) ) ;
#5455=CARTESIAN_POINT ( 'NONE',  ( -1.878215178125004048, -28.81562499938548427, 5.746835883940462963 ) ) ;
#5456=ORIENTED_EDGE ( 'NONE', *, *, #12069, .F. ) ;
#5460=VECTOR ( 'NONE', #7378, 1000.000000000000000 ) ;
#5465=DIRECTION ( 'NONE',  ( -1.000000000000000000, -0.000000000000000000, -0.000000000000000000 ) ) ;
#5467=DIRECTION ( 'NONE',  ( -0.7071067811865487940, -0.7071067811865463515, 0.000000000000000000 ) ) ;
#5469=CARTESIAN_POINT ( 'NONE',  ( -3.999999999999995559, 26.53750000000000142, 6.690598923241487306 ) ) ;
#5472=CARTESIAN_POINT ( 'NONE',  ( 17.28434138175965273, 20.11276850650576975, 5.535898384862237620 ) ) ;
#5474=DIRECTION ( 'NONE',  ( -0.000000000000000000, -0.000000000000000000, -1.000000000000000000 ) ) ;
#5477=CARTESIAN_POINT ( 'NONE',  ( 21.11597625318330884, 15.45912200369085632, 11.30940107675849760 ) ) ;
#5480=CARTESIAN_POINT ( 'NONE',  ( 1.071796769724495668, 27.15759618943233633, 12.99999999999999112 ) ) ;
#5481=CARTESIAN_POINT ( 'NONE',  ( 1.773386257881301553, -29.94852044693267246, 12.59496732558994125 ) ) ;
#5484=ORIENTED_EDGE ( 'NONE', *, *, #8353, .T. ) ;
#5485=ADVANCED_FACE ( 'NONE', ( #7973 ), #6010, .F. ) ;
#5486=AXIS2_PLACEMENT_3D ( 'NONE', #4417, #8344, #16332 ) ;
#5488=VERTEX_POINT ( 'NONE', #18432 ) ;
#5489=ORIENTED_EDGE ( 'NONE', *, *, #7117, .T. ) ;
#5496=EDGE_CURVE ( 'NONE', #14487, #19630, #18118, .T. ) ;
#5497=CIRCLE ( 'NONE', #8006, 0.5000000000000001110 ) ;
#5502=CARTESIAN_POINT ( 'NONE',  ( 3.756430356250002323, 27.46562499938548640, 11.16877607737301226 ) ) ;
#5504=CARTESIAN_POINT ( 'NONE',  ( -4.000000000000003553, -26.78124999877097068, 6.690598923241489970 ) ) ;
#5509=CARTESIAN_POINT ( 'NONE',  ( -1.626862140677534194E-14, -28.43124999877096570, 12.99999999999999289 ) ) ;
#5510=CARTESIAN_POINT ( 'NONE',  ( 3.999999999999997335, -27.00624999877096499, 11.30940107675849404 ) ) ;
#5512=CARTESIAN_POINT ( 'NONE',  ( 4.000000000000003553, 29.89374999877096784, 8.999999999999992895 ) ) ;
#5513=DIRECTION ( 'NONE',  ( 0.000000000000000000, 0.000000000000000000, -1.000000000000000000 ) ) ;
#5514=DIRECTION ( 'NONE',  ( -0.7071067811865487940, -0.7071067811865463515, 0.000000000000000000 ) ) ;
#5522=( BOUNDED_CURVE ( )  B_SPLINE_CURVE ( 2, ( #2149, #14438, #4616, #10351, #449, #8420, #14173, #12598, #16408 ),
 .UNSPECIFIED., .F., .F. ) 
 B_SPLINE_CURVE_WITH_KNOTS ( ( 3, 2, 2, 2, 3 ),
 ( 0.2250000000000000056, 0.2333333333333333370, 0.2500000000000000000, 0.2666666666666666630, 0.2750000000000000222 ),
 .UNSPECIFIED. ) 
 CURVE ( )  GEOMETRIC_REPRESENTATION_ITEM ( )  RATIONAL_B_SPLINE_CURVE ( ( 0.9330127018922194093, 0.9330127018922194093, 1.000000000000000000, 0.8660254037844387076, 1.000000000000000000, 0.8660254037844387076, 1.000000000000000000, 0.9330127018922191873, 0.9330127018922194093 ) ) 
 REPRESENTATION_ITEM ( '' )  );
#5524=CARTESIAN_POINT ( 'NONE',  ( -3.756430356250004099, -27.99062499938548498, 6.831223922626973533 ) ) ;
#5527=CARTESIAN_POINT ( 'NONE',  ( -1.071796769724488563, 28.91740381056766651, 12.99999999999999289 ) ) ;
#5533=EDGE_CURVE ( 'NONE', #8698, #2116, #2610, .T. ) ;
#5536=CARTESIAN_POINT ( 'NONE',  ( -1.859271017917182139E-15, -29.33124999877096428, 12.99999999999999289 ) ) ;
#5537=LINE ( 'NONE', #13521, #9575 ) ;
#5538=CARTESIAN_POINT ( 'NONE',  ( 17.87862548900172044, 23.19102024492039504, 6.831223922626973533 ) ) ;
#5539=DIRECTION ( 'NONE',  ( -0.7071067811865487940, -0.7071067811865463515, 0.000000000000000000 ) ) ;
#5541=EDGE_CURVE ( 'NONE', #10843, #11941, #22552, .T. ) ;
#5542=CARTESIAN_POINT ( 'NONE',  ( 3.756430356250003655, 29.64062499938548356, 8.999999999999992895 ) ) ;
#5543=CARTESIAN_POINT ( 'NONE',  ( 20.32269083260512588, 20.32269083260505482, 13.33755215474603162 ) ) ;
#5546=ORIENTED_EDGE ( 'NONE', *, *, #2336, .F. ) ;
#5548=ORIENTED_EDGE ( 'NONE', *, *, #2666, .F. ) ;
#5553=CARTESIAN_POINT ( 'NONE',  ( -1.071796769724490117, 27.32634618820330630, 4.999999999999992895 ) ) ;
#5565=( BOUNDED_CURVE ( )  B_SPLINE_CURVE ( 2, ( #24882, #11132, #6960, #14939, #3044, #19110, #18994, #1077, #7224 ),
 .UNSPECIFIED., .F., .F. ) 
 B_SPLINE_CURVE_WITH_KNOTS ( ( 3, 2, 2, 2, 3 ),
 ( 0.07500000000000001110, 0.08333333333333332871, 0.1000000000000000056, 0.1166666666666666685, 0.1250000000000000000 ),
 .UNSPECIFIED. ) 
 CURVE ( )  GEOMETRIC_REPRESENTATION_ITEM ( )  RATIONAL_B_SPLINE_CURVE ( ( 0.9330127018922192983, 0.9330127018922194093, 1.000000000000000000, 0.8660254037844387076, 1.000000000000000000, 0.8660254037844387076, 1.000000000000000000, 0.9330127018922194093, 0.9330127018922194093 ) ) 
 REPRESENTATION_ITEM ( '' )  );
#5568=CARTESIAN_POINT ( 'NONE',  ( -3.756430356249996994, 27.61562499938548143, 8.999999999999992895 ) ) ;
#5572=CARTESIAN_POINT ( 'NONE',  ( 3.756430356250002323, 27.80312499938548143, 11.16877607737301403 ) ) ;
#5573=CARTESIAN_POINT ( 'NONE',  ( 0.000000000000000000, 0.000000000000000000, 19.00000000000000000 ) ) ;
#5574=CARTESIAN_POINT ( 'NONE',  ( 16.25461713252580509, 21.91147138201811373, 6.690598923241487306 ) ) ;
#5575=CARTESIAN_POINT ( 'NONE',  ( 19.36809667800328683, 19.36809667800321932, 13.33755215474602984 ) ) ;
#5579=CARTESIAN_POINT ( 'NONE',  ( 23.27056975780394765, 17.95817500188513094, 11.16877607737301403 ) ) ;
#5581=VERTEX_POINT ( 'NONE', #14892 ) ;
#5583=CARTESIAN_POINT ( 'NONE',  ( -2.000000000000000888, -25.82499999999999929, 12.46410161513774817 ) ) ;
#5587=LINE ( 'NONE', #19558, #15941 ) ;
#5589=CARTESIAN_POINT ( 'NONE',  ( -26.00000000000000000, 1.701696020694461131, 20.00001199999999812 ) ) ;
#5600=FACE_OUTER_BOUND ( 'NONE', #10710, .T. ) ;
#5601=CARTESIAN_POINT ( 'NONE',  ( 24.00000000000000355, 0.000000000000000000, 17.00000000000000000 ) ) ;
#5603=CARTESIAN_POINT ( 'NONE',  ( -0.5788183228083377818, -29.99578766836522092, 12.96878440844335678 ) ) ;
#5604=DIRECTION ( 'NONE',  ( 0.000000000000000000, 1.000000000000000000, 0.000000000000000000 ) ) ;
#5605=CARTESIAN_POINT ( 'NONE',  ( 17.39040739893763643, 20.21883452368375700, 12.46410161513774639 ) ) ;
#5606=VERTEX_POINT ( 'NONE', #12536 ) ;
#5610=CARTESIAN_POINT ( 'NONE',  ( -1.071796769724487230, 25.97634618820330132, 4.999999999999992006 ) ) ;
#5613=CARTESIAN_POINT ( 'NONE',  ( 1.999999999999995781, -26.89374999877097139, 5.535898384862237620 ) ) ;
#5618=ORIENTED_EDGE ( 'NONE', *, *, #21163, .T. ) ;
#5619=ORIENTED_EDGE ( 'NONE', *, *, #13131, .T. ) ;
#5622=CARTESIAN_POINT ( 'NONE',  ( 17.91631806831418317, 17.91631806831411922, 12.99999999999999289 ) ) ;
#5625=CARTESIAN_POINT ( 'NONE',  ( 1.999999999999998224, -29.35000000000000142, 12.46410161513774639 ) ) ;
#5631=CARTESIAN_POINT ( 'NONE',  ( -3.756430356249995661, 28.59062499938548640, 6.831223922626973533 ) ) ;
#5635=CARTESIAN_POINT ( 'NONE',  ( -4.000000000000003553, -25.88124999877096855, 6.690598923241489970 ) ) ;
#5636=DIRECTION ( 'NONE',  ( 0.000000000000000000, 1.000000000000000000, 0.000000000000000000 ) ) ;
#5639=CARTESIAN_POINT ( 'NONE',  ( 3.999999999999996447, -26.96874999877096712, 8.999999999999992895 ) ) ;
#5640=CARTESIAN_POINT ( 'NONE',  ( 1.878215178125000939, 27.87812499938548427, 12.25316411605952283 ) ) ;
#5647=EDGE_LOOP ( 'NONE', ( #11883, #20433, #19088, #5546, #2141, #19856 ) ) ;
#5649=EDGE_LOOP ( 'NONE', ( #18202, #7829, #9947, #14142 ) ) ;
#5650=CARTESIAN_POINT ( 'NONE',  ( 1.878215178124995832, -27.20312499938548711, 5.746835883940462963 ) ) ;
#5652=CARTESIAN_POINT ( 'NONE',  ( -0.7500000000000001110, 9.184850993605150903E-17, 15.00000000000000178 ) ) ;
#5656=EDGE_CURVE ( 'NONE', #2042, #13143, #11430, .T. ) ;
#5659=FACE_OUTER_BOUND ( 'NONE', #15278, .T. ) ;
#5660=CARTESIAN_POINT ( 'NONE',  ( 19.15823811790222919, 16.50204073994278531, 5.746835883940462963 ) ) ;
#5661=PLANE ( 'NONE',  #18398 ) ;
#5663=CARTESIAN_POINT ( 'NONE',  ( -3.999999999999996003, 27.43750000000000000, 6.690598923241487306 ) ) ;
#5665=FACE_OUTER_BOUND ( 'NONE', #18463, .T. ) ;
#5666=CARTESIAN_POINT ( 'NONE',  ( 23.37663577498192780, 18.06424101906310753, 8.999999999999992895 ) ) ;
#5672=FACE_OUTER_BOUND ( 'NONE', #1917, .T. ) ;
#5675=ORIENTED_EDGE ( 'NONE', *, *, #3328, .T. ) ;
#5678=ORIENTED_EDGE ( 'NONE', *, *, #18962, .F. ) ;
#5691=CARTESIAN_POINT ( 'NONE',  ( 22.09708691207964293, 16.44023266258718863, 8.999999999999992895 ) ) ;
#5692=CARTESIAN_POINT ( 'NONE',  ( 19.28627369086489551, 21.94247106882419729, 12.25316411605951927 ) ) ;
#5696=CARTESIAN_POINT ( 'NONE',  ( 20.87953742278953229, 20.87953742278946123, 13.33755215474603162 ) ) ;
#5700=CARTESIAN_POINT ( 'NONE',  ( 3.999999999999996447, -26.12500000000000355, 8.999999999999992895 ) ) ;
#5704=DIRECTION ( 'NONE',  ( 0.000000000000000000, 1.000000000000000000, 0.000000000000000000 ) ) ;
#5705=CARTESIAN_POINT ( 'NONE',  ( 25.83240171513483929, 3.403349963601484340, 20.00001200000000168 ) ) ;
#5713=AXIS2_PLACEMENT_3D ( 'NONE', #22301, #20449, #12355 ) ;
#5716=CARTESIAN_POINT ( 'NONE',  ( -3.834746474454188013E-15, -27.75624999877096855, 4.999999999999992006 ) ) ;
#5717=CARTESIAN_POINT ( 'NONE',  ( 22.07057040778514789, 16.41371615829269359, 11.30940107675849760 ) ) ;
#5721=CARTESIAN_POINT ( 'NONE',  ( 17.70860545047158396, 20.53703257521770453, 12.46410161513774639 ) ) ;
#5724=CARTESIAN_POINT ( 'NONE',  ( 1.878215178124995832, -29.00312499938548427, 5.746835883940462963 ) ) ;
#5746=CARTESIAN_POINT ( 'NONE',  ( -1.878215178124995832, 27.65312499938548640, 5.746835883940462963 ) ) ;
#5753=CARTESIAN_POINT ( 'NONE',  ( -2.000000000000003997, -27.26874999877097139, 5.535898384862238508 ) ) ;
#5754=CARTESIAN_POINT ( 'NONE',  ( 3.756430356250004099, 28.89062499938548356, 6.831223922626973533 ) ) ;
#5764=DIRECTION ( 'NONE',  ( -0.7071067811865487940, -0.7071067811865463515, 0.000000000000000000 ) ) ;
#5768=CARTESIAN_POINT ( 'NONE',  ( -1.878215178125004048, -28.47812499938548569, 5.746835883940462963 ) ) ;
#5777=CARTESIAN_POINT ( 'NONE',  ( 19.37037015225818948, 16.71417277429875625, 12.25316411605952283 ) ) ;
#5778=FACE_OUTER_BOUND ( 'NONE', #22339, .T. ) ;
#5783=CARTESIAN_POINT ( 'NONE',  ( 2.000000000000000888, 27.62500000000000000, 12.46410161513774817 ) ) ;
#5788=VERTEX_POINT ( 'NONE', #8462 ) ;
#5806=CARTESIAN_POINT ( 'NONE',  ( 3.469446951953614189E-15, 30.00000000000000355, 8.999999999999992895 ) ) ;
#5808=EDGE_CURVE ( 'NONE', #21834, #3291, #4680, .T. ) ;
#5812=CARTESIAN_POINT ( 'NONE',  ( 1.878215178125004048, 26.11562499938548498, 5.746835883940462963 ) ) ;
#5816=VECTOR ( 'NONE', #14198, 1000.000000000000000 ) ;
#5818=CARTESIAN_POINT ( 'NONE',  ( 20.09951025522764922, 17.27108313048138655, 5.535898384862238508 ) ) ;
#5819=CARTESIAN_POINT ( 'NONE',  ( 21.35910797434536335, 18.70291059638591946, 12.25316411605952283 ) ) ;
#5820=CARTESIAN_POINT ( 'NONE',  ( -3.834746474454188013E-15, -28.65624999877096712, 4.999999999999992006 ) ) ;
#5828=CARTESIAN_POINT ( 'NONE',  ( 3.999999999999996003, -26.53750000000000142, 6.690598923241487306 ) ) ;
#5833=CARTESIAN_POINT ( 'NONE',  ( 1.071796769724493448, -29.57634618820329564, 4.999999999999995559 ) ) ;
#5835=CARTESIAN_POINT ( 'NONE',  ( -3.403349963601461248, 25.83240171513484285, 20.00001200000000168 ) ) ;
#5836=CARTESIAN_POINT ( 'NONE',  ( 1.626862140677534194E-14, 28.43124999877096570, 12.99999999999999289 ) ) ;
#5845=EDGE_CURVE ( 'NONE', #19280, #14695, #15249, .T. ) ;
#5853=CARTESIAN_POINT ( 'NONE',  ( 19.23330444827413643, 22.06173157302024634, 5.535898384862237620 ) ) ;
#5855=FACE_OUTER_BOUND ( 'NONE', #290, .T. ) ;
#5861=PLANE ( 'NONE',  #24166 ) ;
#5866=CARTESIAN_POINT ( 'NONE',  ( -3.756430356250004099, -25.17812499938548498, 6.831223922626973533 ) ) ;
#5868=ORIENTED_EDGE ( 'NONE', *, *, #11059, .F. ) ;
#5878=CARTESIAN_POINT ( 'NONE',  ( 0.7500000000000001110, 0.000000000000000000, 17.00000000000000000 ) ) ;
#5885=CARTESIAN_POINT ( 'NONE',  ( -3.756430356249996994, 28.17812499938548498, 8.999999999999992895 ) ) ;
#5891=PLANE ( 'NONE',  #25816 ) ;
#5893=CARTESIAN_POINT ( 'NONE',  ( -4.000000000000003553, -29.48124999877096997, 6.690598923241489970 ) ) ;
#5894=CARTESIAN_POINT ( 'NONE',  ( -1.878215178124995832, 27.20312499938548711, 5.746835883940462963 ) ) ;
#5897=CARTESIAN_POINT ( 'NONE',  ( 1.071796769724488563, -26.16115380933863221, 12.99999999999999289 ) ) ;
#5900=CARTESIAN_POINT ( 'NONE',  ( 4.000000000000003553, 28.15000000000000213, 8.999999999999992895 ) ) ;
#5906=CARTESIAN_POINT ( 'NONE',  ( -1.878215178125000939, -28.32812499938548711, 12.25316411605952283 ) ) ;
#5907=ORIENTED_EDGE ( 'NONE', *, *, #21594, .F. ) ;
#5910=ORIENTED_EDGE ( 'NONE', *, *, #8610, .F. ) ;
#5912=CARTESIAN_POINT ( 'NONE',  ( -3.756430356249996994, 26.82812499938548711, 8.999999999999992895 ) ) ;
#5914=AXIS2_PLACEMENT_3D ( 'NONE', #22663, #20690, #18720 ) ;
#5917=CARTESIAN_POINT ( 'NONE',  ( 21.21320343559646915, 21.21320343559638744, 12.99999999999999289 ) ) ;
#5918=CARTESIAN_POINT ( 'NONE',  ( 20.95908693567302450, 20.95908693567294989, 13.33755215474602984 ) ) ;
#5920=DIRECTION ( 'NONE',  ( 0.000000000000000000, 0.000000000000000000, -1.000000000000000000 ) ) ;
#5923=CARTESIAN_POINT ( 'NONE',  ( 4.000000000000003553, 28.63750000000000284, 6.690598923241489970 ) ) ;
#5934=CARTESIAN_POINT ( 'NONE',  ( 19.62663259444009611, 19.62663259444001440, 4.999999999999992006 ) ) ;
#5935=CARTESIAN_POINT ( 'NONE',  ( 1.878215178125004048, 25.32812499938548356, 5.746835883940462963 ) ) ;
#5937=CARTESIAN_POINT ( 'NONE',  ( 16.47558800164659587, 19.30401512639272354, 12.46410161513774639 ) ) ;
#5938=VERTEX_POINT ( 'NONE', #25428 ) ;
#5945=( BOUNDED_CURVE ( )  B_SPLINE_CURVE ( 2, ( #24361, #570, #2513, #20689, #22662, #6439, #22385, #10732, #18719 ),
 .UNSPECIFIED., .F., .F. ) 
 B_SPLINE_CURVE_WITH_KNOTS ( ( 3, 2, 2, 2, 3 ),
 ( 0.5250000000000000222, 0.5333333333333333259, 0.5500000000000000444, 0.5666666666666666519, 0.5750000000000000666 ),
 .UNSPECIFIED. ) 
 CURVE ( )  GEOMETRIC_REPRESENTATION_ITEM ( )  RATIONAL_B_SPLINE_CURVE ( ( 0.9330127018922194093, 0.9330127018922194093, 1.000000000000000000, 0.8660254037844387076, 1.000000000000000000, 0.8660254037844387076, 1.000000000000000000, 0.9330127018922189652, 0.9330127018922194093 ) ) 
 REPRESENTATION_ITEM ( '' )  );
#5951=CARTESIAN_POINT ( 'NONE',  ( 3.756430356250004099, 25.62812499938548072, 6.831223922626973533 ) ) ;
#5956=CARTESIAN_POINT ( 'NONE',  ( 22.75999951944203303, 17.10314526994957873, 6.690598923241489970 ) ) ;
#5966=CARTESIAN_POINT ( 'NONE',  ( 3.999999999999997335, -27.51250000000000284, 11.30940107675849404 ) ) ;
#5972=CARTESIAN_POINT ( 'NONE',  ( -24.00000000000000355, 2.939152317953648289E-15, 17.00000000000000000 ) ) ;
#5987=CARTESIAN_POINT ( 'NONE',  ( 18.51293941407127619, 18.51293941407120869, 13.61880215351699874 ) ) ;
#5988=EDGE_CURVE ( 'NONE', #20014, #8256, #7354, .T. ) ;
#5991=CARTESIAN_POINT ( 'NONE',  ( -24.00000000000000355, 2.939152317953648289E-15, 17.00000000000000000 ) ) ;
#5996=CARTESIAN_POINT ( 'NONE',  ( -3.999999999999995559, 26.48124999877096641, 6.690598923241487306 ) ) ;
#6000=CARTESIAN_POINT ( 'NONE',  ( 4.000000000000003553, 29.50000000000000355, 8.999999999999992895 ) ) ;
#6006=ORIENTED_EDGE ( 'NONE', *, *, #25353, .T. ) ;
#6008=DIRECTION ( 'NONE',  ( -0.7071067811865487940, -0.7071067811865463515, 0.000000000000000000 ) ) ;
#6010=CYLINDRICAL_SURFACE ( 'NONE', #18538, 8.000000000000000000 ) ;
#6016=CARTESIAN_POINT ( 'NONE',  ( -1.878215178124998497, 28.70312499938548356, 12.25316411605951927 ) ) ;
#6024=CARTESIAN_POINT ( 'NONE',  ( -1.878215178125004048, -25.32812499938548356, 5.746835883940462963 ) ) ;
#6025=CARTESIAN_POINT ( 'NONE',  ( -3.756430356249997882, 28.21562499938548285, 11.16877607737301226 ) ) ;
#6030=CARTESIAN_POINT ( 'NONE',  ( 25.99307600111999150, -0.5999999999999996447, 19.59999999999999787 ) ) ;
#6031=CARTESIAN_POINT ( 'NONE',  ( -2.672651547586948120E-15, -29.07812499938548356, 13.33755215474603162 ) ) ;
#6032=ORIENTED_EDGE ( 'NONE', *, *, #13540, .T. ) ;
#6034=FACE_OUTER_BOUND ( 'NONE', #16107, .T. ) ;
#6038=ORIENTED_EDGE ( 'NONE', *, *, #7428, .F. ) ;
#6044=CARTESIAN_POINT ( 'NONE',  ( 1.878215178125004048, 27.57812499938548711, 5.746835883940462963 ) ) ;
#6047=CARTESIAN_POINT ( 'NONE',  ( 18.46426205773553164, 21.12045943569482986, 5.746835883940462963 ) ) ;
#6051=CARTESIAN_POINT ( 'NONE',  ( 3.752267015613588906E-15, 28.71250000000000568, 4.381197846482986158 ) ) ;
#6054=CARTESIAN_POINT ( 'NONE',  ( 20.95908693567301739, 20.95908693567294989, 13.33755215474603162 ) ) ;
#6057=ORIENTED_EDGE ( 'NONE', *, *, #22318, .F. ) ;
#6059=ADVANCED_FACE ( 'NONE', ( #9610 ), #6072, .F. ) ;
#6060=ORIENTED_EDGE ( 'NONE', *, *, #7451, .T. ) ;
#6062=CARTESIAN_POINT ( 'NONE',  ( 4.000000000000001776, 29.85624999877096997, 11.30940107675849760 ) ) ;
#6066=EDGE_CURVE ( 'NONE', #19703, #7733, #25569, .T. ) ;
#6067=CARTESIAN_POINT ( 'NONE',  ( 1.999999999999998224, -25.75000000000000355, 12.46410161513774639 ) ) ;
#6068=ORIENTED_EDGE ( 'NONE', *, *, #3082, .T. ) ;
#6069=DIRECTION ( 'NONE',  ( 0.000000000000000000, 0.000000000000000000, -1.000000000000000000 ) ) ;
#6072=CYLINDRICAL_SURFACE ( 'NONE', #4635, 4.000000000000000000 ) ;
#6077=CARTESIAN_POINT ( 'NONE',  ( 19.50730832598391729, 19.50730832598384623, 13.61880215351699874 ) ) ;
#6079=FACE_OUTER_BOUND ( 'NONE', #18000, .T. ) ;
#6081=CARTESIAN_POINT ( 'NONE',  ( 22.98538980507618845, 17.32853555558373060, 11.30940107675849760 ) ) ;
#6083=EDGE_CURVE ( 'NONE', #7895, #933, #13546, .T. ) ;
#6084=CARTESIAN_POINT ( 'NONE',  ( 21.70382253017380592, 19.04762515221435493, 5.746835883940462963 ) ) ;
#6091=( BOUNDED_CURVE ( )  B_SPLINE_CURVE ( 2, ( #16063, #4404, #5853, #10030, #18273, #4018, #19836, #16319, #14363 ),
 .UNSPECIFIED., .F., .F. ) 
 B_SPLINE_CURVE_WITH_KNOTS ( ( 3, 2, 2, 2, 3 ),
 ( 0.9250000000000000444, 0.9333333333333333481, 0.9499999999999999556, 0.9666666666666666741, 0.9749999999999999778 ),
 .UNSPECIFIED. ) 
 CURVE ( )  GEOMETRIC_REPRESENTATION_ITEM ( )  RATIONAL_B_SPLINE_CURVE ( ( 0.9330127018922194093, 0.9330127018922198534, 1.000000000000000000, 0.8660254037844387076, 1.000000000000000000, 0.8660254037844387076, 1.000000000000000000, 0.9330127018922194093, 0.9330127018922194093 ) ) 
 REPRESENTATION_ITEM ( '' )  );
#6097=CARTESIAN_POINT ( 'NONE',  ( 3.756430356249996105, -25.44062499938548427, 6.831223922626973533 ) ) ;
#6099=CARTESIAN_POINT ( 'NONE',  ( 3.959305739469038251E-15, 30.00000000000000355, 12.99999999999999289 ) ) ;
#6102=DIRECTION ( 'NONE',  ( 0.000000000000000000, -1.000000000000000000, 0.000000000000000000 ) ) ;
#6107=CARTESIAN_POINT ( 'NONE',  ( 20.82429470594385634, 15.16744045645140915, 8.999999999999992895 ) ) ;
#6109=DIRECTION ( 'NONE',  ( 1.000000000000000000, 0.000000000000000000, 0.000000000000000000 ) ) ;
#6111=CARTESIAN_POINT ( 'NONE',  ( 16.87775498257738960, 22.53460923206970179, 8.999999999999992895 ) ) ;
#6112=ORIENTED_EDGE ( 'NONE', *, *, #23921, .F. ) ;
#6113=CARTESIAN_POINT ( 'NONE',  ( 3.137519842735244810E-15, -26.91249999999999787, 4.999999999999991118 ) ) ;
#6121=CARTESIAN_POINT ( 'NONE',  ( -1.999999999999998224, 26.14374999877096784, 12.46410161513774639 ) ) ;
#6134=ADVANCED_FACE ( 'NONE', ( #835 ), #20585, .T. ) ;
#6138=CARTESIAN_POINT ( 'NONE',  ( 2.672651547586948120E-15, 26.37812499938548427, 13.33755215474602984 ) ) ;
#6143=CARTESIAN_POINT ( 'NONE',  ( -5.577813053751546416E-15, -25.73124999877097352, 12.99999999999999289 ) ) ;
#6145=CARTESIAN_POINT ( 'NONE',  ( 1.878215178124995832, -25.40312499938548640, 5.746835883940462963 ) ) ;
#6146=CARTESIAN_POINT ( 'NONE',  ( 3.735045420075836212E-15, 28.96562499938548640, 4.662447845253954171 ) ) ;
#6148=CARTESIAN_POINT ( 'NONE',  ( 3.756430356250003655, 25.19687499938548569, 8.999999999999992895 ) ) ;
#6151=CARTESIAN_POINT ( 'NONE',  ( -2.000000000000000888, -28.97500000000000142, 12.46410161513774817 ) ) ;
#6154=ORIENTED_EDGE ( 'NONE', *, *, #16272, .F. ) ;
#6155=VERTEX_POINT ( 'NONE', #8292 ) ;
#6159=EDGE_LOOP ( 'NONE', ( #9156, #3979 ) ) ;
#6162=CARTESIAN_POINT ( 'NONE',  ( 2.672651547586948120E-15, 25.59062499938548640, 13.33755215474603162 ) ) ;
#6166=CARTESIAN_POINT ( 'NONE',  ( 18.14606400620158411, 20.80226138416088588, 5.746835883940462963 ) ) ;
#6168=CARTESIAN_POINT ( 'NONE',  ( 20.46190248058575634, 20.46190248058568173, 12.99999999999999289 ) ) ;
#6170=VECTOR ( 'NONE', #25169, 1000.000000000000000 ) ;
#6172=CARTESIAN_POINT ( 'NONE',  ( 4.000000000000003553, 27.73750000000000071, 6.690598923241489970 ) ) ;
#6176=CARTESIAN_POINT ( 'NONE',  ( 8.831537335106614961E-15, 27.53124999877097068, 12.99999999999999112 ) ) ;
#6182=CARTESIAN_POINT ( 'NONE',  ( 3.752267015613588906E-15, 29.55624999877096926, 4.381197846482986158 ) ) ;
#6184=CARTESIAN_POINT ( 'NONE',  ( 8.831537335106614961E-15, 27.53124999877097068, 12.99999999999999112 ) ) ;
#6196=CARTESIAN_POINT ( 'NONE',  ( 3.063240906311874401, 29.84319947910909931, 11.57226653943513028 ) ) ;
#6197=CARTESIAN_POINT ( 'NONE',  ( -1.878215178124998497, 26.79062499938548214, 12.25316411605951927 ) ) ;
#6204=CARTESIAN_POINT ( 'NONE',  ( -3.918924903856942255, -29.74337361029841276, 9.928636277907717300 ) ) ;
#6205=DIRECTION ( 'NONE',  ( 0.000000000000000000, 0.000000000000000000, 1.000000000000000000 ) ) ;
#6208=CARTESIAN_POINT ( 'NONE',  ( -3.959305671612554781E-15, -30.00000000000000355, 12.99999999999999289 ) ) ;
#6212=CARTESIAN_POINT ( 'NONE',  ( -4.000000000000003553, -29.50000000000000355, 8.999999999999992895 ) ) ;
#6220=CARTESIAN_POINT ( 'NONE',  ( -3.756430356250003211, -27.54062499938547859, 6.831223922626973533 ) ) ;
#6222=CARTESIAN_POINT ( 'NONE',  ( -2.000000000000003997, -29.06874999877096855, 5.535898384862238508 ) ) ;
#6225=AXIS2_PLACEMENT_3D ( 'NONE', #9454, #7488, #15477 ) ;
#6228=CARTESIAN_POINT ( 'NONE',  ( -27.10000000000000497, -0.5999999999999998668, 19.59999999999999787 ) ) ;
#6230=( BOUNDED_CURVE ( )  B_SPLINE_CURVE ( 2, ( #22010, #21502, #11682, #17967, #7764, #23463, #12063, #19519, #3842 ),
 .UNSPECIFIED., .F., .F. ) 
 B_SPLINE_CURVE_WITH_KNOTS ( ( 3, 2, 2, 2, 3 ),
 ( 0.2750000000000000222, 0.2833333333333333259, 0.2999999999999999889, 0.3166666666666666519, 0.3250000000000000111 ),
 .UNSPECIFIED. ) 
 CURVE ( )  GEOMETRIC_REPRESENTATION_ITEM ( )  RATIONAL_B_SPLINE_CURVE ( ( 0.9330127018922194093, 0.9330127018922196314, 1.000000000000000000, 0.8660254037844387076, 1.000000000000000000, 0.8660254037844387076, 1.000000000000000000, 0.9330127018922191873, 0.9330127018922194093 ) ) 
 REPRESENTATION_ITEM ( '' )  );
#6233=DIRECTION ( 'NONE',  ( 0.000000000000000000, -1.000000000000000000, 0.000000000000000000 ) ) ;
#6236=CARTESIAN_POINT ( 'NONE',  ( 18.19474136253732865, 18.19474136253726826, 12.99999999999999289 ) ) ;
#6238=CARTESIAN_POINT ( 'NONE',  ( 22.05081056025715114, 16.73841580433833442, 6.831223922626973533 ) ) ;
#6239=CARTESIAN_POINT ( 'NONE',  ( 18.02680350200553150, 20.85523062675164851, 12.46410161513774639 ) ) ;
#6240=EDGE_LOOP ( 'NONE', ( #4576, #25529, #4006, #18144 ) ) ;
#6243=( BOUNDED_CURVE ( )  B_SPLINE_CURVE ( 2, ( #20748, #12901, #2827, #20344, #8857, #4669, #499, #24807, #2440 ),
 .UNSPECIFIED., .F., .F. ) 
 B_SPLINE_CURVE_WITH_KNOTS ( ( 3, 2, 2, 2, 3 ),
 ( 0.4250000000000000444, 0.4333333333333333481, 0.4500000000000000111, 0.4666666666666666741, 0.4750000000000000333 ),
 .UNSPECIFIED. ) 
 CURVE ( )  GEOMETRIC_REPRESENTATION_ITEM ( )  RATIONAL_B_SPLINE_CURVE ( ( 0.9330127018922194093, 0.9330127018922196314, 1.000000000000000000, 0.8660254037844387076, 1.000000000000000000, 0.8660254037844387076, 1.000000000000000000, 0.9330127018922191873, 0.9330127018922194093 ) ) 
 REPRESENTATION_ITEM ( '' )  );
#6245=CARTESIAN_POINT ( 'NONE',  ( -3.796077574538131660, 29.75903253174124430, 10.28786097927510923 ) ) ;
#6248=CYLINDRICAL_SURFACE ( 'NONE', #13340, 4.000000000000000000 ) ;
#6249=DIRECTION ( 'NONE',  ( 0.000000000000000000, 1.000000000000000000, 0.000000000000000000 ) ) ;
#6251=CARTESIAN_POINT ( 'NONE',  ( -27.10000000000000497, 0.6000000000000000888, 19.59999999999999787 ) ) ;
#6253=CARTESIAN_POINT ( 'NONE',  ( 1.878215178124998497, -27.24062499938548498, 12.25316411605951927 ) ) ;
#6265=EDGE_CURVE ( 'NONE', #16682, #4650, #16208, .T. ) ;
#6269=CARTESIAN_POINT ( 'NONE',  ( 2.672651547586948120E-15, 26.82812499938548356, 13.33755215474602984 ) ) ;
#6270=VECTOR ( 'NONE', #20027, 1000.000000000000000 ) ;
#6278=EDGE_CURVE ( 'NONE', #4122, #15349, #18747, .T. ) ;
#6279=CARTESIAN_POINT ( 'NONE',  ( 1.878215178124998497, -25.55312499938548854, 12.25316411605951927 ) ) ;
#6281=DIRECTION ( 'NONE',  ( -0.7071067811865487940, -0.7071067811865463515, 0.000000000000000000 ) ) ;
#6287=LINE ( 'NONE', #4844, #22545 ) ;
#6299=CARTESIAN_POINT ( 'NONE',  ( -3.756430356249997438, 25.96562499938548640, 11.16877607737301048 ) ) ;
#6303=CARTESIAN_POINT ( 'NONE',  ( 20.32496430686003208, 17.66876692890059530, 12.25316411605952283 ) ) ;
#6305=FACE_OUTER_BOUND ( 'NONE', #17058, .T. ) ;
#6308=DIRECTION ( 'NONE',  ( 0.000000000000000000, 0.000000000000000000, 1.000000000000000000 ) ) ;
#6309=CARTESIAN_POINT ( 'NONE',  ( 3.756430356250003211, 28.32812499938548356, 6.831223922626973533 ) ) ;
#6312=CARTESIAN_POINT ( 'NONE',  ( -1.999999999999995781, 27.40000000000000213, 5.535898384862237620 ) ) ;
#6313=ORIENTED_EDGE ( 'NONE', *, *, #1804, .F. ) ;
#6327=FACE_OUTER_BOUND ( 'NONE', #7928, .T. ) ;
#6329=CARTESIAN_POINT ( 'NONE',  ( -3.469446951953614189E-15, -30.00000000000000355, 8.999999999999992895 ) ) ;
#6332=AXIS2_PLACEMENT_3D ( 'NONE', #9404, #5474, #17266 ) ;
#6335=CARTESIAN_POINT ( 'NONE',  ( 3.677829432474411853, 29.77381621822422275, 10.59017455026297405 ) ) ;
#6337=CARTESIAN_POINT ( 'NONE',  ( 2.672651547586948120E-15, 28.62812499938548783, 13.33755215474602984 ) ) ;
#6340=CARTESIAN_POINT ( 'NONE',  ( 19.02117241391816904, 21.84959953866428606, 12.46410161513774639 ) ) ;
#6341=CARTESIAN_POINT ( 'NONE',  ( -1.999999999999995781, 29.19999999999999929, 5.535898384862237620 ) ) ;
#6342=CARTESIAN_POINT ( 'NONE',  ( 1.071796769724481901, -27.96115380933863293, 12.99999999999999645 ) ) ;
#6343=VECTOR ( 'NONE', #15678, 1000.000000000000000 ) ;
#6349=CARTESIAN_POINT ( 'NONE',  ( 3.999999999999996003, -27.88750000000000284, 6.690598923241487306 ) ) ;
#6355=( BOUNDED_CURVE ( )  B_SPLINE_CURVE ( 2, ( #8441, #14337, #2032, #14579, #22558, #19929, #18372, #6342, #18247 ),
 .UNSPECIFIED., .F., .F. ) 
 B_SPLINE_CURVE_WITH_KNOTS ( ( 3, 2, 2, 2, 3 ),
 ( 0.5250000000000000222, 0.5333333333333333259, 0.5500000000000000444, 0.5666666666666666519, 0.5750000000000000666 ),
 .UNSPECIFIED. ) 
 CURVE ( )  GEOMETRIC_REPRESENTATION_ITEM ( )  RATIONAL_B_SPLINE_CURVE ( ( 0.9330127018922194093, 0.9330127018922194093, 1.000000000000000000, 0.8660254037844387076, 1.000000000000000000, 0.8660254037844387076, 1.000000000000000000, 0.9330127018922189652, 0.9330127018922194093 ) ) 
 REPRESENTATION_ITEM ( '' )  );
#6358=ORIENTED_EDGE ( 'NONE', *, *, #9183, .F. ) ;
#6359=ORIENTED_EDGE ( 'NONE', *, *, #3657, .F. ) ;
#6360=CARTESIAN_POINT ( 'NONE',  ( 1.878215178124998497, -27.35312499938548569, 12.25316411605951927 ) ) ;
#6374=CARTESIAN_POINT ( 'NONE',  ( 15.91640417120904871, 21.22879892712773042, 8.999999999999992895 ) ) ;
#6375=CARTESIAN_POINT ( 'NONE',  ( 18.55713358789543932, 21.38556071264155634, 5.535898384862237620 ) ) ;
#6378=CARTESIAN_POINT ( 'NONE',  ( 3.469446951953614189E-15, 30.00000000000000355, 4.999999999999992006 ) ) ;
#6381=CARTESIAN_POINT ( 'NONE',  ( -2.642157743709451889, 29.88401080970086099, 12.01472878375391140 ) ) ;
#6383=CARTESIAN_POINT ( 'NONE',  ( 20.43330379829292198, 15.12090904237410527, 8.999999999999992895 ) ) ;
#6386=CYLINDRICAL_SURFACE ( 'NONE', #23444, 0.7500000000000001110 ) ;
#6387=CARTESIAN_POINT ( 'NONE',  ( 4.000000000000001776, 26.70624999877097139, 11.30940107675849760 ) ) ;
#6388=CARTESIAN_POINT ( 'NONE',  ( -3.735045420075836212E-15, -25.70312499938548001, 4.662447845253954171 ) ) ;
#6394=CARTESIAN_POINT ( 'NONE',  ( 3.756430356249997882, -25.40312499938548285, 11.16877607737301226 ) ) ;
#6401=CARTESIAN_POINT ( 'NONE',  ( 1.878215178125004048, 26.56562499938548427, 5.746835883940462963 ) ) ;
#6406=CARTESIAN_POINT ( 'NONE',  ( 21.21320343559646915, 21.21320343559638744, 8.999999999999992895 ) ) ;
#6409=CARTESIAN_POINT ( 'NONE',  ( -4.000000000000003553, -28.09374999877097068, 8.999999999999992895 ) ) ;
#6412=VECTOR ( 'NONE', #2466, 1000.000000000000000 ) ;
#6414=FACE_OUTER_BOUND ( 'NONE', #22402, .T. ) ;
#6417=CYLINDRICAL_SURFACE ( 'NONE', #11657, 4.000000000000000000 ) ;
#6424=ORIENTED_EDGE ( 'NONE', *, *, #10475, .T. ) ;
#6425=DIRECTION ( 'NONE',  ( 0.000000000000000000, -1.000000000000000000, 0.000000000000000000 ) ) ;
#6431=CARTESIAN_POINT ( 'NONE',  ( -3.756430356249996994, 25.92812499938548498, 8.999999999999992895 ) ) ;
#6433=CARTESIAN_POINT ( 'NONE',  ( 3.469446951953614189E-15, 30.00000000000000355, 8.999999999999992895 ) ) ;
#6434=CARTESIAN_POINT ( 'NONE',  ( 17.50966790313369259, 20.16586528109299437, 5.746835883940462963 ) ) ;
#6439=CARTESIAN_POINT ( 'NONE',  ( -3.999999999999997335, 27.90624999877097068, 11.30940107675849404 ) ) ;
#6441=CARTESIAN_POINT ( 'NONE',  ( -3.756430356249996994, 28.06562499938548427, 8.999999999999992895 ) ) ;
#6443=DIRECTION ( 'NONE',  ( -0.000000000000000000, -0.000000000000000000, -1.000000000000000000 ) ) ;
#6456=FACE_OUTER_BOUND ( 'NONE', #557, .T. ) ;
#6465=EDGE_CURVE ( 'NONE', #4650, #23081, #13132, .T. ) ;
#6467=CARTESIAN_POINT ( 'NONE',  ( 3.756430356250004099, 28.32812499938548356, 6.831223922626973533 ) ) ;
#6468=CARTESIAN_POINT ( 'NONE',  ( 20.51285331117640709, 15.20045855525759393, 8.999999999999992895 ) ) ;
#6472=CARTESIAN_POINT ( 'NONE',  ( -3.756430356250002323, -26.00312499938548427, 11.16877607737301403 ) ) ;
#6474=EDGE_LOOP ( 'NONE', ( #18427, #12595, #14889 ) ) ;
#6476=CARTESIAN_POINT ( 'NONE',  ( -2.000000000000000888, -28.97500000000000142, 12.46410161513774817 ) ) ;
#6479=VERTEX_POINT ( 'NONE', #5536 ) ;
#6480=CARTESIAN_POINT ( 'NONE',  ( 3.999999999999997335, -29.25624999877096855, 11.30940107675849404 ) ) ;
#6485=CARTESIAN_POINT ( 'NONE',  ( 3.756430356249996105, -25.89062499938548356, 6.831223922626973533 ) ) ;
#6487=CARTESIAN_POINT ( 'NONE',  ( -4.000000000000001776, -28.95624999877097494, 11.30940107675849760 ) ) ;
#6491=CARTESIAN_POINT ( 'NONE',  ( 21.96892380712053239, 19.14049668237426616, 5.535898384862238508 ) ) ;
#6496=CARTESIAN_POINT ( 'NONE',  ( 21.99777755166815751, 16.68538279574934435, 11.16877607737301226 ) ) ;
#6497=CARTESIAN_POINT ( 'NONE',  ( 17.92073748482754780, 20.74916460957366127, 5.535898384862237620 ) ) ;
#6504=CARTESIAN_POINT ( 'NONE',  ( 21.75237235625120036, 16.09551810675874961, 11.30940107675849760 ) ) ;
#6505=AXIS2_PLACEMENT_3D ( 'NONE', #7206, #9298, #15190 ) ;
#6506=ORIENTED_EDGE ( 'NONE', *, *, #1804, .T. ) ;
#6509=CARTESIAN_POINT ( 'NONE',  ( 3.756430356249996994, -26.26562499938548711, 8.999999999999992895 ) ) ;
#6510=CARTESIAN_POINT ( 'NONE',  ( 17.11198410471449094, 19.94041122946061151, 12.46410161513774639 ) ) ;
#6512=FACE_OUTER_BOUND ( 'NONE', #23813, .T. ) ;
#6514=CARTESIAN_POINT ( 'NONE',  ( -1.878215178125004048, -25.21562499938548285, 5.746835883940462963 ) ) ;
#6516=ORIENTED_EDGE ( 'NONE', *, *, #23757, .F. ) ;
#6524=CARTESIAN_POINT ( 'NONE',  ( -3.756430356249997882, 25.85312499938548925, 11.16877607737301226 ) ) ;
#6526=CARTESIAN_POINT ( 'NONE',  ( 20.50609665440990526, 14.84924240491746339, 8.999999999999992895 ) ) ;
#6527=CARTESIAN_POINT ( 'NONE',  ( 1.999999999999998224, -28.90000000000000213, 12.46410161513774639 ) ) ;
#6531=CARTESIAN_POINT ( 'NONE',  ( -3.999999999999996447, 28.76874999877096784, 8.999999999999992895 ) ) ;
#6532=CARTESIAN_POINT ( 'NONE',  ( 1.878215178124995832, -25.85312499938548569, 5.746835883940462963 ) ) ;
#6537=CARTESIAN_POINT ( 'NONE',  ( 2.004590926901224535, -29.93374515888019971, 5.528701699505815803 ) ) ;
#6540=CARTESIAN_POINT ( 'NONE',  ( -3.469446951953614189E-15, -30.00000000000000355, 4.999999999999992006 ) ) ;
#6544=ORIENTED_EDGE ( 'NONE', *, *, #14170, .F. ) ;
#6546=ORIENTED_EDGE ( 'NONE', *, *, #23210, .T. ) ;
#6551=( BOUNDED_CURVE ( )  B_SPLINE_CURVE ( 2, ( #167, #17947, #23825, #33, #18326 ),
 .UNSPECIFIED., .F., .T. ) 
 B_SPLINE_CURVE_WITH_KNOTS ( ( 3, 2, 3 ),
 ( 0.9749999999999999778, 0.9833333333333332815, 0.9889400238386636399 ),
 .UNSPECIFIED. ) 
 CURVE ( )  GEOMETRIC_REPRESENTATION_ITEM ( )  RATIONAL_B_SPLINE_CURVE ( ( 0.9330127018922194093, 0.9330127018922194093, 1.000000000000000000, 0.9549307542065648136, 0.9401842259098239785 ) ) 
 REPRESENTATION_ITEM ( '' )  );
#6554=CARTESIAN_POINT ( 'NONE',  ( 21.36138144860026600, 16.04898669268145639, 11.16877607737301226 ) ) ;
#6557=CARTESIAN_POINT ( 'NONE',  ( 1.701696020694480449, -26.00000000000000355, 20.00001200000000878 ) ) ;
#6563=CARTESIAN_POINT ( 'NONE',  ( -3.756430356249996994, 29.41562499938548569, 8.999999999999992895 ) ) ;
#6570=ORIENTED_EDGE ( 'NONE', *, *, #16093, .F. ) ;
#6571=CARTESIAN_POINT ( 'NONE',  ( 3.834746474454188013E-15, 28.65624999877096712, 4.999999999999992006 ) ) ;
#6576=CARTESIAN_POINT ( 'NONE',  ( 0.000000000000000000, 0.000000000000000000, 15.00000000000000178 ) ) ;
#6583=DIRECTION ( 'NONE',  ( 0.000000000000000000, 1.000000000000000000, 0.000000000000000000 ) ) ;
#6586=CARTESIAN_POINT ( 'NONE',  ( 16.63462326141533865, 19.29082063937464397, 5.746835883940462963 ) ) ;
#6587=CARTESIAN_POINT ( 'NONE',  ( 1.878215178125000939, 27.31562499938548427, 12.25316411605952283 ) ) ;
#6589=CARTESIAN_POINT ( 'NONE',  ( 20.80453485841585959, 15.49214010249704643, 11.16877607737301403 ) ) ;
#6592=CARTESIAN_POINT ( 'NONE',  ( 20.87601458749065131, 19.36026505963852173, 12.99999999999998757 ) ) ;
#6593=CARTESIAN_POINT ( 'NONE',  ( -1.878215178125000939, -27.76562499938548356, 12.25316411605952283 ) ) ;
#6594=LINE ( 'NONE', #6208, #5816 ) ;
#6597=CARTESIAN_POINT ( 'NONE',  ( -2.000000000000000888, -28.52500000000000213, 12.46410161513774817 ) ) ;
#6604=ORIENTED_EDGE ( 'NONE', *, *, #12674, .T. ) ;
#6605=CARTESIAN_POINT ( 'NONE',  ( -2.672651547586948120E-15, -26.94062499938548783, 13.33755215474603162 ) ) ;
#6612=VECTOR ( 'NONE', #3479, 999.9999999999998863 ) ;
#6614=CARTESIAN_POINT ( 'NONE',  ( 18.73522341023428339, 20.25097293808625665, 12.99999999999999645 ) ) ;
#6619=CARTESIAN_POINT ( 'NONE',  ( 16.87099832581089132, 22.18339308172956237, 8.999999999999992895 ) ) ;
#6620=CARTESIAN_POINT ( 'NONE',  ( 23.30358785661013243, 17.64673360711768169, 11.30940107675849760 ) ) ;
#6630=CARTESIAN_POINT ( 'NONE',  ( 4.000000000000003553, 28.13124999877096855, 6.690598923241489970 ) ) ;
#6631=CARTESIAN_POINT ( 'NONE',  ( -1.878215178125000939, -25.51562499938548356, 12.25316411605952283 ) ) ;
#6633=CARTESIAN_POINT ( 'NONE',  ( 17.78062925563244079, 19.29637878348441404, 12.99999999999999467 ) ) ;
#6638=ORIENTED_EDGE ( 'NONE', *, *, #13633, .T. ) ;
#6639=CARTESIAN_POINT ( 'NONE',  ( 1.878215178124998497, -25.44062499938548427, 12.25316411605951927 ) ) ;
#6643=EDGE_CURVE ( 'NONE', #15394, #17898, #2044, .T. ) ;
#6650=CARTESIAN_POINT ( 'NONE',  ( 21.83060874209248325, 20.31485921424036434, 12.99999999999999467 ) ) ;
#6652=CARTESIAN_POINT ( 'NONE',  ( 3.756430356250003655, 26.49062499938548498, 8.999999999999992895 ) ) ;
#6653=CARTESIAN_POINT ( 'NONE',  ( 17.75721904254721295, 17.75721904254714545, 4.999999999999992006 ) ) ;
#6657=CARTESIAN_POINT ( 'NONE',  ( 21.21320343559646915, 21.21320343559638744, 12.99999999999999289 ) ) ;
#6659=CARTESIAN_POINT ( 'NONE',  ( 16.79378605318053985, 19.62221317792666753, 12.46410161513774639 ) ) ;
#6660=CARTESIAN_POINT ( 'NONE',  ( -3.756430356250003655, -26.15312499938548640, 8.999999999999992895 ) ) ;
#6664=CARTESIAN_POINT ( 'NONE',  ( 3.871726839561290490, -29.74915783848840434, 10.03836643961818886 ) ) ;
#6678=CARTESIAN_POINT ( 'NONE',  ( -3.756430356249997438, 29.11562499938548498, 11.16877607737301048 ) ) ;
#6683=CARTESIAN_POINT ( 'NONE',  ( 22.68720666332504621, 17.37481190740622239, 6.831223922626973533 ) ) ;
#6685=CARTESIAN_POINT ( 'NONE',  ( -1.701696020694465128, -26.00000000000001066, 20.00001200000000878 ) ) ;
#6691=AXIS2_PLACEMENT_3D ( 'NONE', #12016, #2355, #20133 ) ;
#6695=DIRECTION ( 'NONE',  ( 0.000000000000000000, 0.000000000000000000, -1.000000000000000000 ) ) ;
#6697=ORIENTED_EDGE ( 'NONE', *, *, #23757, .T. ) ;
#6703=CARTESIAN_POINT ( 'NONE',  ( 3.756430356249997882, -25.51562499938548356, 11.16877607737301226 ) ) ;
#6704=ORIENTED_EDGE ( 'NONE', *, *, #18730, .F. ) ;
#6713=AXIS2_PLACEMENT_3D ( 'NONE', #23451, #11542, #7752 ) ;
#6716=CARTESIAN_POINT ( 'NONE',  ( 18.22561351908507277, 20.88181089704437454, 5.746835883940462963 ) ) ;
#6718=EDGE_CURVE ( 'NONE', #23467, #19338, #5587, .T. ) ;
#6720=CARTESIAN_POINT ( 'NONE',  ( 1.878215178125004048, 28.81562499938548427, 5.746835883940462963 ) ) ;
#6721=CARTESIAN_POINT ( 'NONE',  ( 19.44991966514168169, 16.79372228718224491, 12.25316411605952283 ) ) ;
#6727=CARTESIAN_POINT ( 'NONE',  ( 0.000000000000000000, 10.00000000000000000, 13.00000000000000178 ) ) ;
#6728=CARTESIAN_POINT ( 'NONE',  ( -3.735045420075836212E-15, -27.50312499938548427, 4.662447845253954171 ) ) ;
#6738=CARTESIAN_POINT ( 'NONE',  ( 3.999999999999996447, -29.21874999877096712, 8.999999999999992895 ) ) ;
#6743=CARTESIAN_POINT ( 'NONE',  ( 1.878215178124995832, -25.85312499938548569, 5.746835883940462963 ) ) ;
#6753=DIRECTION ( 'NONE',  ( 0.000000000000000000, -1.000000000000000000, 0.000000000000000000 ) ) ;
#6754=EDGE_CURVE ( 'NONE', #17713, #6479, #15660, .T. ) ;
#6760=CARTESIAN_POINT ( 'NONE',  ( 20.11283227250407180, 17.45663489454462436, 5.746835883940462963 ) ) ;
#6761=CARTESIAN_POINT ( 'NONE',  ( 20.80453485841585959, 15.49214010249704643, 11.16877607737301226 ) ) ;
#6768=DIRECTION ( 'NONE',  ( 0.7071067811865487940, 0.7071067811865463515, 0.000000000000000000 ) ) ;
#6772=CARTESIAN_POINT ( 'NONE',  ( 2.000000000000000888, 28.91874999877096997, 12.46410161513774817 ) ) ;
#6773=CARTESIAN_POINT ( 'NONE',  ( -3.756430356250004099, -26.52812499938548285, 6.831223922626973533 ) ) ;
#6774=CARTESIAN_POINT ( 'NONE',  ( -1.999999999999998224, 25.69374999877097210, 12.46410161513774639 ) ) ;
#6776=VECTOR ( 'NONE', #59, 1000.000000000000000 ) ;
#6777=LINE ( 'NONE', #20895, #16672 ) ;
#6779=ORIENTED_EDGE ( 'NONE', *, *, #12019, .T. ) ;
#6780=CARTESIAN_POINT ( 'NONE',  ( -3.756430356250003655, -26.04062499938548569, 8.999999999999992895 ) ) ;
#6787=( BOUNDED_CURVE ( )  B_SPLINE_CURVE ( 2, ( #5137, #14818, #16783, #8938, #22791, #9176, #5378, #17168, #6835 ),
 .UNSPECIFIED., .F., .F. ) 
 B_SPLINE_CURVE_WITH_KNOTS ( ( 3, 2, 2, 2, 3 ),
 ( 0.3250000000000000111, 0.3333333333333333148, 0.3499999999999999778, 0.3666666666666666408, 0.3750000000000000000 ),
 .UNSPECIFIED. ) 
 CURVE ( )  GEOMETRIC_REPRESENTATION_ITEM ( )  RATIONAL_B_SPLINE_CURVE ( ( 0.9330127018922194093, 0.9330127018922196314, 1.000000000000000000, 0.8660254037844387076, 1.000000000000000000, 0.8660254037844387076, 1.000000000000000000, 0.9330127018922194093, 0.9330127018922194093 ) ) 
 REPRESENTATION_ITEM ( '' )  );
#6791=CARTESIAN_POINT ( 'NONE',  ( 3.756430356250002323, 29.60312499938548569, 11.16877607737301226 ) ) ;
#6797=PRODUCT_DEFINITION_CONTEXT ( 'detailed design', #8614, 'design' ) ;
#6798=DIRECTION ( 'NONE',  ( 0.000000000000000000, 0.000000000000000000, -1.000000000000000000 ) ) ;
#6799=CARTESIAN_POINT ( 'NONE',  ( 19.01364670445742888, 20.52939623230939858, 12.99999999999999645 ) ) ;
#6801=DIRECTION ( 'NONE',  ( -0.7071067811865487940, -0.7071067811865463515, 0.000000000000000000 ) ) ;
#6802=CARTESIAN_POINT ( 'NONE',  ( -3.735045420075836212E-15, -27.61562499938548498, 4.662447845253954171 ) ) ;
#6804=LINE ( 'NONE', #16885, #12892 ) ;
#6816=CARTESIAN_POINT ( 'NONE',  ( 3.469446951953614189E-15, 30.00000000000000355, 8.999999999999992895 ) ) ;
#6817=VECTOR ( 'NONE', #13979, 1000.000000000000000 ) ;
#6820=CARTESIAN_POINT ( 'NONE',  ( 3.756430356250003655, 28.40312499938548640, 8.999999999999992895 ) ) ;
#6826=CARTESIAN_POINT ( 'NONE',  ( -1.878215178124998497, 26.00312499938548783, 12.25316411605951927 ) ) ;
#6827=EDGE_CURVE ( 'NONE', #10501, #476, #18773, .T. ) ;
#6835=CARTESIAN_POINT ( 'NONE',  ( -1.859271017917182139E-15, -26.68750000000000000, 12.99999999999999289 ) ) ;
#6840=EDGE_CURVE ( 'NONE', #1348, #24947, #9767, .T. ) ;
#6841=EDGE_LOOP ( 'NONE', ( #12278, #4608, #16264, #18489 ) ) ;
#6844=CARTESIAN_POINT ( 'NONE',  ( -3.735045420075836212E-15, -25.36562499938548498, 4.662447845253954171 ) ) ;
#6845=ORIENTED_EDGE ( 'NONE', *, *, #19639, .T. ) ;
#6849=DIRECTION ( 'NONE',  ( -0.7071067811865487940, -0.7071067811865463515, 0.000000000000000000 ) ) ;
#6851=CARTESIAN_POINT ( 'NONE',  ( 1.999999999999995781, -27.40000000000000213, 5.535898384862237620 ) ) ;
#6853=CARTESIAN_POINT ( 'NONE',  ( 17.32411613907045478, 20.15254326381657535, 5.535898384862237620 ) ) ;
#6854=CARTESIAN_POINT ( 'NONE',  ( 18.41350252340144422, 18.41350252340138383, 13.33755215474602984 ) ) ;
#6857=CARTESIAN_POINT ( 'NONE',  ( -3.756430356249996994, 27.61562499938548143, 8.999999999999992895 ) ) ;
#6860=CARTESIAN_POINT ( 'NONE',  ( 17.91631806831418317, 17.91631806831411566, 12.99999999999999289 ) ) ;
#6862=DIRECTION ( 'NONE',  ( 1.000000000000000000, 0.000000000000000000, 0.000000000000000000 ) ) ;
#6864=CARTESIAN_POINT ( 'NONE',  ( 1.878215178124995832, -26.64062499938548711, 5.746835883940462963 ) ) ;
#6865=EDGE_CURVE ( 'NONE', #19049, #8071, #5497, .T. ) ;
#6875=CARTESIAN_POINT ( 'NONE',  ( 1.878215178124995832, -29.45312499938548356, 5.746835883940462963 ) ) ;
#6885=ADVANCED_FACE ( 'NONE', ( #14700 ), #967, .T. ) ;
#6888=CARTESIAN_POINT ( 'NONE',  ( 20.85081121023835138, 15.19395696074590241, 6.690598923241489970 ) ) ;
#6889=CARTESIAN_POINT ( 'NONE',  ( 21.44093096148375466, 16.12853620556493794, 11.16877607737301226 ) ) ;
#6898=CARTESIAN_POINT ( 'NONE',  ( 4.000000000000001776, 28.50624999877096855, 11.30940107675849760 ) ) ;
#6899=CARTESIAN_POINT ( 'NONE',  ( 3.756430356249995661, -29.37812499938548427, 6.831223922626973533 ) ) ;
#6904=CARTESIAN_POINT ( 'NONE',  ( 1.878215178124998497, -28.59062499938548285, 12.25316411605951927 ) ) ;
#6915=CARTESIAN_POINT ( 'NONE',  ( 1.878215178125004048, 28.81562499938548427, 5.746835883940462963 ) ) ;
#6916=CARTESIAN_POINT ( 'NONE',  ( 19.14491610062580662, 16.31648897587954750, 5.535898384862238508 ) ) ;
#6921=CARTESIAN_POINT ( 'NONE',  ( 3.834746474454188013E-15, 25.95624999877096428, 4.999999999999992006 ) ) ;
#6923=CARTESIAN_POINT ( 'NONE',  ( 21.21320343559646915, 21.21320343559638744, 8.999999999999992895 ) ) ;
#6924=CARTESIAN_POINT ( 'NONE',  ( -3.756430356250004099, -26.19062499938548783, 6.831223922626973533 ) ) ;
#6928=CARTESIAN_POINT ( 'NONE',  ( 21.58443449571939965, 18.75600737097314052, 12.46410161513774817 ) ) ;
#6932=DIRECTION ( 'NONE',  ( -0.7071067811865487940, -0.7071067811865463515, 0.000000000000000000 ) ) ;
#6934=VERTEX_POINT ( 'NONE', #24764 ) ;
#6938=VERTEX_POINT ( 'NONE', #14556 ) ;
#6940=ADVANCED_FACE ( 'NONE', ( #12854 ), #20828, .F. ) ;
#6945=EDGE_LOOP ( 'NONE', ( #1371, #24611, #1738 ) ) ;
#6947=CARTESIAN_POINT ( 'NONE',  ( 3.756430356250003655, 29.75312499938548783, 8.999999999999992895 ) ) ;
#6950=CARTESIAN_POINT ( 'NONE',  ( 22.95237170627000367, 17.63997695035117985, 11.16877607737301226 ) ) ;
#6951=CARTESIAN_POINT ( 'NONE',  ( 1.878215178125004048, 25.77812499938548640, 5.746835883940462963 ) ) ;
#6956=CARTESIAN_POINT ( 'NONE',  ( 18.98139765660737055, 21.80982478135348757, 12.46410161513774639 ) ) ;
#6960=CARTESIAN_POINT ( 'NONE',  ( -2.000000000000000888, -25.37500000000000000, 12.46410161513774817 ) ) ;
#6966=CARTESIAN_POINT ( 'NONE',  ( -3.756430356250003655, -25.70312499938548356, 8.999999999999992895 ) ) ;
#6978=CARTESIAN_POINT ( 'NONE',  ( 22.44855812467459089, 17.13616336875576351, 6.831223922626973533 ) ) ;
#6980=CARTESIAN_POINT ( 'NONE',  ( 2.000000000000000888, 25.37500000000000000, 12.46410161513774817 ) ) ;
#6981=CARTESIAN_POINT ( 'NONE',  ( 17.58921741601718125, 20.24541479397648303, 5.746835883940462963 ) ) ;
#6982=DIRECTION ( 'NONE',  ( 0.000000000000000000, -1.000000000000000000, 0.000000000000000000 ) ) ;
#6983=VERTEX_POINT ( 'NONE', #19253 ) ;
#6985=CARTESIAN_POINT ( 'NONE',  ( -1.878215178125000939, -28.21562499938548640, 12.25316411605952283 ) ) ;
#7005=CARTESIAN_POINT ( 'NONE',  ( 20.58122674904192451, 20.58122674904186411, 4.999999999999992006 ) ) ;
#7008=CARTESIAN_POINT ( 'NONE',  ( -3.756430356249996105, 28.02812499938548996, 6.831223922626973533 ) ) ;
#7009=CARTESIAN_POINT ( 'NONE',  ( -3.834746474454188013E-15, -28.20624999877096428, 4.999999999999992006 ) ) ;
#7010=CARTESIAN_POINT ( 'NONE',  ( 20.40224034548861809, 20.40224034548853638, 4.662447845253954171 ) ) ;
#7011=CARTESIAN_POINT ( 'NONE',  ( 17.93620544610052647, 17.93620544610046252, 4.662447845253954171 ) ) ;
#7014=CARTESIAN_POINT ( 'NONE',  ( 23.77396755978151077, 18.29757075420054235, 7.964378325765101962 ) ) ;
#7015=CARTESIAN_POINT ( 'NONE',  ( 21.70609600442870857, 16.39370124850988830, 8.999999999999992895 ) ) ;
#7018=ORIENTED_EDGE ( 'NONE', *, *, #24863, .F. ) ;
#7020=CARTESIAN_POINT ( 'NONE',  ( -1.999999999999998224, 28.84374999877096712, 12.46410161513774639 ) ) ;
#7021=CARTESIAN_POINT ( 'NONE',  ( -3.756430356250002323, -29.15312499938548640, 11.16877607737301226 ) ) ;
#7025=ORIENTED_EDGE ( 'NONE', *, *, #15570, .T. ) ;
#7026=CARTESIAN_POINT ( 'NONE',  ( -1.878215178125000939, -27.76562499938548356, 12.25316411605952283 ) ) ;
#7029=CARTESIAN_POINT ( 'NONE',  ( 20.46846337105369074, 21.93416294652367426, 5.127803451112006528 ) ) ;
#7033=DIRECTION ( 'NONE',  ( 0.000000000000000000, 0.000000000000000000, 1.000000000000000000 ) ) ;
#7039=CARTESIAN_POINT ( 'NONE',  ( 1.878215178125000939, 28.66562499938548569, 12.25316411605952283 ) ) ;
#7042=UNCERTAINTY_MEASURE_WITH_UNIT (LENGTH_MEASURE( 1.000000000000000082E-05 ), #11728, 'distance_accuracy_value', 'NONE');
#7049=CARTESIAN_POINT ( 'NONE',  ( -3.735045420075836212E-15, -26.71562499938548640, 4.662447845253954171 ) ) ;
#7053=CARTESIAN_POINT ( 'NONE',  ( -3.999999999999996447, 26.06874999877096855, 8.999999999999992895 ) ) ;
#7054=CARTESIAN_POINT ( 'NONE',  ( -1.057460391440397258E-14, 29.16249999999999787, 4.999999999999992006 ) ) ;
#7055=AXIS2_PLACEMENT_3D ( 'NONE', #5573, #21519, #5308 ) ;
#7056=VERTEX_POINT ( 'NONE', #23688 ) ;
#7059=ORIENTED_EDGE ( 'NONE', *, *, #7653, .T. ) ;
#7069=EDGE_CURVE ( 'NONE', #23065, #13512, #5404, .T. ) ;
#7070=AXIS2_PLACEMENT_3D ( 'NONE', #9670, #21952, #13713 ) ;
#7075=FACE_OUTER_BOUND ( 'NONE', #16434, .T. ) ;
#7077=CARTESIAN_POINT ( 'NONE',  ( 23.36965697125208408, -11.52193136556784658, 20.00001200000000168 ) ) ;
#7078=VECTOR ( 'NONE', #2298, 1000.000000000000000 ) ;
#7089=CARTESIAN_POINT ( 'NONE',  ( 8.831537335106614961E-15, 27.53124999877097068, 12.99999999999999112 ) ) ;
#7096=DIRECTION ( 'NONE',  ( -0.8660254037844397068, -0.4999999999999983347, 0.000000000000000000 ) ) ;
#7098=CARTESIAN_POINT ( 'NONE',  ( -2.672651547586948120E-15, -25.59062499938548640, 13.33755215474602984 ) ) ;
#7110=CARTESIAN_POINT ( 'NONE',  ( 20.40451381974352074, 17.74831644178408041, 12.25316411605952283 ) ) ;
#7115=CARTESIAN_POINT ( 'NONE',  ( 4.000000000000003553, 25.93750000000000000, 6.690598923241489970 ) ) ;
#7117=EDGE_CURVE ( 'NONE', #22503, #12726, #5267, .T. ) ;
#7118=CARTESIAN_POINT ( 'NONE',  ( 21.46744746577824969, 16.15505270985943298, 8.999999999999992895 ) ) ;
#7119=CARTESIAN_POINT ( 'NONE',  ( 19.18911027444997686, 19.18911027444989870, 12.99999999999999112 ) ) ;
#7120=ORIENTED_EDGE ( 'NONE', *, *, #18264, .F. ) ;
#7123=CARTESIAN_POINT ( 'NONE',  ( -3.735045420075836212E-15, -26.60312499938547859, 4.662447845253954171 ) ) ;
#7126=FACE_OUTER_BOUND ( 'NONE', #19823, .T. ) ;
#7135=CARTESIAN_POINT ( 'NONE',  ( 3.756430356249997438, -29.11562499938548498, 11.16877607737301048 ) ) ;
#7136=LINE ( 'NONE', #24658, #14717 ) ;
#7141=EDGE_CURVE ( 'NONE', #1926, #21566, #15603, .T. ) ;
#7145=ADVANCED_FACE ( 'NONE', ( #17155 ), #21194, .F. ) ;
#7148=CARTESIAN_POINT ( 'NONE',  ( -1.878215178124995832, 27.09062499938548640, 5.746835883940462963 ) ) ;
#7149=LINE ( 'NONE', #15139, #10368 ) ;
#7150=CARTESIAN_POINT ( 'NONE',  ( 21.59775651299582222, 18.94155913503637478, 12.25316411605952283 ) ) ;
#7151=CARTESIAN_POINT ( 'NONE',  ( 15.99595368409253915, 21.30834844001121553, 8.999999999999992895 ) ) ;
#7152=CARTESIAN_POINT ( 'NONE',  ( 18.59690834520624136, 21.42533546995235838, 5.535898384862237620 ) ) ;
#7155=CARTESIAN_POINT ( 'NONE',  ( 15.91640417120904871, 21.22879892712773042, 8.999999999999992895 ) ) ;
#7156=CARTESIAN_POINT ( 'NONE',  ( 22.28712185865447637, 19.45869473390820659, 5.535898384862238508 ) ) ;
#7158=CARTESIAN_POINT ( 'NONE',  ( -27.10000000000000497, 0.6000000000000000888, 19.00000000000000000 ) ) ;
#7159=CARTESIAN_POINT ( 'NONE',  ( -3.999999999999996003, 27.38124999877096855, 6.690598923241487306 ) ) ;
#7160=CARTESIAN_POINT ( 'NONE',  ( -3.756430356250002323, -28.25312499938548427, 11.16877607737301226 ) ) ;
#7167=CARTESIAN_POINT ( 'NONE',  ( -2.672651547586948120E-15, -28.62812499938548783, 13.33755215474602984 ) ) ;
#7168=ORIENTED_EDGE ( 'NONE', *, *, #14772, .T. ) ;
#7169=PRODUCT ( 'casing', 'casing', '', ( #7276 ) ) ;
#7171=CARTESIAN_POINT ( 'NONE',  ( 20.46600609040033447, 21.93646478979743719, 12.87134967428165666 ) ) ;
#7175=DIRECTION ( 'NONE',  ( 1.000000000000000000, 0.000000000000000000, 0.000000000000000000 ) ) ;
#7178=CARTESIAN_POINT ( 'NONE',  ( -8.831537335106614961E-15, -27.53124999877097068, 12.99999999999999112 ) ) ;
#7183=CARTESIAN_POINT ( 'NONE',  ( 16.90427148687188819, 22.56112573636419683, 11.30940107675849404 ) ) ;
#7185=DIRECTION ( 'NONE',  ( 0.8660254037844397068, -0.4999999999999983347, 0.000000000000000000 ) ) ;
#7187=CARTESIAN_POINT ( 'NONE',  ( 1.878215178124998497, -29.15312499938548640, 12.25316411605951927 ) ) ;
#7190=ADVANCED_FACE ( 'NONE', ( #7075 ), #225, .F. ) ;
#7198=CARTESIAN_POINT ( 'NONE',  ( 21.05852382634284936, 21.05852382634277831, 12.99999999999999289 ) ) ;
#7206=CARTESIAN_POINT ( 'NONE',  ( -3.469446951953614189E-15, -30.00000000000000355, 8.999999999999992895 ) ) ;
#7212=CARTESIAN_POINT ( 'NONE',  ( 21.27955846146187113, 18.62336108350243080, 12.25316411605952283 ) ) ;
#7213=CARTESIAN_POINT ( 'NONE',  ( 2.672651547586948120E-15, 26.49062499938548143, 13.33755215474602984 ) ) ;
#7215=FACE_OUTER_BOUND ( 'NONE', #18703, .T. ) ;
#7224=CARTESIAN_POINT ( 'NONE',  ( -3.834746474454188013E-15, -25.56250000000000000, 4.999999999999992006 ) ) ;
#7227=ORIENTED_EDGE ( 'NONE', *, *, #2985, .F. ) ;
#7229=EDGE_CURVE ( 'NONE', #17829, #990, #10129, .T. ) ;
#7231=CARTESIAN_POINT ( 'NONE',  ( -3.878215178125003604, -29.82343749907822783, 8.999999999999992895 ) ) ;
#7244=CARTESIAN_POINT ( 'NONE',  ( 21.46744746577824969, 16.15505270985943298, 8.999999999999992895 ) ) ;
#7247=CARTESIAN_POINT ( 'NONE',  ( 3.756430356250002323, 29.60312499938548569, 11.16877607737301226 ) ) ;
#7248=( BOUNDED_CURVE ( )  B_SPLINE_CURVE ( 2, ( #16971, #1266, #15003, #9105, #17095, #25070, #7156, #23115, #11188 ),
 .UNSPECIFIED., .F., .F. ) 
 B_SPLINE_CURVE_WITH_KNOTS ( ( 3, 2, 2, 2, 3 ),
 ( 0.8750000000000000000, 0.8833333333333333037, 0.9000000000000000222, 0.9166666666666666297, 0.9249999999999999334 ),
 .UNSPECIFIED. ) 
 CURVE ( )  GEOMETRIC_REPRESENTATION_ITEM ( )  RATIONAL_B_SPLINE_CURVE ( ( 0.9330127018922194093, 0.9330127018922194093, 1.000000000000000000, 0.8660254037844387076, 1.000000000000000000, 0.8660254037844387076, 1.000000000000000000, 0.9330127018922198534, 0.9330127018922194093 ) ) 
 REPRESENTATION_ITEM ( '' )  );
#7249=CARTESIAN_POINT ( 'NONE',  ( 21.81216202160669226, 16.49976726568787200, 6.831223922626973533 ) ) ;
#7251=EDGE_LOOP ( 'NONE', ( #7677, #16236, #16443, #1863 ) ) ;
#7255=CARTESIAN_POINT ( 'NONE',  ( -3.756430356250002323, -28.70312499938548356, 11.16877607737301403 ) ) ;
#7257=ORIENTED_EDGE ( 'NONE', *, *, #23882, .F. ) ;
#7261=ORIENTED_EDGE ( 'NONE', *, *, #5304, .T. ) ;
#7262=ADVANCED_FACE ( 'NONE', ( #16152 ), #3715, .F. ) ;
#7268=CARTESIAN_POINT ( 'NONE',  ( -3.756430356250003655, -29.30312499938548498, 8.999999999999992895 ) ) ;
#7269=CARTESIAN_POINT ( 'NONE',  ( 1.859271017917182139E-15, 25.78750000000000142, 12.99999999999999289 ) ) ;
#7271=EDGE_CURVE ( 'NONE', #21566, #5410, #5103, .T. ) ;
#7273=CARTESIAN_POINT ( 'NONE',  ( 22.38876845931909187, 16.73191420982663757, 11.30940107675849760 ) ) ;
#7276=PRODUCT_CONTEXT ( 'NONE', #599, 'mechanical' ) ;
#7278=CARTESIAN_POINT ( 'NONE',  ( -3.959305671612554781E-15, -30.00000000000000355, 12.99999999999999289 ) ) ;
#7279=CARTESIAN_POINT ( 'NONE',  ( 3.756430356250003211, 26.07812499938548356, 6.831223922626973533 ) ) ;
#7281=CARTESIAN_POINT ( 'NONE',  ( 20.08404229395466700, 20.08404229395459240, 4.662447845253954171 ) ) ;
#7282=CARTESIAN_POINT ( 'NONE',  ( 15.96943717979804056, 21.28183193571671694, 6.831223922626973533 ) ) ;
#7283=CARTESIAN_POINT ( 'NONE',  ( 16.26787538380399312, 21.92472963329630531, 11.30940107675849404 ) ) ;
#7287=CARTESIAN_POINT ( 'NONE',  ( 21.38562447863985483, 18.72942710068040739, 5.746835883940462963 ) ) ;
#7291=CARTESIAN_POINT ( 'NONE',  ( 2.672651547586948120E-15, 26.49062499938548143, 13.33755215474602984 ) ) ;
#7292=CARTESIAN_POINT ( 'NONE',  ( -3.735045420075836212E-15, -27.95312499938548001, 4.662447845253954171 ) ) ;
#7297=CARTESIAN_POINT ( 'NONE',  ( -3.756430356250004099, -27.87812499938548427, 6.831223922626973533 ) ) ;
#7300=CARTESIAN_POINT ( 'NONE',  ( 18.61651080183891338, 23.52545784775749382, 6.994934987683498306 ) ) ;
#7302=EDGE_CURVE ( 'NONE', #6155, #12209, #2571, .T. ) ;
#7306=CARTESIAN_POINT ( 'NONE',  ( 3.999999999999996447, -27.41874999877096641, 8.999999999999992895 ) ) ;
#7310=CARTESIAN_POINT ( 'NONE',  ( -3.137519842735244810E-15, 26.46249999999999858, 4.999999999999991118 ) ) ;
#7313=CARTESIAN_POINT ( 'NONE',  ( -2.000000000000003997, -27.71874999877097068, 5.535898384862238508 ) ) ;
#7314=CARTESIAN_POINT ( 'NONE',  ( -2.672651547586948120E-15, -28.74062499938548498, 13.33755215474602984 ) ) ;
#7316=PLANE ( 'NONE',  #11234 ) ;
#7319=CARTESIAN_POINT ( 'NONE',  ( -4.000000000000003553, -25.00000000000000000, 8.999999999999992895 ) ) ;
#7328=DIRECTION ( 'NONE',  ( 0.000000000000000000, -1.000000000000000000, 0.000000000000000000 ) ) ;
#7329=CARTESIAN_POINT ( 'NONE',  ( 0.000000000000000000, 0.000000000000000000, 19.59999999999999787 ) ) ;
#7335=CARTESIAN_POINT ( 'NONE',  ( 3.756430356250002323, 25.66562499938548569, 11.16877607737301226 ) ) ;
#7342=CARTESIAN_POINT ( 'NONE',  ( -3.469446951953614189E-15, -30.00000000000000355, 4.999999999999992006 ) ) ;
#7344=CARTESIAN_POINT ( 'NONE',  ( -2.000000000000000888, -26.21874999877096712, 12.46410161513774817 ) ) ;
#7349=EDGE_LOOP ( 'NONE', ( #4683, #15048, #1416, #12309 ) ) ;
#7354=( BOUNDED_CURVE ( )  B_SPLINE_CURVE ( 2, ( #18915, #19034, #1115, #7273, #17077, #25051, #1247, #9230, #21634 ),
 .UNSPECIFIED., .F., .F. ) 
 B_SPLINE_CURVE_WITH_KNOTS ( ( 3, 2, 2, 2, 3 ),
 ( 0.5750000000000000666, 0.5833333333333333703, 0.5999999999999999778, 0.6166666666666666963, 0.6250000000000000000 ),
 .UNSPECIFIED. ) 
 CURVE ( )  GEOMETRIC_REPRESENTATION_ITEM ( )  RATIONAL_B_SPLINE_CURVE ( ( 0.9330127018922194093, 0.9330127018922198534, 1.000000000000000000, 0.8660254037844387076, 1.000000000000000000, 0.8660254037844387076, 1.000000000000000000, 0.9330127018922194093, 0.9330127018922194093 ) ) 
 REPRESENTATION_ITEM ( '' )  );
#7355=ORIENTED_EDGE ( 'NONE', *, *, #10213, .F. ) ;
#7357=CARTESIAN_POINT ( 'NONE',  ( 1.878215178124998497, -29.15312499938548640, 12.25316411605951927 ) ) ;
#7366=CARTESIAN_POINT ( 'NONE',  ( 20.16359180683815921, 20.16359180683807750, 4.662447845253954171 ) ) ;
#7368=CARTESIAN_POINT ( 'NONE',  ( 2.000000000000003997, 25.97500000000000142, 5.535898384862238508 ) ) ;
#7369=CARTESIAN_POINT ( 'NONE',  ( 16.95054783869437642, 22.26294259461305103, 8.999999999999992895 ) ) ;
#7370=CARTESIAN_POINT ( 'NONE',  ( -4.000000000000003553, -25.19687499938548569, 8.999999999999992895 ) ) ;
#7371=ORIENTED_EDGE ( 'NONE', *, *, #3301, .T. ) ;
#7374=CARTESIAN_POINT ( 'NONE',  ( -3.756430356250003211, -28.77812499938548285, 6.831223922626973533 ) ) ;
#7378=DIRECTION ( 'NONE',  ( 0.000000000000000000, 1.000000000000000000, 0.000000000000000000 ) ) ;
#7379=ORIENTED_EDGE ( 'NONE', *, *, #3657, .T. ) ;
#7380=ORIENTED_EDGE ( 'NONE', *, *, #15303, .T. ) ;
#7381=DIRECTION ( 'NONE',  ( 0.000000000000000000, -1.000000000000000000, 0.000000000000000000 ) ) ;
#7382=CARTESIAN_POINT ( 'NONE',  ( -3.878215178125003604, -25.07031249969274356, 8.999999999999992895 ) ) ;
#7395=CARTESIAN_POINT ( 'NONE',  ( -1.878215178124995832, 26.19062499938548427, 5.746835883940462963 ) ) ;
#7397=CARTESIAN_POINT ( 'NONE',  ( 23.00540471485899374, 17.69300995894016992, 6.831223922626973533 ) ) ;
#7398=CARTESIAN_POINT ( 'NONE',  ( 22.71372316761954124, 17.40132841170072808, 11.16877607737301226 ) ) ;
#7400=CARTESIAN_POINT ( 'NONE',  ( 21.21320343559646915, 21.21320343559638744, 8.999999999999992895 ) ) ;
#7403=CARTESIAN_POINT ( 'NONE',  ( 21.73261250872320005, 16.42021775280438689, 6.831223922626973533 ) ) ;
#7404=DIRECTION ( 'NONE',  ( 0.000000000000000000, -1.000000000000000000, 0.000000000000000000 ) ) ;
#7407=CARTESIAN_POINT ( 'NONE',  ( 3.756430356250003655, 26.60312499938548569, 8.999999999999992895 ) ) ;
#7408=CARTESIAN_POINT ( 'NONE',  ( -1.878215178125000939, -29.56562499938548427, 12.25316411605952283 ) ) ;
#7413=CARTESIAN_POINT ( 'NONE',  ( -3.756430356250003655, -28.74062499938548498, 8.999999999999992895 ) ) ;
#7416=CARTESIAN_POINT ( 'NONE',  ( 18.35963726379211991, 23.72622656523767759, 7.708599238039754553 ) ) ;
#7421=CARTESIAN_POINT ( 'NONE',  ( 1.999999999999995781, -27.34374999877097068, 5.535898384862237620 ) ) ;
#7425=CARTESIAN_POINT ( 'NONE',  ( -1.071796769724488563, 27.06115380933863435, 12.99999999999999289 ) ) ;
#7426=CARTESIAN_POINT ( 'NONE',  ( -0.5000000000000001110, 10.00000000000000000, 15.00000000000000178 ) ) ;
#7427=CARTESIAN_POINT ( 'NONE',  ( 18.35384038830430597, 18.35384038830423492, 4.381197846482986158 ) ) ;
#7428=EDGE_CURVE ( 'NONE', #9493, #16293, #8790, .T. ) ;
#7430=CARTESIAN_POINT ( 'NONE',  ( -4.000000000000003553, -27.68124999877096926, 6.690598923241489970 ) ) ;
#7431=CARTESIAN_POINT ( 'NONE',  ( -3.756430356250004099, -28.89062499938548356, 6.831223922626973533 ) ) ;
#7436=CARTESIAN_POINT ( 'NONE',  ( -4.000000000000001776, -28.56249999999999645, 11.30940107675849760 ) ) ;
#7437=ORIENTED_EDGE ( 'NONE', *, *, #17040, .F. ) ;
#7447=ORIENTED_EDGE ( 'NONE', *, *, #21042, .T. ) ;
#7451=EDGE_CURVE ( 'NONE', #17713, #12604, #10894, .T. ) ;
#7455=CARTESIAN_POINT ( 'NONE',  ( -3.756430356249997882, 27.31562499938548427, 11.16877607737301226 ) ) ;
#7457=VECTOR ( 'NONE', #10038, 1000.000000000000000 ) ;
#7462=DIRECTION ( 'NONE',  ( -0.000000000000000000, -0.000000000000000000, 1.000000000000000000 ) ) ;
#7464=CARTESIAN_POINT ( 'NONE',  ( -2.000000000000003997, -25.91874999877096997, 5.535898384862238508 ) ) ;
#7466=AXIS2_PLACEMENT_3D ( 'NONE', #19026, #991, #23207 ) ;
#7476=FACE_OUTER_BOUND ( 'NONE', #25004, .T. ) ;
#7478=CARTESIAN_POINT ( 'NONE',  ( 1.878215178124998497, -26.90312499938548285, 12.25316411605951927 ) ) ;
#7483=ORIENTED_EDGE ( 'NONE', *, *, #16907, .F. ) ;
#7488=DIRECTION ( 'NONE',  ( 0.000000000000000000, 0.000000000000000000, 1.000000000000000000 ) ) ;
#7489=CARTESIAN_POINT ( 'NONE',  ( 21.46517399152334704, 18.80897661356389605, 5.746835883940462963 ) ) ;
#7491=CARTESIAN_POINT ( 'NONE',  ( 4.000000000000003553, 25.00000000000000000, 8.999999999999992895 ) ) ;
#7492=CARTESIAN_POINT ( 'NONE',  ( 18.89079960070236908, 18.89079960070229802, 4.662447845253954171 ) ) ;
#7495=ORIENTED_EDGE ( 'NONE', *, *, #12221, .F. ) ;
#7499=CARTESIAN_POINT ( 'NONE',  ( 4.000000000000003553, 28.18750000000000000, 6.690598923241489970 ) ) ;
#7500=ORIENTED_EDGE ( 'NONE', *, *, #9920, .T. ) ;
#7507=ORIENTED_EDGE ( 'NONE', *, *, #3335, .F. ) ;
#7511=LINE ( 'NONE', #23601, #19349 ) ;
#7517=CARTESIAN_POINT ( 'NONE',  ( 3.735045420075836212E-15, 29.30312499938548498, 4.662447845253954171 ) ) ;
#7518=CARTESIAN_POINT ( 'NONE',  ( 8.831537335106614961E-15, 27.13750000000000284, 12.99999999999999112 ) ) ;
#7520=CARTESIAN_POINT ( 'NONE',  ( 1.878215178125004048, 27.01562499938548711, 5.746835883940462963 ) ) ;
#7523=CARTESIAN_POINT ( 'NONE',  ( 22.12360341637413796, 16.46674916688168366, 6.690598923241489970 ) ) ;
#7525=CARTESIAN_POINT ( 'NONE',  ( 18.96807563933094798, 21.62427301729024975, 12.25316411605951927 ) ) ;
#7531=CARTESIAN_POINT ( 'NONE',  ( 21.41441445718925962, 16.10201970127043936, 6.831223922626973533 ) ) ;
#7534=CARTESIAN_POINT ( 'NONE',  ( 19.99344423804966198, 17.16501711330340996, 12.46410161513774817 ) ) ;
#7535=CARTESIAN_POINT ( 'NONE',  ( 1.999999999999995781, -26.50000000000000355, 5.535898384862237620 ) ) ;
#7537=VERTEX_POINT ( 'NONE', #9047 ) ;
#7540=DIRECTION ( 'NONE',  ( 0.000000000000000000, -1.000000000000000000, 0.000000000000000000 ) ) ;
#7541=CARTESIAN_POINT ( 'NONE',  ( -23.36965697125209473, 11.52193136556784481, 20.00001200000000168 ) ) ;
#7544=VERTEX_POINT ( 'NONE', #21335 ) ;
#7546=CARTESIAN_POINT ( 'NONE',  ( 18.84633213526256768, 23.34175242840538900, 6.557713274934320324 ) ) ;
#7548=( BOUNDED_CURVE ( )  B_SPLINE_CURVE ( 2, ( #7893, #16412, #9860, #15882, #23856, #23984, #6067, #22015, #4095 ),
 .UNSPECIFIED., .F., .F. ) 
 B_SPLINE_CURVE_WITH_KNOTS ( ( 3, 2, 2, 2, 3 ),
 ( 0.1250000000000000000, 0.1333333333333333315, 0.1499999999999999944, 0.1666666666666666574, 0.1749999999999999889 ),
 .UNSPECIFIED. ) 
 CURVE ( )  GEOMETRIC_REPRESENTATION_ITEM ( )  RATIONAL_B_SPLINE_CURVE ( ( 0.9330127018922194093, 0.9330127018922194093, 1.000000000000000000, 0.8660254037844387076, 1.000000000000000000, 0.8660254037844387076, 1.000000000000000000, 0.9330127018922194093, 0.9330127018922194093 ) ) 
 REPRESENTATION_ITEM ( '' )  );
#7562=DIRECTION ( 'NONE',  ( 0.000000000000000000, 1.000000000000000000, 0.000000000000000000 ) ) ;
#7564=CARTESIAN_POINT ( 'NONE',  ( 18.19474136253732865, 18.19474136253726471, 13.61880215351699874 ) ) ;
#7565=ORIENTED_EDGE ( 'NONE', *, *, #2001, .F. ) ;
#7566=CARTESIAN_POINT ( 'NONE',  ( -3.999999999999996447, 27.47499999999999787, 8.999999999999992895 ) ) ;
#7569=CARTESIAN_POINT ( 'NONE',  ( -27.10000000000000497, -0.5999999999999998668, 19.59999999999999787 ) ) ;
#7572=CARTESIAN_POINT ( 'NONE',  ( 1.859271017917182139E-15, 28.88124999877096499, 12.99999999999999289 ) ) ;
#7588=EDGE_CURVE ( 'NONE', #23573, #9107, #9071, .T. ) ;
#7595=CARTESIAN_POINT ( 'NONE',  ( 1.878215178125000939, 27.42812499938548498, 12.25316411605952283 ) ) ;
#7603=CARTESIAN_POINT ( 'NONE',  ( -4.000000000000003553, -27.23124999877096997, 6.690598923241489970 ) ) ;
#7605=CARTESIAN_POINT ( 'NONE',  ( 2.672651547586948120E-15, 28.74062499938548498, 13.33755215474602984 ) ) ;
#7606=CARTESIAN_POINT ( 'NONE',  ( 0.000000000000000000, 10.00000000000000000, 13.00000000000000178 ) ) ;
#7612=ORIENTED_EDGE ( 'NONE', *, *, #4182, .T. ) ;
#7613=CARTESIAN_POINT ( 'NONE',  ( -3.834746474454188013E-15, -28.65624999877096712, 4.999999999999992006 ) ) ;
#7614=VERTEX_POINT ( 'NONE', #21583 ) ;
#7615=CARTESIAN_POINT ( 'NONE',  ( 3.756430356249997882, -29.11562499938548143, 11.16877607737301226 ) ) ;
#7620=ORIENTED_EDGE ( 'NONE', *, *, #24390, .F. ) ;
#7626=CARTESIAN_POINT ( 'NONE',  ( 20.43330379829292198, 15.12090904237410527, 8.999999999999992895 ) ) ;
#7627=( BOUNDED_CURVE ( )  B_SPLINE_CURVE ( 2, ( #6236, #16814, #4143, #235, #8206, #9898, #22693, #16179, #17884 ),
 .UNSPECIFIED., .F., .F. ) 
 B_SPLINE_CURVE_WITH_KNOTS ( ( 3, 2, 2, 2, 3 ),
 ( 0.07500000000000001110, 0.08333333333333332871, 0.1000000000000000056, 0.1166666666666666685, 0.1249999999999999861 ),
 .UNSPECIFIED. ) 
 CURVE ( )  GEOMETRIC_REPRESENTATION_ITEM ( )  RATIONAL_B_SPLINE_CURVE ( ( 0.9330127018922192983, 0.9330127018922194093, 1.000000000000000000, 0.8660254037844387076, 1.000000000000000000, 0.8660254037844387076, 1.000000000000000000, 0.9330127018922195203, 0.9330127018922194093 ) ) 
 REPRESENTATION_ITEM ( '' )  );
#7630=CARTESIAN_POINT ( 'NONE',  ( -1.999999999999995781, 27.40000000000000213, 5.535898384862237620 ) ) ;
#7651=CARTESIAN_POINT ( 'NONE',  ( -1.859271017917182139E-15, -26.68750000000000000, 12.99999999999999289 ) ) ;
#7653=EDGE_CURVE ( 'NONE', #14487, #9154, #3544, .T. ) ;
#7654=COLOUR_RGB ( '',0.8941176470588234615, 0.8941176470588234615, 0.8941176470588234615 ) ;
#7655=CARTESIAN_POINT ( 'NONE',  ( -1.878215178124995832, 27.99062499938548143, 5.746835883940462963 ) ) ;
#7660=CARTESIAN_POINT ( 'NONE',  ( 2.672651547586948120E-15, 28.62812499938548783, 13.33755215474603162 ) ) ;
#7661=PLANE ( 'NONE',  #7055 ) ;
#7662=CARTESIAN_POINT ( 'NONE',  ( 21.77888886054569539, 16.12203461105324820, 8.999999999999992895 ) ) ;
#7663=CARTESIAN_POINT ( 'NONE',  ( 22.42204162038009230, 17.10964686446126848, 8.999999999999992895 ) ) ;
#7664=DIRECTION ( 'NONE',  ( 0.000000000000000000, 0.000000000000000000, -1.000000000000000000 ) ) ;
#7667=CARTESIAN_POINT ( 'NONE',  ( 18.14379053194667790, 23.45618528786534895, 8.999999999999992895 ) ) ;
#7668=DIRECTION ( 'NONE',  ( 1.000000000000000000, 0.000000000000000000, 0.000000000000000000 ) ) ;
#7671=CARTESIAN_POINT ( 'NONE',  ( -2.000000000000000888, -26.27499999999999858, 12.46410161513774817 ) ) ;
#7677=ORIENTED_EDGE ( 'NONE', *, *, #23921, .T. ) ;
#7679=ORIENTED_EDGE ( 'NONE', *, *, #44, .T. ) ;
#7694=DIRECTION ( 'NONE',  ( 0.000000000000000000, 0.000000000000000000, 1.000000000000000000 ) ) ;
#7695=CARTESIAN_POINT ( 'NONE',  ( 17.60253943329360382, 20.43096655803972084, 5.535898384862237620 ) ) ;
#7698=CARTESIAN_POINT ( 'NONE',  ( 1.878215178124995832, -28.55312499938548498, 5.746835883940462963 ) ) ;
#7702=CARTESIAN_POINT ( 'NONE',  ( 1.071796769724487675, 29.08615380933863293, 4.999999999999988454 ) ) ;
#7708=ORIENTED_EDGE ( 'NONE', *, *, #13171, .F. ) ;
#7711=ORIENTED_EDGE ( 'NONE', *, *, #21354, .T. ) ;
#7715=CARTESIAN_POINT ( 'NONE',  ( 1.071796769724493448, -29.18259618943233136, 4.999999999999995559 ) ) ;
#7721=CARTESIAN_POINT ( 'NONE',  ( -3.756430356249997882, 27.76562499938549067, 11.16877607737301226 ) ) ;
#7723=CARTESIAN_POINT ( 'NONE',  ( 20.28643891059321902, 21.80218843844518872, 12.99999999999999289 ) ) ;
#7728=CARTESIAN_POINT ( 'NONE',  ( -2.000000000000000888, -27.11874999877096926, 12.46410161513774817 ) ) ;
#7729=CARTESIAN_POINT ( 'NONE',  ( 3.756430356250002323, 28.81562499938548427, 11.16877607737301226 ) ) ;
#7733=VERTEX_POINT ( 'NONE', #5509 ) ;
#7735=CARTESIAN_POINT ( 'NONE',  ( 2.000000000000003997, 25.46874999877096712, 5.535898384862238508 ) ) ;
#7736=VERTEX_POINT ( 'NONE', #19757 ) ;
#7739=DIRECTION ( 'NONE',  ( 1.000000000000000000, 0.000000000000000000, 0.000000000000000000 ) ) ;
#7740=EDGE_LOOP ( 'NONE', ( #8481, #20152, #15430 ) ) ;
#7741=CARTESIAN_POINT ( 'NONE',  ( 3.756430356249996994, -28.17812499938548498, 8.999999999999992895 ) ) ;
#7743=CARTESIAN_POINT ( 'NONE',  ( -1.071796769724493448, 28.73259618943232852, 4.999999999999995559 ) ) ;
#7751=CARTESIAN_POINT ( 'NONE',  ( 17.93165849759071762, 23.24405325350938867, 11.16877607737301226 ) ) ;
#7752=DIRECTION ( 'NONE',  ( -1.000000000000000000, 0.000000000000000000, 0.000000000000000000 ) ) ;
#7754=CARTESIAN_POINT ( 'NONE',  ( -1.999999999999998224, 27.55000000000000071, 12.46410161513774639 ) ) ;
#7756=CARTESIAN_POINT ( 'NONE',  ( 22.31370212894720240, 19.65750475098775496, 12.25316411605952283 ) ) ;
#7758=ORIENTED_EDGE ( 'NONE', *, *, #7302, .T. ) ;
#7764=CARTESIAN_POINT ( 'NONE',  ( 4.000000000000003553, 26.35000000000000142, 8.999999999999992895 ) ) ;
#7765=CARTESIAN_POINT ( 'NONE',  ( 17.07220934740368889, 19.90063647214981302, 12.46410161513774639 ) ) ;
#7766=CARTESIAN_POINT ( 'NONE',  ( 15.00834143068450999, 20.66519568017682573, 8.999999999999992895 ) ) ;
#7769=( BOUNDED_CURVE ( )  B_SPLINE_CURVE ( 2, ( #6468, #10366, #2544, #467, #12617, #20717, #18511, #16548, #10762, #24507, #6721, #6589, #14573, #22555, #716, #18750, #842, #5026, #2934, #17439, #3310, #19265, #23078, #19133, #13141, #1097, #3184, #25289, #23194, #11286, #23453, #3449, #5162, #20989, #979, #1224, #7118, #1488, #11152, #7492, #6981, #13006, #8960, #25168, #9461, #5279, #10896, #9341, #3066, #7249, #15229, #1368, #13255, #15486, #21227, #16935, #15102, #17325, #25406, #9206, #12867, #21106, #20844, #11423, #18896, #17196, #7369, #15346, #13394, #23316, #19397, #21370, #5406, #24904, #14962, #11034, #22939, #19013, #9073, #17056, #25025, #3833, #15617, #21881, #4081, #9845, #17827, #12054, #9585, #3574, #15867, #11675, #23702, #5543, #9970, #13526, #23584, #1612, #16131, #1883, #20036, #2139, #18104, #25798, #9727, #13912, #10102, #11813, #5666, #3694, #11545, #14037, #21752, #17961, #1757, #19651, #19899, #6054, #7756, #16007, #17708 ),
 .UNSPECIFIED., .F., .F. ) 
 B_SPLINE_CURVE_WITH_KNOTS ( ( 3, 2, 2, 2, 2, 2, 2, 2, 2, 2, 2, 2, 2, 2, 2, 2, 2, 2, 2, 2, 2, 2, 2, 2, 2, 2, 2, 2, 2, 2, 2, 2, 2, 2, 2, 2, 2, 2, 2, 2, 2, 2, 2, 2, 2, 2, 2, 2, 2, 2, 2, 2, 2, 2, 2, 2, 2, 2, 2, 2, 3 ),
 ( 0.000000000000000000, 0.01666666666666666644, 0.03333333333333333287, 0.05000000000000000278, 0.06666666666666666574, 0.08333333333333332871, 0.1000000000000000056, 0.1166666666666666685, 0.1333333333333333315, 0.1499999999999999944, 0.1666666666666666574, 0.1833333333333333204, 0.2000000000000000111, 0.2166666666666666741, 0.2333333333333333370, 0.2500000000000000000, 0.2666666666666666630, 0.2833333333333333259, 0.2999999999999999889, 0.3166666666666666519, 0.3333333333333333148, 0.3499999999999999778, 0.3666666666666666408, 0.3833333333333333592, 0.4000000000000000222, 0.4166666666666666852, 0.4333333333333333481, 0.4500000000000000111, 0.4666666666666666741, 0.4833333333333333370, 0.5000000000000000000, 0.5166666666666667185, 0.5333333333333333259, 0.5500000000000000444, 0.5666666666666666519, 0.5833333333333333703, 0.5999999999999999778, 0.6166666666666666963, 0.6333333333333333037, 0.6500000000000000222, 0.6666666666666666297, 0.6833333333333333481, 0.6999999999999999556, 0.7166666666666666741, 0.7333333333333332815, 0.7500000000000000000, 0.7666666666666667185, 0.7833333333333333259, 0.8000000000000000444, 0.8166666666666666519, 0.8333333333333333703, 0.8499999999999999778, 0.8666666666666666963, 0.8833333333333333037, 0.9000000000000000222, 0.9166666666666666297, 0.9333333333333333481, 0.9499999999999999556, 0.9666666666666666741, 0.9833333333333332815, 1.000000000000000000 ),
 .UNSPECIFIED. ) 
 CURVE ( )  GEOMETRIC_REPRESENTATION_ITEM ( )  RATIONAL_B_SPLINE_CURVE ( ( 1.000000000000000000, 0.8660254037844387076, 1.000000000000000000, 0.8660254037844387076, 1.000000000000000000, 0.8660254037844387076, 1.000000000000000000, 0.8660254037844387076, 1.000000000000000000, 0.8660254037844387076, 1.000000000000000000, 0.8660254037844387076, 1.000000000000000000, 0.8660254037844387076, 1.000000000000000000, 0.8660254037844387076, 1.000000000000000000, 0.8660254037844387076, 1.000000000000000000, 0.8660254037844387076, 1.000000000000000000, 0.8660254037844387076, 1.000000000000000000, 0.8660254037844387076, 1.000000000000000000, 0.8660254037844387076, 1.000000000000000000, 0.8660254037844387076, 1.000000000000000000, 0.8660254037844387076, 1.000000000000000000, 0.8660254037844387076, 1.000000000000000000, 0.8660254037844387076, 1.000000000000000000, 0.8660254037844387076, 1.000000000000000000, 0.8660254037844387076, 1.000000000000000000, 0.8660254037844387076, 1.000000000000000000, 0.8660254037844387076, 1.000000000000000000, 0.8660254037844387076, 1.000000000000000000, 0.8660254037844387076, 1.000000000000000000, 0.8660254037844387076, 1.000000000000000000, 0.8660254037844387076, 1.000000000000000000, 0.8660254037844387076, 1.000000000000000000, 0.8660254037844387076, 1.000000000000000000, 0.8660254037844387076, 1.000000000000000000, 0.8660254037844387076, 1.000000000000000000, 0.8660254037844387076, 1.000000000000000000, 0.8660254037844387076, 1.000000000000000000, 0.8660254037844387076, 1.000000000000000000, 0.8660254037844387076, 1.000000000000000000, 0.8660254037844387076, 1.000000000000000000, 0.8660254037844387076, 1.000000000000000000, 0.8660254037844387076, 1.000000000000000000, 0.8660254037844387076, 1.000000000000000000, 0.8660254037844387076, 1.000000000000000000, 0.8660254037844387076, 1.000000000000000000, 0.8660254037844387076, 1.000000000000000000, 0.8660254037844387076, 1.000000000000000000, 0.8660254037844387076, 1.000000000000000000, 0.8660254037844387076, 1.000000000000000000, 0.8660254037844387076, 1.000000000000000000, 0.8660254037844387076, 1.000000000000000000, 0.8660254037844387076, 1.000000000000000000, 0.8660254037844387076, 1.000000000000000000, 0.8660254037844387076, 1.000000000000000000, 0.8660254037844387076, 1.000000000000000000, 0.8660254037844387076, 1.000000000000000000, 0.8660254037844387076, 1.000000000000000000, 0.8660254037844387076, 1.000000000000000000, 0.8660254037844387076, 1.000000000000000000, 0.8660254037844387076, 1.000000000000000000, 0.8660254037844387076, 1.000000000000000000, 0.8660254037844387076, 1.000000000000000000, 0.8660254037844387076, 1.000000000000000000, 0.8660254037844387076, 1.000000000000000000, 0.8660254037844387076, 1.000000000000000000, 0.8660254037844387076, 1.000000000000000000 ) ) 
 REPRESENTATION_ITEM ( '' )  );
#7772=VERTEX_POINT ( 'NONE', #22356 ) ;
#7779=CARTESIAN_POINT ( 'NONE',  ( 3.756430356250002323, 25.55312499938548143, 11.16877607737301226 ) ) ;
#7782=CARTESIAN_POINT ( 'NONE',  ( -3.878215178125003604, -25.32343749907822783, 8.999999999999992895 ) ) ;
#7783=CARTESIAN_POINT ( 'NONE',  ( 22.41528496361359046, 16.75843071412113972, 8.999999999999992895 ) ) ;
#7784=CARTESIAN_POINT ( 'NONE',  ( 18.19682354053567153, 23.50921829645433903, 6.831223922626973533 ) ) ;
#7786=CARTESIAN_POINT ( 'NONE',  ( 0.000000000000000000, 0.000000000000000000, 0.000000000000000000 ) ) ;
#7790=CARTESIAN_POINT ( 'NONE',  ( 18.77930694887276886, 17.26355742102066415, 4.999999999999992006 ) ) ;
#7793=CARTESIAN_POINT ( 'NONE',  ( -4.000000000000003553, -27.28749999999999787, 6.690598923241489970 ) ) ;
#7794=CARTESIAN_POINT ( 'NONE',  ( -4.000000000000003553, -29.89374999877096784, 8.999999999999992895 ) ) ;
#7798=VERTEX_POINT ( 'NONE', #24570 ) ;
#7799=CARTESIAN_POINT ( 'NONE',  ( 3.756430356249996994, -29.41562499938548569, 8.999999999999992895 ) ) ;
#7815=CARTESIAN_POINT ( 'NONE',  ( 20.78451994863305430, 15.12766569914060888, 8.999999999999992895 ) ) ;
#7818=CARTESIAN_POINT ( 'NONE',  ( 0.2644264925860129734, 30.00000000000001421, 4.999999999999992006 ) ) ;
#7820=FACE_OUTER_BOUND ( 'NONE', #9001, .T. ) ;
#7822=LINE ( 'NONE', #9909, #6817 ) ;
#7828=VERTEX_POINT ( 'NONE', #18443 ) ;
#7829=ORIENTED_EDGE ( 'NONE', *, *, #22775, .T. ) ;
#7830=EDGE_CURVE ( 'NONE', #8636, #17199, #16114, .T. ) ;
#7834=CIRCLE ( 'NONE', #22445, 30.00000000000000355 ) ;
#7839=( NAMED_UNIT ( * ) SI_UNIT ( $, .STERADIAN. ) SOLID_ANGLE_UNIT ( ) );
#7840=CARTESIAN_POINT ( 'NONE',  ( 3.756430356250004099, 29.34062499938548640, 6.831223922626973533 ) ) ;
#7844=CARTESIAN_POINT ( 'NONE',  ( -3.469446951953614189E-15, -25.00000000000000000, 8.999999999999992895 ) ) ;
#7847=CARTESIAN_POINT ( 'NONE',  ( -4.000000000000003553, -27.64374999877096784, 8.999999999999992895 ) ) ;
#7848=CARTESIAN_POINT ( 'NONE',  ( 1.878215178125000939, 26.97812499938548569, 12.25316411605952283 ) ) ;
#7849=DIRECTION ( 'NONE',  ( 1.000000000000000000, 0.000000000000000000, 0.000000000000000000 ) ) ;
#7853=ORIENTED_EDGE ( 'NONE', *, *, #16431, .F. ) ;
#7854=CARTESIAN_POINT ( 'NONE',  ( 3.369928719974892281E-15, 25.50624999877096855, 4.999999999999992006 ) ) ;
#7860=CARTESIAN_POINT ( 'NONE',  ( -1.878215178125000939, -27.87812499938548427, 12.25316411605952283 ) ) ;
#7871=CARTESIAN_POINT ( 'NONE',  ( 21.78337204305729458, 19.12717466509784003, 5.746835883940462963 ) ) ;
#7872=EDGE_CURVE ( 'NONE', #20357, #421, #14433, .T. ) ;
#7874=VECTOR ( 'NONE', #2394, 1000.000000000000000 ) ;
#7877=CARTESIAN_POINT ( 'NONE',  ( 2.000000000000003997, 27.32500000000000284, 5.535898384862238508 ) ) ;
#7886=CARTESIAN_POINT ( 'NONE',  ( -3.999999999999996003, 29.18124999877096926, 6.690598923241487306 ) ) ;
#7892=CIRCLE ( 'NONE', #9555, 26.00000000000000355 ) ;
#7893=CARTESIAN_POINT ( 'NONE',  ( -3.834746474454188013E-15, -25.56250000000000000, 4.999999999999992006 ) ) ;
#7895=VERTEX_POINT ( 'NONE', #16360 ) ;
#7903=ADVANCED_FACE ( 'NONE', ( #11357 ), #9278, .T. ) ;
#7905=CARTESIAN_POINT ( 'NONE',  ( 1.878215178125000939, 26.41562499938548214, 12.25316411605952283 ) ) ;
#7911=CARTESIAN_POINT ( 'NONE',  ( 20.62984034111755705, 17.80141321637130147, 12.46410161513774817 ) ) ;
#7912=CARTESIAN_POINT ( 'NONE',  ( 21.14697593998939595, 18.49077856202994852, 5.746835883940462963 ) ) ;
#7913=CARTESIAN_POINT ( 'NONE',  ( -3.579383266608310077, -29.78592973091716800, 10.80044967790457378 ) ) ;
#7919=EDGE_LOOP ( 'NONE', ( #6516, #10690, #14412, #16645 ) ) ;
#7921=CARTESIAN_POINT ( 'NONE',  ( 3.999999999999996003, -27.43750000000000000, 6.690598923241487306 ) ) ;
#7928=EDGE_LOOP ( 'NONE', ( #15918, #13825, #1953, #18529 ) ) ;
#7930=ORIENTED_EDGE ( 'NONE', *, *, #7229, .T. ) ;
#7934=AXIS2_PLACEMENT_3D ( 'NONE', #20218, #6753, #20744 ) ;
#7948=CARTESIAN_POINT ( 'NONE',  ( 19.74153744638290320, 16.91311032163664407, 5.535898384862238508 ) ) ;
#7949=ORIENTED_EDGE ( 'NONE', *, *, #22393, .T. ) ;
#7960=CARTESIAN_POINT ( 'NONE',  ( 4.000000000000003553, 25.84374999877096712, 8.999999999999992895 ) ) ;
#7962=CARTESIAN_POINT ( 'NONE',  ( -4.000000000000003553, -26.38750000000000284, 6.690598923241489970 ) ) ;
#7973=FACE_OUTER_BOUND ( 'NONE', #11304, .T. ) ;
#7979=CARTESIAN_POINT ( 'NONE',  ( -3.756430356249997882, 28.66562499938548569, 11.16877607737301226 ) ) ;
#7985=DIRECTION ( 'NONE',  ( 0.000000000000000000, 0.000000000000000000, -1.000000000000000000 ) ) ;
#7986=CARTESIAN_POINT ( 'NONE',  ( 4.000000000000001776, 25.80624999877096926, 11.30940107675849760 ) ) ;
#7988=CARTESIAN_POINT ( 'NONE',  ( -3.752267015613588906E-15, -29.55624999877096926, 4.381197846482986158 ) ) ;
#7990=CARTESIAN_POINT ( 'NONE',  ( 1.878215178125000939, 28.32812499938548711, 12.25316411605952283 ) ) ;
#7993=EDGE_CURVE ( 'NONE', #8636, #5294, #23255, .T. ) ;
#8001=FACE_OUTER_BOUND ( 'NONE', #1594, .T. ) ;
#8003=CARTESIAN_POINT ( 'NONE',  ( -2.672651547586948120E-15, -26.82812499938548356, 13.33755215474602984 ) ) ;
#8006=AXIS2_PLACEMENT_3D ( 'NONE', #20972, #11021, #19002 ) ;
#8009=CARTESIAN_POINT ( 'NONE',  ( 2.672651547586948120E-15, 27.39062499938548356, 13.33755215474603162 ) ) ;
#8014=CARTESIAN_POINT ( 'NONE',  ( 21.06742642710591440, 18.41122904914646341, 5.746835883940462963 ) ) ;
#8016=EDGE_CURVE ( 'NONE', #6983, #14487, #18957, .T. ) ;
#8018=CARTESIAN_POINT ( 'NONE',  ( 4.000000000000001776, 27.21250000000000213, 11.30940107675849760 ) ) ;
#8025=ORIENTED_EDGE ( 'NONE', *, *, #4105, .F. ) ;
#8030=CARTESIAN_POINT ( 'NONE',  ( -26.00000000000000355, 0.000000000000000000, 19.59999999999999787 ) ) ;
#8031=CARTESIAN_POINT ( 'NONE',  ( 3.735045420075836212E-15, 25.81562499938548783, 4.662447845253954171 ) ) ;
#8032=CARTESIAN_POINT ( 'NONE',  ( 15.57844627214710975, 21.23530052163942372, 6.690598923241487306 ) ) ;
#8034=CARTESIAN_POINT ( 'NONE',  ( 18.67203843983824996, 18.67203843983818246, 4.999999999999991118 ) ) ;
#8042=CARTESIAN_POINT ( 'NONE',  ( 4.000000000000003553, 29.05000000000000071, 8.999999999999992895 ) ) ;
#8045=CARTESIAN_POINT ( 'NONE',  ( 2.000000000000003997, 29.51874999877096784, 5.535898384862238508 ) ) ;
#8049=CARTESIAN_POINT ( 'NONE',  ( 3.756430356250004099, 25.17812499938548498, 6.831223922626973533 ) ) ;
#8053=CARTESIAN_POINT ( 'NONE',  ( 17.32411613907045478, 20.15254326381657535, 5.535898384862237620 ) ) ;
#8054=CYLINDRICAL_SURFACE ( 'NONE', #12640, 4.000000000000000000 ) ;
#8056=DIRECTION ( 'NONE',  ( 0.000000000000000000, 0.000000000000000000, -1.000000000000000000 ) ) ;
#8057=CARTESIAN_POINT ( 'NONE',  ( -1.999999999999998224, 29.29374999877096997, 12.46410161513774639 ) ) ;
#8059=CARTESIAN_POINT ( 'NONE',  ( 19.10065816080342671, 21.75685553876272493, 5.746835883940462963 ) ) ;
#8062=CARTESIAN_POINT ( 'NONE',  ( -2.620986760973688460E-15, -27.58750000000000213, 13.61880215351699874 ) ) ;
#8070=PLANE ( 'NONE',  #18833 ) ;
#8071=VERTEX_POINT ( 'NONE', #19199 ) ;
#8072=VERTEX_POINT ( 'NONE', #14783 ) ;
#8075=CARTESIAN_POINT ( 'NONE',  ( -1.859271017917182139E-15, -28.88124999877096499, 12.99999999999999289 ) ) ;
#8078=CARTESIAN_POINT ( 'NONE',  ( 3.469446951953614189E-15, 30.00000000000000355, 4.999999999999992006 ) ) ;
#8080=FACE_BOUND ( 'NONE', #9536, .T. ) ;
#8086=CARTESIAN_POINT ( 'NONE',  ( 16.53304042674895058, 22.18989467624125922, 6.690598923241487306 ) ) ;
#8088=DIRECTION ( 'NONE',  ( 0.000000000000000000, 0.000000000000000000, 1.000000000000000000 ) ) ;
#8093=( GEOMETRIC_REPRESENTATION_CONTEXT ( 3 ) GLOBAL_UNCERTAINTY_ASSIGNED_CONTEXT ( ( #4713 ) ) GLOBAL_UNIT_ASSIGNED_CONTEXT ( ( #3407, #17407, #5364 ) ) REPRESENTATION_CONTEXT ( 'NONE', 'WORKASPACE' ) );
#8097=LINE ( 'NONE', #511, #78 ) ;
#8101=DIRECTION ( 'NONE',  ( -0.7071067811865487940, -0.7071067811865463515, 0.000000000000000000 ) ) ;
#8103=EDGE_CURVE ( 'NONE', #7056, #20899, #25732, .T. ) ;
#8116=CARTESIAN_POINT ( 'NONE',  ( 3.756430356250002323, 26.45312499938548356, 11.16877607737301226 ) ) ;
#8121=CARTESIAN_POINT ( 'NONE',  ( 1.071796769724487230, -25.52634618820330559, 4.999999999999992006 ) ) ;
#8123=CARTESIAN_POINT ( 'NONE',  ( 1.999999999999995781, -28.24374999877096570, 5.535898384862237620 ) ) ;
#8124=CARTESIAN_POINT ( 'NONE',  ( 1.878215178125004048, 28.92812499938548854, 5.746835883940462963 ) ) ;
#8127=ORIENTED_EDGE ( 'NONE', *, *, #20142, .T. ) ;
#8136=EDGE_LOOP ( 'NONE', ( #25861, #25686, #4068, #133 ) ) ;
#8140=CARTESIAN_POINT ( 'NONE',  ( 3.756430356250003211, 27.09062499938548640, 6.831223922626973533 ) ) ;
#8141=ADVANCED_FACE ( 'NONE', ( #5855 ), #23438, .F. ) ;
#8144=CARTESIAN_POINT ( 'NONE',  ( 20.74922837557196331, 18.09303099761251588, 5.746835883940462963 ) ) ;
#8148=CARTESIAN_POINT ( 'NONE',  ( 4.000000000000003553, 27.25000000000000000, 8.999999999999992895 ) ) ;
#8158=CARTESIAN_POINT ( 'NONE',  ( -3.756430356249995661, 25.89062499938548356, 6.831223922626973533 ) ) ;
#8159=CARTESIAN_POINT ( 'NONE',  ( 16.96614333022570875, 19.79457045497182577, 5.535898384862237620 ) ) ;
#8161=ORIENTED_EDGE ( 'NONE', *, *, #7141, .F. ) ;
#8165=ADVANCED_FACE ( 'NONE', ( #24610 ), #8054, .F. ) ;
#8174=CARTESIAN_POINT ( 'NONE',  ( -4.000000000000003553, -29.69687499938548569, 8.999999999999992895 ) ) ;
#8180=CARTESIAN_POINT ( 'NONE',  ( 21.00669330961039449, 19.49094378175826847, 4.999999999999992895 ) ) ;
#8181=CARTESIAN_POINT ( 'NONE',  ( 3.756430356249996105, -25.77812499938548285, 6.831223922626973533 ) ) ;
#8185=CARTESIAN_POINT ( 'NONE',  ( 3.999999999999996447, -28.82499999999999929, 8.999999999999992895 ) ) ;
#8190=DIRECTION ( 'NONE',  ( -0.7071067811865487940, -0.7071067811865463515, -0.000000000000000000 ) ) ;
#8196=CARTESIAN_POINT ( 'NONE',  ( 3.959305671612554781E-15, 30.00000000000000355, 12.99999999999999289 ) ) ;
#8206=CARTESIAN_POINT ( 'NONE',  ( 21.10271800016700183, 15.44586375067455464, 8.999999999999992895 ) ) ;
#8208=CARTESIAN_POINT ( 'NONE',  ( 20.32496430686003208, 17.66876692890059530, 12.25316411605952283 ) ) ;
#8209=CARTESIAN_POINT ( 'NONE',  ( 16.85123847828289811, 22.50809272777520675, 6.690598923241487306 ) ) ;
#8214=CARTESIAN_POINT ( 'NONE',  ( -3.595210675795415867, 29.78396494222454294, 7.227341970420264161 ) ) ;
#8219=DIRECTION ( 'NONE',  ( -0.000000000000000000, 1.000000000000000000, -0.000000000000000000 ) ) ;
#8221=CARTESIAN_POINT ( 'NONE',  ( -3.735045420075836212E-15, -27.05312499938548498, 4.662447845253954171 ) ) ;
#8224=ORIENTED_EDGE ( 'NONE', *, *, #13962, .T. ) ;
#8225=ORIENTED_EDGE ( 'NONE', *, *, #8423, .F. ) ;
#8235=CARTESIAN_POINT ( 'NONE',  ( -3.756430356249996994, 26.71562499938548285, 8.999999999999992895 ) ) ;
#8243=CARTESIAN_POINT ( 'NONE',  ( -3.752267015613588906E-15, -28.20624999877096784, 4.381197846482986158 ) ) ;
#8245=CARTESIAN_POINT ( 'NONE',  ( 2.672651547586948120E-15, 29.64062499938548356, 13.33755215474602984 ) ) ;
#8246=CARTESIAN_POINT ( 'NONE',  ( -3.469446951953614189E-15, -30.00000000000000355, 4.999999999999992006 ) ) ;
#8248=CARTESIAN_POINT ( 'NONE',  ( 3.974466138550253103, -29.73560671006806899, 8.477544402765669673 ) ) ;
#8249=ORIENTED_EDGE ( 'NONE', *, *, #23882, .T. ) ;
#8256=VERTEX_POINT ( 'NONE', #20194 ) ;
#8257=ORIENTED_EDGE ( 'NONE', *, *, #8562, .T. ) ;
#8261=CARTESIAN_POINT ( 'NONE',  ( 3.756430356250003655, 26.60312499938548569, 8.999999999999992895 ) ) ;
#8264=CARTESIAN_POINT ( 'NONE',  ( 21.06969990136081705, 15.75730514544200211, 8.999999999999992895 ) ) ;
#8270=CARTESIAN_POINT ( 'NONE',  ( 2.000000000000000888, 29.42500000000000071, 12.46410161513774817 ) ) ;
#8273=DIRECTION ( 'NONE',  ( 0.000000000000000000, 1.000000000000000000, 0.000000000000000000 ) ) ;
#8274=CARTESIAN_POINT ( 'NONE',  ( -1.071796769724498999, -28.05759618943233491, 12.99999999999998757 ) ) ;
#8283=CARTESIAN_POINT ( 'NONE',  ( 21.44743255599544440, 15.79057830650299366, 6.690598923241489970 ) ) ;
#8292=CARTESIAN_POINT ( 'NONE',  ( -25.99307600111999150, -0.5999999999999996447, 19.00000000000000000 ) ) ;
#8295=CARTESIAN_POINT ( 'NONE',  ( -3.756430356249996994, 28.06562499938548427, 8.999999999999992895 ) ) ;
#8300=CARTESIAN_POINT ( 'NONE',  ( 22.00869856443133088, 19.18027143968506465, 5.535898384862238508 ) ) ;
#8309=CARTESIAN_POINT ( 'NONE',  ( 22.37551020630278842, 16.71865595681033412, 8.999999999999992895 ) ) ;
#8317=CARTESIAN_POINT ( 'NONE',  ( 3.756430356249996994, -26.37812499938548783, 8.999999999999992895 ) ) ;
#8319=CARTESIAN_POINT ( 'NONE',  ( 1.071796769724494558, 28.18615380933863435, 4.999999999999992895 ) ) ;
#8320=VECTOR ( 'NONE', #11429, 1000.000000000000000 ) ;
#8324=DIRECTION ( 'NONE',  ( -0.8660254037844397068, -0.4999999999999983347, 0.000000000000000000 ) ) ;
#8332=CARTESIAN_POINT ( 'NONE',  ( 21.04318339706631846, 15.73078864114750530, 11.16877607737301226 ) ) ;
#8333=CARTESIAN_POINT ( 'NONE',  ( 21.22646168687465007, 18.39803456212839450, 12.46410161513774817 ) ) ;
#8334=ORIENTED_EDGE ( 'NONE', *, *, #15730, .F. ) ;
#8335=CARTESIAN_POINT ( 'NONE',  ( 3.999999999999995559, -26.98750000000000071, 6.690598923241487306 ) ) ;
#8341=CARTESIAN_POINT ( 'NONE',  ( 20.77801835412136100, 15.46562359820254784, 6.831223922626973533 ) ) ;
#8342=DIRECTION ( 'NONE',  ( 0.9659258262890673130, -0.2588190451025242922, 0.000000000000000000 ) ) ;
#8344=DIRECTION ( 'NONE',  ( 0.000000000000000000, 0.000000000000000000, 1.000000000000000000 ) ) ;
#8345=CARTESIAN_POINT ( 'NONE',  ( 2.000000000000003997, 25.91874999877096997, 5.535898384862238508 ) ) ;
#8346=CARTESIAN_POINT ( 'NONE',  ( -3.756430356250004099, -26.07812499938548356, 6.831223922626973533 ) ) ;
#8352=ORIENTED_EDGE ( 'NONE', *, *, #14474, .T. ) ;
#8353=EDGE_CURVE ( 'NONE', #13915, #7056, #21602, .T. ) ;
#8359=AXIS2_PLACEMENT_3D ( 'NONE', #17238, #9380, #11070 ) ;
#8362=CARTESIAN_POINT ( 'NONE',  ( -3.756430356249996994, 27.16562499938548214, 8.999999999999992895 ) ) ;
#8363=VECTOR ( 'NONE', #18984, 1000.000000000000000 ) ;
#8369=CARTESIAN_POINT ( 'NONE',  ( -1.999999999999998224, 28.84374999877096712, 12.46410161513774639 ) ) ;
#8370=CARTESIAN_POINT ( 'NONE',  ( -3.756430356250004099, -25.74062499938548143, 6.831223922626973533 ) ) ;
#8375=CARTESIAN_POINT ( 'NONE',  ( 1.999999999999998224, -25.30000000000000426, 12.46410161513774639 ) ) ;
#8376=ORIENTED_EDGE ( 'NONE', *, *, #9576, .F. ) ;
#8386=ORIENTED_EDGE ( 'NONE', *, *, #2089, .F. ) ;
#8393=CARTESIAN_POINT ( 'NONE',  ( 3.756430356250003211, 27.54062499938547859, 6.831223922626973533 ) ) ;
#8394=( BOUNDED_CURVE ( )  B_SPLINE_CURVE ( 2, ( #8552, #17971, #10232, #18229, #312, #8283, #12335, #16265, #8034 ),
 .UNSPECIFIED., .F., .F. ) 
 B_SPLINE_CURVE_WITH_KNOTS ( ( 3, 2, 2, 2, 3 ),
 ( 0.1750000000000000167, 0.1833333333333333204, 0.2000000000000000111, 0.2166666666666666741, 0.2250000000000000056 ),
 .UNSPECIFIED. ) 
 CURVE ( )  GEOMETRIC_REPRESENTATION_ITEM ( )  RATIONAL_B_SPLINE_CURVE ( ( 0.9330127018922194093, 0.9330127018922196314, 1.000000000000000000, 0.8660254037844387076, 1.000000000000000000, 0.8660254037844387076, 1.000000000000000000, 0.9330127018922194093, 0.9330127018922194093 ) ) 
 REPRESENTATION_ITEM ( '' )  );
#8399=CARTESIAN_POINT ( 'NONE',  ( 22.31597560320210505, 17.00358084728328478, 11.16877607737301226 ) ) ;
#8407=CARTESIAN_POINT ( 'NONE',  ( 3.756430356250002323, 28.25312499938548427, 11.16877607737301403 ) ) ;
#8411=CARTESIAN_POINT ( 'NONE',  ( -4.000000000000001776, -28.11250000000000071, 11.30940107675849760 ) ) ;
#8418=EDGE_CURVE ( 'NONE', #4092, #18554, #5565, .T. ) ;
#8420=CARTESIAN_POINT ( 'NONE',  ( -3.999999999999997335, 26.16250000000000142, 11.30940107675849404 ) ) ;
#8423=EDGE_CURVE ( 'NONE', #5410, #21566, #3047, .T. ) ;
#8435=CARTESIAN_POINT ( 'NONE',  ( -1.878215178124995832, 27.99062499938548143, 5.746835883940462963 ) ) ;
#8439=CARTESIAN_POINT ( 'NONE',  ( 17.84560739019553921, 23.50246163968784430, 6.690598923241487306 ) ) ;
#8440=CARTESIAN_POINT ( 'NONE',  ( -1.071796769724493448, 29.18259618943233136, 4.999999999999995559 ) ) ;
#8441=CARTESIAN_POINT ( 'NONE',  ( -3.834746474454188013E-15, -27.75624999877096855, 4.999999999999992006 ) ) ;
#8447=CARTESIAN_POINT ( 'NONE',  ( 3.999999999999996447, -28.37500000000000000, 8.999999999999992895 ) ) ;
#8452=CARTESIAN_POINT ( 'NONE',  ( 1.057460391440397258E-14, -29.10624999877096641, 4.999999999999992006 ) ) ;
#8456=VERTEX_POINT ( 'NONE', #7089 ) ;
#8457=EDGE_LOOP ( 'NONE', ( #21614, #21990, #18999, #1597 ) ) ;
#8458=CARTESIAN_POINT ( 'NONE',  ( 1.878215178124995832, -27.65312499938548640, 5.746835883940462963 ) ) ;
#8460=CARTESIAN_POINT ( 'NONE',  ( -1.626862140677534194E-14, -28.03750000000000497, 12.99999999999999289 ) ) ;
#8461=EDGE_CURVE ( 'NONE', #12953, #14487, #17668, .T. ) ;
#8462=CARTESIAN_POINT ( 'NONE',  ( 3.469446951953614189E-15, 30.00000000000000355, 4.999999999999992006 ) ) ;
#8467=LINE ( 'NONE', #18541, #16348 ) ;
#8471=CARTESIAN_POINT ( 'NONE',  ( 17.61573392031167273, 20.27193129827097806, 12.25316411605951927 ) ) ;
#8472=CARTESIAN_POINT ( 'NONE',  ( 23.62178590814407642, 17.96493165865162567, 11.30940107675849760 ) ) ;
#8473=CARTESIAN_POINT ( 'NONE',  ( -1.071796769724488563, 28.46740381056766722, 12.99999999999999289 ) ) ;
#8481=ORIENTED_EDGE ( 'NONE', *, *, #18899, .T. ) ;
#8483=CARTESIAN_POINT ( 'NONE',  ( 2.620986760973688460E-15, 25.73124999877096997, 13.61880215351699874 ) ) ;
#8484=CARTESIAN_POINT ( 'NONE',  ( -3.735045420075836212E-15, -27.50312499938548783, 4.662447845253954171 ) ) ;
#8490=CARTESIAN_POINT ( 'NONE',  ( -3.756430356250002323, -25.55312499938548143, 11.16877607737301226 ) ) ;
#8491=VERTEX_POINT ( 'NONE', #21341 ) ;
#8492=VERTEX_POINT ( 'NONE', #25522 ) ;
#8495=STYLED_ITEM('',(#25907),#4848);
#8502=CARTESIAN_POINT ( 'NONE',  ( -4.000000000000003553, -29.50000000000000355, 8.999999999999992895 ) ) ;
#8503=CARTESIAN_POINT ( 'NONE',  ( 3.756430356250003655, 25.59062499938548285, 8.999999999999992895 ) ) ;
#8505=LINE ( 'NONE', #12685, #22171 ) ;
#8509=CARTESIAN_POINT ( 'NONE',  ( 22.54985889724113335, 19.78820606519062508, 12.50294890599016639 ) ) ;
#8512=CARTESIAN_POINT ( 'NONE',  ( 1.878215178124995832, -27.65312499938548640, 5.746835883940462963 ) ) ;
#8515=CARTESIAN_POINT ( 'NONE',  ( 19.03001124868299243, 19.03001124868293559, 4.999999999999991118 ) ) ;
#8528=VERTEX_POINT ( 'NONE', #1728 ) ;
#8529=DIRECTION ( 'NONE',  ( 0.000000000000000000, 0.000000000000000000, 1.000000000000000000 ) ) ;
#8530=CARTESIAN_POINT ( 'NONE',  ( 3.756430356250003655, 28.85312499938548569, 8.999999999999992895 ) ) ;
#8534=CARTESIAN_POINT ( 'NONE',  ( 15.88988766691455368, 21.20228242283322828, 6.831223922626973533 ) ) ;
#8544=CARTESIAN_POINT ( 'NONE',  ( -2.000000000000003997, -28.16874999877096997, 5.535898384862238508 ) ) ;
#8545=ORIENTED_EDGE ( 'NONE', *, *, #15223, .F. ) ;
#8546=ORIENTED_EDGE ( 'NONE', *, *, #1970, .T. ) ;
#8552=CARTESIAN_POINT ( 'NONE',  ( 18.51293941407127974, 18.51293941407120869, 12.99999999999999112 ) ) ;
#8559=CARTESIAN_POINT ( 'NONE',  ( -3.469446951953614189E-15, -30.00000000000000355, 8.999999999999992895 ) ) ;
#8560=CARTESIAN_POINT ( 'NONE',  ( 17.67766952966372429, 17.67766952966365324, 12.99999999999999289 ) ) ;
#8561=CARTESIAN_POINT ( 'NONE',  ( 17.93620544610052647, 17.93620544610046252, 4.662447845253954171 ) ) ;
#8562=EDGE_CURVE ( 'NONE', #2329, #1175, #21980, .T. ) ;
#8563=CARTESIAN_POINT ( 'NONE',  ( 3.756430356250004099, 28.77812499938548285, 6.831223922626973533 ) ) ;
#8566=CARTESIAN_POINT ( 'NONE',  ( 20.30280345481878967, 20.30280345481871151, 4.381197846482986158 ) ) ;
#8568=EDGE_CURVE ( 'NONE', #20899, #21834, #17103, .T. ) ;
#8570=CARTESIAN_POINT ( 'NONE',  ( 3.756430356249997438, -28.10312499938548569, 11.16877607737301048 ) ) ;
#8575=CARTESIAN_POINT ( 'NONE',  ( -4.000000000000003553, -29.08750000000000213, 6.690598923241489970 ) ) ;
#8577=ORIENTED_EDGE ( 'NONE', *, *, #21163, .F. ) ;
#8578=ORIENTED_EDGE ( 'NONE', *, *, #17040, .T. ) ;
#8582=VERTEX_POINT ( 'NONE', #9942 ) ;
#8583=CARTESIAN_POINT ( 'NONE',  ( 3.756430356249996994, -27.27812499938548640, 8.999999999999992895 ) ) ;
#8585=DIRECTION ( 'NONE',  ( -1.000000000000000000, -0.000000000000000000, -0.000000000000000000 ) ) ;
#8592=CARTESIAN_POINT ( 'NONE',  ( 4.000000000000001776, 25.41250000000000142, 11.30940107675849760 ) ) ;
#8593=CARTESIAN_POINT ( 'NONE',  ( 20.96136040992792715, 18.30516303196848327, 12.25316411605952283 ) ) ;
#8594=CARTESIAN_POINT ( 'NONE',  ( 19.62663259444009611, 19.62663259444002151, 4.381197846482986158 ) ) ;
#8600=CARTESIAN_POINT ( 'NONE',  ( 19.15823811790222919, 16.50204073994278531, 5.746835883940462963 ) ) ;
#8602=CIRCLE ( 'NONE', #249, 26.00000000000000355 ) ;
#8605=CARTESIAN_POINT ( 'NONE',  ( 4.000000000000003553, 27.68124999877096926, 6.690598923241489970 ) ) ;
#8606=CARTESIAN_POINT ( 'NONE',  ( 1.878215178124998497, -25.89062499938548356, 12.25316411605951927 ) ) ;
#8610=EDGE_CURVE ( 'NONE', #11941, #8582, #20442, .T. ) ;
#8612=CARTESIAN_POINT ( 'NONE',  ( 3.756430356249997882, -26.30312499938548498, 11.16877607737301226 ) ) ;
#8614=APPLICATION_CONTEXT ( 'automotive_design' ) ;
#8615=ORIENTED_EDGE ( 'NONE', *, *, #22350, .T. ) ;
#8618=CARTESIAN_POINT ( 'NONE',  ( 4.000000000000003553, 27.70000000000000284, 8.999999999999992895 ) ) ;
#8619=( BOUNDED_CURVE ( )  B_SPLINE_CURVE ( 2, ( #9548, #21197, #9307, #25642, #9167, #15198, #11389, #7723, #17292 ),
 .UNSPECIFIED., .F., .F. ) 
 B_SPLINE_CURVE_WITH_KNOTS ( ( 3, 2, 2, 2, 3 ),
 ( 0.9249999999999999334, 0.9333333333333333481, 0.9499999999999999556, 0.9666666666666666741, 0.9749999999999999778 ),
 .UNSPECIFIED. ) 
 CURVE ( )  GEOMETRIC_REPRESENTATION_ITEM ( )  RATIONAL_B_SPLINE_CURVE ( ( 0.9330127018922194093, 0.9330127018922189652, 1.000000000000000000, 0.8660254037844387076, 1.000000000000000000, 0.8660254037844387076, 1.000000000000000000, 0.9330127018922194093, 0.9330127018922194093 ) ) 
 REPRESENTATION_ITEM ( '' )  );
#8622=CARTESIAN_POINT ( 'NONE',  ( -4.000000000000001776, -27.15624999877097423, 11.30940107675849760 ) ) ;
#8623=CARTESIAN_POINT ( 'NONE',  ( 3.756430356250003655, 26.04062499938548569, 8.999999999999992895 ) ) ;
#8624=CARTESIAN_POINT ( 'NONE',  ( 18.50088365464961626, 16.98513412679750090, 4.999999999999992006 ) ) ;
#8625=CARTESIAN_POINT ( 'NONE',  ( -1.859271017917182139E-15, -28.93749999999999645, 12.99999999999999289 ) ) ;
#8630=CARTESIAN_POINT ( 'NONE',  ( 1.878215178124995832, -27.20312499938548711, 5.746835883940462963 ) ) ;
#8631=CARTESIAN_POINT ( 'NONE',  ( 1.878215178125000939, 29.67812499938548498, 12.25316411605952283 ) ) ;
#8632=CARTESIAN_POINT ( 'NONE',  ( -8.831537335106614961E-15, -26.23749999999999716, 12.99999999999999112 ) ) ;
#8636=VERTEX_POINT ( 'NONE', #10454 ) ;
#8640=ORIENTED_EDGE ( 'NONE', *, *, #10574, .F. ) ;
#8648=CARTESIAN_POINT ( 'NONE',  ( 3.756430356250003211, 28.89062499938548356, 6.831223922626973533 ) ) ;
#8650=CARTESIAN_POINT ( 'NONE',  ( 21.59775651299582222, 18.94155913503637478, 12.25316411605952283 ) ) ;
#8652=CARTESIAN_POINT ( 'NONE',  ( -3.403349963601427053, -25.83240171513484640, 20.00001199999999812 ) ) ;
#8665=ADVANCED_FACE ( 'NONE', ( #22362 ), #24720, .T. ) ;
#8672=DIRECTION ( 'NONE',  ( 0.000000000000000000, 0.000000000000000000, 1.000000000000000000 ) ) ;
#8674=ADVANCED_FACE ( 'NONE', ( #6414 ), #785, .T. ) ;
#8677=DIRECTION ( 'NONE',  ( 0.000000000000000000, -1.000000000000000000, 0.000000000000000000 ) ) ;
#8678=DIRECTION ( 'NONE',  ( 0.000000000000000000, 0.000000000000000000, -1.000000000000000000 ) ) ;
#8681=CARTESIAN_POINT ( 'NONE',  ( -3.756430356249996994, 28.51562499938548356, 8.999999999999992895 ) ) ;
#8686=CARTESIAN_POINT ( 'NONE',  ( 1.878215178124998497, -27.24062499938548498, 12.25316411605951927 ) ) ;
#8691=CARTESIAN_POINT ( 'NONE',  ( 20.23961848442275269, 18.72386895657063377, 12.99999999999999112 ) ) ;
#8692=CARTESIAN_POINT ( 'NONE',  ( 19.94483064597403654, 19.94483064597395838, 4.999999999999992006 ) ) ;
#8698=VERTEX_POINT ( 'NONE', #22636 ) ;
#8699=EDGE_CURVE ( 'NONE', #5581, #13483, #22240, .T. ) ;
#8700=CARTESIAN_POINT ( 'NONE',  ( -2.672651547586948120E-15, -26.49062499938548498, 13.33755215474603162 ) ) ;
#8703=EDGE_CURVE ( 'NONE', #6938, #23711, #13523, .T. ) ;
#8706=CARTESIAN_POINT ( 'NONE',  ( 21.19421263902459529, 19.67846311117246927, 12.99999999999999467 ) ) ;
#8712=CARTESIAN_POINT ( 'NONE',  ( -3.756430356249997438, 25.40312499938548285, 11.16877607737301048 ) ) ;
#8713=CARTESIAN_POINT ( 'NONE',  ( 3.999999999999996447, -28.31874999877096855, 8.999999999999992895 ) ) ;
#8714=CARTESIAN_POINT ( 'NONE',  ( 19.92494326818769323, 19.92494326818762218, 13.33755215474602984 ) ) ;
#8715=CARTESIAN_POINT ( 'NONE',  ( 15.38607408531914089, 20.69846884123782260, 11.16877607737301226 ) ) ;
#8722=CARTESIAN_POINT ( 'NONE',  ( 0.000000000000000000, 10.00000000000000000, 15.00000000000000178 ) ) ;
#8725=CARTESIAN_POINT ( 'NONE',  ( 3.752267015613588906E-15, 27.30624999877097281, 4.381197846482986158 ) ) ;
#8726=CARTESIAN_POINT ( 'NONE',  ( -1.878215178125004048, -26.11562499938548498, 5.746835883940462963 ) ) ;
#8728=VERTEX_POINT ( 'NONE', #3249 ) ;
#8733=CARTESIAN_POINT ( 'NONE',  ( -1.878215178125000939, -25.51562499938548356, 12.25316411605952283 ) ) ;
#8734=VERTEX_POINT ( 'NONE', #7054 ) ;
#8745=CARTESIAN_POINT ( 'NONE',  ( 3.756430356250004099, 27.87812499938548427, 6.831223922626973533 ) ) ;
#8751=CARTESIAN_POINT ( 'NONE',  ( 18.88296798233768214, 20.39871751018965895, 4.999999999999992006 ) ) ;
#8754=CARTESIAN_POINT ( 'NONE',  ( 3.756430356249997882, -26.41562499938548569, 11.16877607737301226 ) ) ;
#8765=( BOUNDED_CURVE ( )  B_SPLINE_CURVE ( 2, ( #10952, #20501, #12032, #4817, #22464, #24825, #23954, #1025, #4690 ),
 .UNSPECIFIED., .F., .F. ) 
 B_SPLINE_CURVE_WITH_KNOTS ( ( 3, 2, 2, 2, 3 ),
 ( 0.2250000000000000056, 0.2333333333333333370, 0.2500000000000000000, 0.2666666666666666630, 0.2750000000000000222 ),
 .UNSPECIFIED. ) 
 CURVE ( )  GEOMETRIC_REPRESENTATION_ITEM ( )  RATIONAL_B_SPLINE_CURVE ( ( 0.9330127018922194093, 0.9330127018922194093, 1.000000000000000000, 0.8660254037844387076, 1.000000000000000000, 0.8660254037844387076, 1.000000000000000000, 0.9330127018922191873, 0.9330127018922194093 ) ) 
 REPRESENTATION_ITEM ( '' )  );
#8769=ORIENTED_EDGE ( 'NONE', *, *, #20034, .F. ) ;
#8773=( BOUNDED_CURVE ( )  B_SPLINE_CURVE ( 2, ( #7310, #25475, #15549, #5469, #1427, #9780, #17760, #11738, #23385 ),
 .UNSPECIFIED., .F., .F. ) 
 B_SPLINE_CURVE_WITH_KNOTS ( ( 3, 2, 2, 2, 3 ),
 ( 0.3250000000000000111, 0.3333333333333333148, 0.3499999999999999778, 0.3666666666666666408, 0.3750000000000000000 ),
 .UNSPECIFIED. ) 
 CURVE ( )  GEOMETRIC_REPRESENTATION_ITEM ( )  RATIONAL_B_SPLINE_CURVE ( ( 0.9330127018922194093, 0.9330127018922196314, 1.000000000000000000, 0.8660254037844387076, 1.000000000000000000, 0.8660254037844387076, 1.000000000000000000, 0.9330127018922194093, 0.9330127018922194093 ) ) 
 REPRESENTATION_ITEM ( '' )  );
#8777=CARTESIAN_POINT ( 'NONE',  ( -3.756430356249996994, 27.72812499938548569, 8.999999999999992895 ) ) ;
#8782=CARTESIAN_POINT ( 'NONE',  ( 19.52492222951535439, 22.18111960747465261, 12.25316411605951927 ) ) ;
#8783=DIRECTION ( 'NONE',  ( 0.000000000000000000, 0.000000000000000000, -1.000000000000000000 ) ) ;
#8786=VECTOR ( 'NONE', #19210, 1000.000000000000000 ) ;
#8788=DIRECTION ( 'NONE',  ( -0.8660254037844397068, 0.4999999999999983347, 0.000000000000000000 ) ) ;
#8789=DIRECTION ( 'NONE',  ( 0.000000000000000000, 0.000000000000000000, -1.000000000000000000 ) ) ;
#8790=LINE ( 'NONE', #24482, #18447 ) ;
#8797=ORIENTED_EDGE ( 'NONE', *, *, #12468, .F. ) ;
#8800=ORIENTED_EDGE ( 'NONE', *, *, #12347, .T. ) ;
#8801=DIRECTION ( 'NONE',  ( 0.000000000000000000, 0.000000000000000000, -1.000000000000000000 ) ) ;
#8803=CARTESIAN_POINT ( 'NONE',  ( 3.756430356249996994, -26.37812499938548783, 8.999999999999992895 ) ) ;
#8807=ORIENTED_EDGE ( 'NONE', *, *, #11521, .F. ) ;
#8813=EDGE_CURVE ( 'NONE', #1657, #22706, #19774, .T. ) ;
#8816=CARTESIAN_POINT ( 'NONE',  ( 19.55598568231966539, 16.89978830436022150, 5.746835883940462963 ) ) ;
#8817=VECTOR ( 'NONE', #8190, 1000.000000000000000 ) ;
#8820=CARTESIAN_POINT ( 'NONE',  ( -3.756430356249997882, 27.65312499938548640, 11.16877607737301226 ) ) ;
#8825=CARTESIAN_POINT ( 'NONE',  ( -2.000000000000003997, -25.07499999999999929, 5.535898384862238508 ) ) ;
#8826=EDGE_CURVE ( 'NONE', #19703, #3427, #22438, .T. ) ;
#8829=CARTESIAN_POINT ( 'NONE',  ( 3.756430356249996105, -28.02812499938548996, 6.831223922626973533 ) ) ;
#8842=CARTESIAN_POINT ( 'NONE',  ( 3.756430356249996105, -27.24062499938548498, 6.831223922626973533 ) ) ;
#8845=AXIS2_PLACEMENT_3D ( 'NONE', #6576, #8672, #22680 ) ;
#8849=AXIS2_PLACEMENT_3D ( 'NONE', #9164, #13224, #8783 ) ;
#8857=CARTESIAN_POINT ( 'NONE',  ( 16.55955693104344206, 22.21641118053575426, 8.999999999999992895 ) ) ;
#8858=CARTESIAN_POINT ( 'NONE',  ( 5.577813053751546416E-15, 25.33750000000000213, 12.99999999999999289 ) ) ;
#8859=CARTESIAN_POINT ( 'NONE',  ( 17.91631806831418317, 17.91631806831411922, 13.61880215351699874 ) ) ;
#8860=CARTESIAN_POINT ( 'NONE',  ( 19.44991966514168169, 16.79372228718224491, 12.25316411605952283 ) ) ;
#8869=CARTESIAN_POINT ( 'NONE',  ( 22.72022476213122744, 17.06337051263877669, 6.690598923241489970 ) ) ;
#8872=CARTESIAN_POINT ( 'NONE',  ( 3.752267015613588906E-15, 29.10624999877096997, 4.381197846482986158 ) ) ;
#8873=CARTESIAN_POINT ( 'NONE',  ( -1.878215178125004048, -27.91562499938548569, 5.746835883940462963 ) ) ;
#8875=ORIENTED_EDGE ( 'NONE', *, *, #5808, .F. ) ;
#8879=CARTESIAN_POINT ( 'NONE',  ( 1.878215178124995832, -26.19062499938548427, 5.746835883940462963 ) ) ;
#8883=CIRCLE ( 'NONE', #14720, 4.000000000000000000 ) ;
#8889=DIRECTION ( 'NONE',  ( 0.000000000000000000, 0.000000000000000000, -1.000000000000000000 ) ) ;
#8890=CARTESIAN_POINT ( 'NONE',  ( 3.735045420075836212E-15, 27.50312499938548783, 4.662447845253954171 ) ) ;
#8892=CARTESIAN_POINT ( 'NONE',  ( 21.23398739633539023, 19.71823786848327131, 12.99999999999999467 ) ) ;
#8901=CARTESIAN_POINT ( 'NONE',  ( -3.756430356250003655, -27.05312499938548498, 8.999999999999992895 ) ) ;
#8909=DIRECTION ( 'NONE',  ( 0.000000000000000000, 1.000000000000000000, 0.000000000000000000 ) ) ;
#8911=EDGE_LOOP ( 'NONE', ( #22109, #646, #15839, #17067 ) ) ;
#8912=EDGE_CURVE ( 'NONE', #421, #22340, #25121, .T. ) ;
#8914=ORIENTED_EDGE ( 'NONE', *, *, #11059, .T. ) ;
#8921=CARTESIAN_POINT ( 'NONE',  ( -1.878215178124998497, 29.60312499938548569, 12.25316411605951927 ) ) ;
#8925=CARTESIAN_POINT ( 'NONE',  ( -4.000000000000003553, -25.39374999877096784, 8.999999999999992895 ) ) ;
#8926=CARTESIAN_POINT ( 'NONE',  ( -3.756430356249995661, 26.79062499938548925, 6.831223922626973533 ) ) ;
#8931=DIRECTION ( 'NONE',  ( 0.000000000000000000, -1.000000000000000000, 0.000000000000000000 ) ) ;
#8936=DIRECTION ( 'NONE',  ( 0.000000000000000000, 0.000000000000000000, -1.000000000000000000 ) ) ;
#8938=CARTESIAN_POINT ( 'NONE',  ( 3.999999999999995559, -26.53750000000000142, 6.690598923241487306 ) ) ;
#8942=( BOUNDED_CURVE ( )  B_SPLINE_CURVE ( 2, ( #1948, #16076, #3911, #14376, #18170, #17895, #19969, #2074, #16468 ),
 .UNSPECIFIED., .F., .F. ) 
 B_SPLINE_CURVE_WITH_KNOTS ( ( 3, 2, 2, 2, 3 ),
 ( 0.3750000000000000000, 0.3833333333333333592, 0.4000000000000000222, 0.4166666666666666852, 0.4250000000000000444 ),
 .UNSPECIFIED. ) 
 CURVE ( )  GEOMETRIC_REPRESENTATION_ITEM ( )  RATIONAL_B_SPLINE_CURVE ( ( 0.9330127018922194093, 0.9330127018922194093, 1.000000000000000000, 0.8660254037844387076, 1.000000000000000000, 0.8660254037844387076, 1.000000000000000000, 0.9330127018922191873, 0.9330127018922194093 ) ) 
 REPRESENTATION_ITEM ( '' )  );
#8943=VERTEX_POINT ( 'NONE', #11751 ) ;
#8947=CARTESIAN_POINT ( 'NONE',  ( -3.756430356250002323, -26.11562499938548498, 11.16877607737301226 ) ) ;
#8952=CARTESIAN_POINT ( 'NONE',  ( 1.057460391440397258E-14, -29.16249999999999787, 4.999999999999992006 ) ) ;
#8954=CARTESIAN_POINT ( 'NONE',  ( 19.18911027444997686, 19.18911027444989870, 12.99999999999999112 ) ) ;
#8957=CARTESIAN_POINT ( 'NONE',  ( 20.19238178538755690, 17.53618440742811302, 5.746835883940462963 ) ) ;
#8959=CARTESIAN_POINT ( 'NONE',  ( -3.999999999999996447, 26.12500000000000355, 8.999999999999992895 ) ) ;
#8960=CARTESIAN_POINT ( 'NONE',  ( 16.31415173562648491, 21.62654649154516306, 8.999999999999992895 ) ) ;
#8962=ORIENTED_EDGE ( 'NONE', *, *, #8461, .T. ) ;
#8964=CARTESIAN_POINT ( 'NONE',  ( 1.878215178124995832, -27.09062499938548640, 5.746835883940462963 ) ) ;
#8970=ORIENTED_EDGE ( 'NONE', *, *, #25631, .F. ) ;
#8975=EDGE_LOOP ( 'NONE', ( #8546, #2393 ) ) ;
#8976=CARTESIAN_POINT ( 'NONE',  ( -1.071796769724488563, 25.76740381056766793, 12.99999999999999289 ) ) ;
#8977=EDGE_CURVE ( 'NONE', #8256, #20149, #7822, .T. ) ;
#8983=CARTESIAN_POINT ( 'NONE',  ( 1.071796769724487230, -28.28259618943233988, 4.999999999999992006 ) ) ;
#8985=CARTESIAN_POINT ( 'NONE',  ( 1.878215178125004048, 27.91562499938548569, 5.746835883940462963 ) ) ;
#8987=CARTESIAN_POINT ( 'NONE',  ( 20.82429470594385634, 15.16744045645140915, 8.999999999999992895 ) ) ;
#8988=CARTESIAN_POINT ( 'NONE',  ( 15.70427213685309020, 21.01666689277176658, 11.16877607737301226 ) ) ;
#8992=CARTESIAN_POINT ( 'NONE',  ( 17.21571288163933033, 22.52810763755800494, 11.16877607737301048 ) ) ;
#8993=ORIENTED_EDGE ( 'NONE', *, *, #3561, .F. ) ;
#8995=CARTESIAN_POINT ( 'NONE',  ( -1.999999999999995781, 28.24374999877096570, 5.535898384862237620 ) ) ;
#8996=CARTESIAN_POINT ( 'NONE',  ( -3.756430356250003655, -27.84062499938548640, 8.999999999999992895 ) ) ;
#9001=EDGE_LOOP ( 'NONE', ( #2065, #11333, #20394, #11800 ) ) ;
#9002=CARTESIAN_POINT ( 'NONE',  ( 1.878215178124995832, -27.54062499938548214, 5.746835883940462963 ) ) ;
#9006=CARTESIAN_POINT ( 'NONE',  ( 19.41874785118199043, 22.86831248503511205, 5.819033386899013394 ) ) ;
#9011=CARTESIAN_POINT ( 'NONE',  ( 3.756430356250002323, 28.25312499938548427, 11.16877607737301226 ) ) ;
#9014=FACE_OUTER_BOUND ( 'NONE', #12797, .T. ) ;
#9018=CARTESIAN_POINT ( 'NONE',  ( 1.878215178124995832, -28.10312499938548569, 5.746835883940462963 ) ) ;
#9031=DIRECTION ( 'NONE',  ( 0.000000000000000000, 0.000000000000000000, -1.000000000000000000 ) ) ;
#9033=( BOUNDED_CURVE ( )  B_SPLINE_CURVE ( 2, ( #3744, #10143, #17618, #1925, #15536, #1801, #4005, #23503, #22042 ),
 .UNSPECIFIED., .F., .F. ) 
 B_SPLINE_CURVE_WITH_KNOTS ( ( 3, 2, 2, 2, 3 ),
 ( 0.1749999999999999889, 0.1833333333333333204, 0.2000000000000000111, 0.2166666666666666741, 0.2250000000000000056 ),
 .UNSPECIFIED. ) 
 CURVE ( )  GEOMETRIC_REPRESENTATION_ITEM ( )  RATIONAL_B_SPLINE_CURVE ( ( 0.9330127018922194093, 0.9330127018922194093, 1.000000000000000000, 0.8660254037844387076, 1.000000000000000000, 0.8660254037844387076, 1.000000000000000000, 0.9330127018922194093, 0.9330127018922194093 ) ) 
 REPRESENTATION_ITEM ( '' )  );
#9035=EDGE_CURVE ( 'NONE', #1175, #24947, #12267, .T. ) ;
#9036=CARTESIAN_POINT ( 'NONE',  ( -3.756430356249996994, 29.07812499938548356, 8.999999999999992895 ) ) ;
#9037=EDGE_CURVE ( 'NONE', #13915, #130, #24158, .T. ) ;
#9040=CARTESIAN_POINT ( 'NONE',  ( 23.58876780933789519, 18.27637305341907492, 11.16877607737301226 ) ) ;
#9042=CARTESIAN_POINT ( 'NONE',  ( -1.878215178124998497, 26.90312499938548285, 12.25316411605951927 ) ) ;
#9043=CARTESIAN_POINT ( 'NONE',  ( 15.85973458909327505, -20.67279826512041296, 20.00001199999999457 ) ) ;
#9047=CARTESIAN_POINT ( 'NONE',  ( -3.834746474454188013E-15, -28.20624999877096428, 4.999999999999992006 ) ) ;
#9055=CARTESIAN_POINT ( 'NONE',  ( 0.000000000000000000, 10.00000000000000000, 15.00000000000000178 ) ) ;
#9057=CARTESIAN_POINT ( 'NONE',  ( -3.735045420075836212E-15, -25.81562499938548783, 4.662447845253954171 ) ) ;
#9064=CARTESIAN_POINT ( 'NONE',  ( 18.28634663658058912, 19.80209616443256593, 4.999999999999992895 ) ) ;
#9067=DIRECTION ( 'NONE',  ( 0.7071067811865487940, 0.7071067811865463515, 0.000000000000000000 ) ) ;
#9068=CARTESIAN_POINT ( 'NONE',  ( 21.12273290994980712, 15.81033815403099752, 11.16877607737301226 ) ) ;
#9070=CARTESIAN_POINT ( 'NONE',  ( -1.999999999999995781, 25.60000000000000142, 5.535898384862237620 ) ) ;
#9071=( BOUNDED_CURVE ( )  B_SPLINE_CURVE ( 2, ( #954, #1337, #1462, #1192, #23171, #5251, #6956, #14936, #11252 ),
 .UNSPECIFIED., .F., .F. ) 
 B_SPLINE_CURVE_WITH_KNOTS ( ( 3, 2, 2, 2, 3 ),
 ( 0.7249999999999999778, 0.7333333333333332815, 0.7500000000000000000, 0.7666666666666667185, 0.7750000000000000222 ),
 .UNSPECIFIED. ) 
 CURVE ( )  GEOMETRIC_REPRESENTATION_ITEM ( )  RATIONAL_B_SPLINE_CURVE ( ( 0.9330127018922194093, 0.9330127018922194093, 1.000000000000000000, 0.8660254037844387076, 1.000000000000000000, 0.8660254037844387076, 1.000000000000000000, 0.9330127018922194093, 0.9330127018922194093 ) ) 
 REPRESENTATION_ITEM ( '' )  );
#9072=EDGE_CURVE ( 'NONE', #18519, #20151, #22982, .T. ) ;
#9073=CARTESIAN_POINT ( 'NONE',  ( 17.26874589022832751, 22.58114064614699856, 8.999999999999992895 ) ) ;
#9075=ORIENTED_EDGE ( 'NONE', *, *, #12648, .T. ) ;
#9077=CARTESIAN_POINT ( 'NONE',  ( -3.756430356250003655, -27.84062499938548640, 8.999999999999992895 ) ) ;
#9080=CARTESIAN_POINT ( 'NONE',  ( -3.469446951953614189E-15, -30.00000000000000355, 4.999999999999992006 ) ) ;
#9086=ORIENTED_EDGE ( 'NONE', *, *, #8699, .F. ) ;
#9087=CARTESIAN_POINT ( 'NONE',  ( 3.756430356249997438, -29.56562499938549493, 11.16877607737301048 ) ) ;
#9090=CARTESIAN_POINT ( 'NONE',  ( -2.000000000000003997, -26.36874999877096926, 5.535898384862238508 ) ) ;
#9092=EDGE_CURVE ( 'NONE', #20170, #25112, #24275, .T. ) ;
#9095=CARTESIAN_POINT ( 'NONE',  ( -3.999999999999995559, 26.98750000000000071, 6.690598923241487306 ) ) ;
#9098=CARTESIAN_POINT ( 'NONE',  ( -1.878215178124998497, 26.79062499938548214, 12.25316411605951927 ) ) ;
#9100=CARTESIAN_POINT ( 'NONE',  ( 18.07541709408115693, 18.07541709408108943, 4.381197846482986158 ) ) ;
#9101=CARTESIAN_POINT ( 'NONE',  ( 18.09530447186750024, 18.09530447186743629, 13.33755215474602984 ) ) ;
#9103=CARTESIAN_POINT ( 'NONE',  ( 23.83637464252882765, 18.21619809234428189, 8.475804415688520166 ) ) ;
#9104=CARTESIAN_POINT ( 'NONE',  ( 17.93393197184562027, 20.59012934980492560, 12.25316411605951927 ) ) ;
#9105=CARTESIAN_POINT ( 'NONE',  ( 23.62178590814407642, 17.96493165865162212, 11.30940107675849760 ) ) ;
#9107=VERTEX_POINT ( 'NONE', #2714 ) ;
#9109=CARTESIAN_POINT ( 'NONE',  ( 3.752267015613588906E-15, 28.65624999877096712, 4.381197846482986158 ) ) ;
#9110=CARTESIAN_POINT ( 'NONE',  ( -4.000000000000001776, -25.41250000000000142, 11.30940107675849760 ) ) ;
#9115=CARTESIAN_POINT ( 'NONE',  ( 1.878215178124995832, -28.44062499938548427, 5.746835883940462963 ) ) ;
#9116=ORIENTED_EDGE ( 'NONE', *, *, #23564, .F. ) ;
#9118=CARTESIAN_POINT ( 'NONE',  ( 18.19529158423879878, 23.85228215861205570, 9.259737768674039415 ) ) ;
#9124=EDGE_CURVE ( 'NONE', #961, #19280, #4558, .T. ) ;
#9125=AXIS2_PLACEMENT_3D ( 'NONE', #7606, #5379, #6862 ) ;
#9127=DIRECTION ( 'NONE',  ( 0.000000000000000000, 0.000000000000000000, -1.000000000000000000 ) ) ;
#9130=DIRECTION ( 'NONE',  ( 0.000000000000000000, -1.000000000000000000, 0.000000000000000000 ) ) ;
#9133=DIRECTION ( 'NONE',  ( 0.000000000000000000, -1.000000000000000000, 0.000000000000000000 ) ) ;
#9140=DIRECTION ( 'NONE',  ( 0.000000000000000000, 0.000000000000000000, -1.000000000000000000 ) ) ;
#9143=CARTESIAN_POINT ( 'NONE',  ( -3.959305739469038251E-15, -30.00000000000000355, 12.99999999999999289 ) ) ;
#9150=( BOUNDED_CURVE ( )  B_SPLINE_CURVE ( 2, ( #11120, #12833, #20807, #2890, #19099 ),
 .UNSPECIFIED., .F., .F. ) 
 B_SPLINE_CURVE_WITH_KNOTS ( ( 3, 2, 3 ),
 ( 0.9749999999999999778, 0.9833333333333332815, 1.000000000000000000 ),
 .UNSPECIFIED. ) 
 CURVE ( )  GEOMETRIC_REPRESENTATION_ITEM ( )  RATIONAL_B_SPLINE_CURVE ( ( 0.9330127018922194093, 0.9330127018922194093, 1.000000000000000000, 0.8660254037844387076, 1.000000000000000000 ) ) 
 REPRESENTATION_ITEM ( '' )  );
#9151=AXIS2_PLACEMENT_3D ( 'NONE', #19146, #25181, #23331 ) ;
#9154=VERTEX_POINT ( 'NONE', #885 ) ;
#9156=ORIENTED_EDGE ( 'NONE', *, *, #6865, .T. ) ;
#9160=AXIS2_PLACEMENT_3D ( 'NONE', #22214, #2217, #10174 ) ;
#9163=CARTESIAN_POINT ( 'NONE',  ( 19.41885621233737069, 22.07505359029666536, 5.746835883940462963 ) ) ;
#9164=CARTESIAN_POINT ( 'NONE',  ( -3.469446951953614189E-15, -30.00000000000000355, 8.999999999999992895 ) ) ;
#9167=CARTESIAN_POINT ( 'NONE',  ( 18.15054718871317974, 23.80740143820548482, 8.999999999999992895 ) ) ;
#9171=DIRECTION ( 'NONE',  ( 1.000000000000000000, 0.000000000000000000, 0.000000000000000000 ) ) ;
#9172=CARTESIAN_POINT ( 'NONE',  ( -4.000000000000003553, -29.50000000000000355, 8.999999999999992895 ) ) ;
#9173=EDGE_CURVE ( 'NONE', #8491, #17932, #10743, .T. ) ;
#9174=CARTESIAN_POINT ( 'NONE',  ( 1.999999999999995781, -25.54374999877096997, 5.535898384862237620 ) ) ;
#9176=CARTESIAN_POINT ( 'NONE',  ( 3.999999999999997335, -26.61250000000000071, 11.30940107675849404 ) ) ;
#9177=CARTESIAN_POINT ( 'NONE',  ( 3.469446951953614189E-15, 25.00000000000000000, 8.999999999999992895 ) ) ;
#9179=ADVANCED_FACE ( 'NONE', ( #22732 ), #22984, .F. ) ;
#9183=EDGE_CURVE ( 'NONE', #21627, #24890, #18384, .T. ) ;
#9187=ORIENTED_EDGE ( 'NONE', *, *, #15864, .F. ) ;
#9188=CARTESIAN_POINT ( 'NONE',  ( 3.756430356249995661, -26.79062499938548925, 6.831223922626973533 ) ) ;
#9193=ORIENTED_EDGE ( 'NONE', *, *, #22721, .F. ) ;
#9194=CARTESIAN_POINT ( 'NONE',  ( 21.21320343559646915, 21.21320343559638744, 12.99999999999999289 ) ) ;
#9200=CARTESIAN_POINT ( 'NONE',  ( 20.82877788845545552, 18.17258051049600454, 5.746835883940462963 ) ) ;
#9203=AXIS2_PLACEMENT_3D ( 'NONE', #25709, #20842, #25403 ) ;
#9204=CARTESIAN_POINT ( 'NONE',  ( 2.620986760973688460E-15, 25.33750000000000568, 13.61880215351699874 ) ) ;
#9206=CARTESIAN_POINT ( 'NONE',  ( 22.07732706455164617, 16.76493230863282591, 11.16877607737301403 ) ) ;
#9212=CARTESIAN_POINT ( 'NONE',  ( 3.756430356249996994, -29.41562499938548569, 8.999999999999992895 ) ) ;
#9221=AXIS2_PLACEMENT_3D ( 'NONE', #13700, #7562, #25231 ) ;
#9226=CARTESIAN_POINT ( 'NONE',  ( -3.756430356250003655, -28.85312499938548569, 8.999999999999992895 ) ) ;
#9230=CARTESIAN_POINT ( 'NONE',  ( 20.41007196385330147, 18.89432243600117900, 4.999999999999992895 ) ) ;
#9232=( BOUNDED_CURVE ( )  B_SPLINE_CURVE ( 2, ( #10253, #328, #16040, #18136, #20196 ),
 .UNSPECIFIED., .F., .F. ) 
 B_SPLINE_CURVE_WITH_KNOTS ( ( 3, 2, 3 ),
 ( 0.000000000000000000, 0.01666666666666666644, 0.02500000000000000486 ),
 .UNSPECIFIED. ) 
 CURVE ( )  GEOMETRIC_REPRESENTATION_ITEM ( )  RATIONAL_B_SPLINE_CURVE ( ( 1.000000000000000000, 0.8660254037844387076, 1.000000000000000000, 0.9330127018922194093, 0.9330127018922194093 ) ) 
 REPRESENTATION_ITEM ( '' )  );
#9240=CARTESIAN_POINT ( 'NONE',  ( 1.878215178125000939, 27.76562499938548356, 12.25316411605952283 ) ) ;
#9241=CARTESIAN_POINT ( 'NONE',  ( -1.775433037296146654, -29.94838521766437722, 5.406171146379000092 ) ) ;
#9242=CARTESIAN_POINT ( 'NONE',  ( 14.98182492639001673, 20.63867917588233070, 6.690598923241487306 ) ) ;
#9243=CARTESIAN_POINT ( 'NONE',  ( 21.14924941424430571, 15.83685465832548900, 8.999999999999992895 ) ) ;
#9244=EDGE_CURVE ( 'NONE', #12726, #1614, #20758, .T. ) ;
#9245=CYLINDRICAL_SURFACE ( 'NONE', #12575, 4.000000000000000000 ) ;
#9247=VECTOR ( 'NONE', #12646, 1000.000000000000000 ) ;
#9249=CARTESIAN_POINT ( 'NONE',  ( 16.52628376998245230, 21.83867852590111980, 6.831223922626973533 ) ) ;
#9253=CARTESIAN_POINT ( 'NONE',  ( -1.878215178124995832, 26.30312499938548498, 5.746835883940462963 ) ) ;
#9254=CARTESIAN_POINT ( 'NONE',  ( 3.999999999999997335, -25.26249999999999929, 11.30940107675849404 ) ) ;
#9256=ORIENTED_EDGE ( 'NONE', *, *, #19094, .F. ) ;
#9260=CARTESIAN_POINT ( 'NONE',  ( -2.672651547586948120E-15, -29.07812499938548001, 13.33755215474602984 ) ) ;
#9262=ORIENTED_EDGE ( 'NONE', *, *, #18674, .F. ) ;
#9278=PLANE ( 'NONE',  #14314 ) ;
#9279=CARTESIAN_POINT ( 'NONE',  ( -1.071796769724492338, -29.80134618820330417, 12.99999999999999467 ) ) ;
#9280=CARTESIAN_POINT ( 'NONE',  ( -3.756430356250003655, -29.30312499938548498, 8.999999999999992895 ) ) ;
#9282=CARTESIAN_POINT ( 'NONE',  ( 20.10392967174102097, 20.10392967174092860, 12.99999999999999289 ) ) ;
#9286=CARTESIAN_POINT ( 'NONE',  ( 1.039771317798496408, -29.98307469845295969, 12.87134967428165666 ) ) ;
#9293=VERTEX_POINT ( 'NONE', #1132 ) ;
#9295=EDGE_LOOP ( 'NONE', ( #1976, #13211, #15688, #23274, #10527, #14946, #25082, #12452, #14548, #5114, #10489, #8025, #13237, #19401, #23306, #5037, #4539, #13381, #9187, #1623, #3706, #3499, #12398, #763 ) ) ;
#9298=DIRECTION ( 'NONE',  ( 0.000000000000000000, 1.000000000000000000, 0.000000000000000000 ) ) ;
#9299=EDGE_CURVE ( 'NONE', #10227, #14283, #7248, .T. ) ;
#9302=AXIS2_PLACEMENT_3D ( 'NONE', #11400, #4999, #12981 ) ;
#9305=CARTESIAN_POINT ( 'NONE',  ( -3.756430356249996994, 25.47812499938548569, 8.999999999999992895 ) ) ;
#9306=CARTESIAN_POINT ( 'NONE',  ( -2.000000000000003997, -26.81874999877096855, 5.535898384862238508 ) ) ;
#9307=CARTESIAN_POINT ( 'NONE',  ( 19.51172774249728192, 22.34015486724339183, 5.535898384862237620 ) ) ;
#9309=FACE_OUTER_BOUND ( 'NONE', #5198, .T. ) ;
#9312=CARTESIAN_POINT ( 'NONE',  ( 1.999999999999995781, -26.44374999877096855, 5.535898384862237620 ) ) ;
#9326=CARTESIAN_POINT ( 'NONE',  ( -3.735045420075836212E-15, -28.96562499938548640, 4.662447845253954171 ) ) ;
#9329=EDGE_CURVE ( 'NONE', #1173, #5294, #9905, .T. ) ;
#9330=AXIS2_PLACEMENT_3D ( 'NONE', #11273, #19257, #1357 ) ;
#9337=CARTESIAN_POINT ( 'NONE',  ( 16.66113976570983368, 19.31733714366914256, 12.25316411605951927 ) ) ;
#9338=EDGE_CURVE ( 'NONE', #23470, #10871, #21727, .T. ) ;
#9340=CARTESIAN_POINT ( 'NONE',  ( -3.999999999999997335, 25.26249999999999929, 11.30940107675849404 ) ) ;
#9341=CARTESIAN_POINT ( 'NONE',  ( 21.75912901301770219, 16.44673425709888548, 11.16877607737301403 ) ) ;
#9342=DIRECTION ( 'NONE',  ( 0.000000000000000000, 1.000000000000000000, 0.000000000000000000 ) ) ;
#9348=CARTESIAN_POINT ( 'NONE',  ( -1.878215178125004048, -29.26562499938548356, 5.746835883940462963 ) ) ;
#9353=CARTESIAN_POINT ( 'NONE',  ( 3.063240906311874401, 29.84319947910909931, 11.57226653943513028 ) ) ;
#9354=ORIENTED_EDGE ( 'NONE', *, *, #19887, .F. ) ;
#9356=CARTESIAN_POINT ( 'NONE',  ( 3.469446951953614189E-15, 30.00000000000000355, 8.999999999999992895 ) ) ;
#9358=EDGE_LOOP ( 'NONE', ( #377, #15720 ) ) ;
#9359=CARTESIAN_POINT ( 'NONE',  ( -3.756430356250003655, -29.75312499938548783, 8.999999999999992895 ) ) ;
#9360=DIRECTION ( 'NONE',  ( 0.000000000000000000, -1.000000000000000000, 0.000000000000000000 ) ) ;
#9364=EDGE_CURVE ( 'NONE', #23065, #20357, #15527, .T. ) ;
#9366=CARTESIAN_POINT ( 'NONE',  ( -30.00000000000000355, 0.000000000000000000, 20.00000000000000000 ) ) ;
#9369=ADVANCED_FACE ( 'NONE', ( #25834 ), #17359, .F. ) ;
#9370=CARTESIAN_POINT ( 'NONE',  ( -3.756430356249996994, 27.16562499938548214, 8.999999999999992895 ) ) ;
#9372=CARTESIAN_POINT ( 'NONE',  ( 19.10065816080342671, 21.75685553876272493, 5.746835883940462963 ) ) ;
#9373=CARTESIAN_POINT ( 'NONE',  ( 17.87862548900172044, 23.19102024492039504, 6.831223922626973533 ) ) ;
#9374=CARTESIAN_POINT ( 'NONE',  ( 18.99023649137219039, 18.99023649137212999, 4.999999999999991118 ) ) ;
#9375=CARTESIAN_POINT ( 'NONE',  ( 0.000000000000000000, 0.000000000000000000, 20.00000000000000000 ) ) ;
#9379=CARTESIAN_POINT ( 'NONE',  ( 18.88852612644745932, 21.54472350440676109, 12.25316411605951927 ) ) ;
#9380=DIRECTION ( 'NONE',  ( 0.7071067811865487940, 0.7071067811865463515, 0.000000000000000000 ) ) ;
#9381=ORIENTED_EDGE ( 'NONE', *, *, #5808, .T. ) ;
#9383=CARTESIAN_POINT ( 'NONE',  ( 3.756430356250003655, 25.70312499938548356, 8.999999999999992895 ) ) ;
#9384=CARTESIAN_POINT ( 'NONE',  ( 1.878215178124998497, -28.59062499938548285, 12.25316411605951927 ) ) ;
#9387=CARTESIAN_POINT ( 'NONE',  ( -20.67279826512042717, 15.85973458909326084, 20.00001200000000168 ) ) ;
#9388=CARTESIAN_POINT ( 'NONE',  ( -3.756430356250004099, -27.42812499938548143, 6.831223922626973533 ) ) ;
#9391=CARTESIAN_POINT ( 'NONE',  ( 18.21624468915290507, 23.83633969896351701, 9.525109153848150711 ) ) ;
#9395=CARTESIAN_POINT ( 'NONE',  ( 3.999999999999997335, -27.45624999877096784, 11.30940107675849404 ) ) ;
#9397=FACE_OUTER_BOUND ( 'NONE', #5647, .T. ) ;
#9398=CARTESIAN_POINT ( 'NONE',  ( -2.665892461326258456, -29.88220662469441891, 11.99618178085344056 ) ) ;
#9401=CARTESIAN_POINT ( 'NONE',  ( 18.83113746560522372, 18.83113746560515622, 13.61880215351699874 ) ) ;
#9402=B_SPLINE_CURVE_WITH_KNOTS ( 'NONE', 3,
 ( #2210, #10168, #12386, #22453, #245, #16462, #18166, #12514, #22330, #20353, #122, #18035, #8214, #2328, #16188, #4412, #18409, #11991, #20232, #10288, #6245, #14236, #20491, #22205, #19965, #6381, #18280, #368, #16072, #13977, #2587, #2448, #10551, #24034 ),
 .UNSPECIFIED., .F., .F.,
 ( 4, 2, 2, 2, 2, 2, 2, 2, 2, 2, 2, 2, 2, 2, 2, 2, 4 ),
 ( 0.000000000000000000, 0.0007824850735655043557, 0.001564970147131008711, 0.002347455220696513176, 0.003129940294262017423, 0.003912425367827521670, 0.004694910441393026351, 0.005477395514958530165, 0.006259880588524034846, 0.007042365662089539527, 0.007824850735655043341, 0.008607335809220547154, 0.009389820882786052703, 0.01017230595635155652, 0.01095479102991706033, 0.01173727610348256588, 0.01251976117704806969 ),
 .UNSPECIFIED. ) ;
#9404=CARTESIAN_POINT ( 'NONE',  ( 0.000000000000000000, 0.000000000000000000, 20.00000000000000000 ) ) ;
#9408=ADVANCED_FACE ( 'NONE', ( #9759 ), #9492, .T. ) ;
#9410=CARTESIAN_POINT ( 'NONE',  ( 0.5265545572341292502, -29.99647701088549923, 12.97381592328244082 ) ) ;
#9412=CARTESIAN_POINT ( 'NONE',  ( 1.999999999999998224, -27.04374999877096641, 12.46410161513774639 ) ) ;
#9426=PRESENTATION_STYLE_ASSIGNMENT (( #3270 ) ) ;
#9427=CARTESIAN_POINT ( 'NONE',  ( 2.672651547586948120E-15, 29.19062499938548783, 13.33755215474602984 ) ) ;
#9429=CARTESIAN_POINT ( 'NONE',  ( 3.834746474454188013E-15, 28.65624999877096712, 4.999999999999992006 ) ) ;
#9432=CARTESIAN_POINT ( 'NONE',  ( 3.469446951953614189E-15, 30.00000000000000355, 8.999999999999992895 ) ) ;
#9434=CARTESIAN_POINT ( 'NONE',  ( -4.000000000000001776, -29.46250000000000213, 11.30940107675849760 ) ) ;
#9435=CARTESIAN_POINT ( 'NONE',  ( 1.999999999999998224, -27.04374999877096641, 12.46410161513774639 ) ) ;
#9439=CARTESIAN_POINT ( 'NONE',  ( -4.000000000000001776, -25.86250000000000071, 11.30940107675849760 ) ) ;
#9441=DIRECTION ( 'NONE',  ( 0.000000000000000000, 0.000000000000000000, 1.000000000000000000 ) ) ;
#9445=CYLINDRICAL_SURFACE ( 'NONE', #14977, 24.00000000000000355 ) ;
#9447=CARTESIAN_POINT ( 'NONE',  ( -3.756430356250002323, -28.36562499938548854, 11.16877607737301226 ) ) ;
#9450=EDGE_LOOP ( 'NONE', ( #11879, #24235, #9830, #1952 ) ) ;
#9454=CARTESIAN_POINT ( 'NONE',  ( 0.000000000000000000, 0.000000000000000000, 15.00000000000000178 ) ) ;
#9455=CARTESIAN_POINT ( 'NONE',  ( 22.76675617620853131, 17.45436142028971460, 6.831223922626973533 ) ) ;
#9457=CARTESIAN_POINT ( 'NONE',  ( -3.756430356250003655, -25.25312499938548427, 8.999999999999992895 ) ) ;
#9459=CARTESIAN_POINT ( 'NONE',  ( 3.752267015613588906E-15, 26.91250000000000142, 4.381197846482986158 ) ) ;
#9461=CARTESIAN_POINT ( 'NONE',  ( 17.69528343319515784, 20.35148081115446317, 12.25316411605951927 ) ) ;
#9462=CARTESIAN_POINT ( 'NONE',  ( 2.000000000000003997, 26.81874999877096855, 5.535898384862238508 ) ) ;
#9467=CYLINDRICAL_SURFACE ( 'NONE', #21665, 4.000000000000000000 ) ;
#9472=ORIENTED_EDGE ( 'NONE', *, *, #12593, .T. ) ;
#9476=CARTESIAN_POINT ( 'NONE',  ( 3.756430356249996105, -28.14062499938548356, 6.831223922626973533 ) ) ;
#9481=CARTESIAN_POINT ( 'NONE',  ( 3.756430356250002323, 27.35312499938547859, 11.16877607737301226 ) ) ;
#9484=CARTESIAN_POINT ( 'NONE',  ( -1.878215178124995832, 25.74062499938548498, 5.746835883940462963 ) ) ;
#9486=CARTESIAN_POINT ( 'NONE',  ( 21.43417430471724927, 15.77732005522480563, 11.30940107675849760 ) ) ;
#9487=CARTESIAN_POINT ( 'NONE',  ( 22.39552511608559371, 17.08313036016677700, 11.16877607737301226 ) ) ;
#9489=CARTESIAN_POINT ( 'NONE',  ( 0.000000000000000000, 10.00000000000000000, 15.00000000000000178 ) ) ;
#9491=CARTESIAN_POINT ( 'NONE',  ( 22.02429405596265610, 16.71189930004383584, 8.999999999999992895 ) ) ;
#9492=PLANE ( 'NONE',  #9203 ) ;
#9493=VERTEX_POINT ( 'NONE', #9457 ) ;
#9495=CARTESIAN_POINT ( 'NONE',  ( 3.999999999999996003, -25.63749999999999929, 6.690598923241487306 ) ) ;
#9501=CARTESIAN_POINT ( 'NONE',  ( 1.071796769724488563, -29.76115380933863364, 12.99999999999999289 ) ) ;
#9502=CARTESIAN_POINT ( 'NONE',  ( -1.701696020694479783, 25.99999999999999645, 20.00001200000000523 ) ) ;
#9503=CARTESIAN_POINT ( 'NONE',  ( 1.878215178124998497, -27.24062499938548498, 12.25316411605951927 ) ) ;
#9518=CARTESIAN_POINT ( 'NONE',  ( 17.07220934740368889, 19.90063647214981302, 12.46410161513774639 ) ) ;
#9521=CARTESIAN_POINT ( 'NONE',  ( -3.756430356250002323, -28.81562499938548427, 11.16877607737301226 ) ) ;
#9526=CARTESIAN_POINT ( 'NONE',  ( -1.057460391440397258E-14, 29.10624999877096641, 4.999999999999992006 ) ) ;
#9527=VERTEX_POINT ( 'NONE', #23074 ) ;
#9529=CARTESIAN_POINT ( 'NONE',  ( 3.756430356249995661, -25.32812499938548356, 6.831223922626973533 ) ) ;
#9531=ORIENTED_EDGE ( 'NONE', *, *, #14503, .F. ) ;
#9536=EDGE_LOOP ( 'NONE', ( #16438, #23920, #14697, #9531 ) ) ;
#9545=CARTESIAN_POINT ( 'NONE',  ( -1.878215178124998497, 27.80312499938548498, 12.25316411605951927 ) ) ;
#9548=CARTESIAN_POINT ( 'NONE',  ( 20.89942480057588980, 20.89942480057579033, 4.999999999999992006 ) ) ;
#9552=CARTESIAN_POINT ( 'NONE',  ( 4.000000000000003553, 25.19687499938548569, 8.999999999999992895 ) ) ;
#9553=CARTESIAN_POINT ( 'NONE',  ( 1.999999999999995781, -25.99374999877096926, 5.535898384862237620 ) ) ;
#9554=CARTESIAN_POINT ( 'NONE',  ( 1.878215178125004048, 27.12812499938548783, 5.746835883940462963 ) ) ;
#9555=AXIS2_PLACEMENT_3D ( 'NONE', #11949, #2404, #10508 ) ;
#9560=ORIENTED_EDGE ( 'NONE', *, *, #17459, .T. ) ;
#9567=CARTESIAN_POINT ( 'NONE',  ( 3.756430356249995661, -29.04062499938548569, 6.831223922626973533 ) ) ;
#9570=EDGE_CURVE ( 'NONE', #5581, #14528, #20053, .T. ) ;
#9575=VECTOR ( 'NONE', #3566, 1000.000000000000000 ) ;
#9576=EDGE_CURVE ( 'NONE', #1614, #10560, #20935, .T. ) ;
#9580=CARTESIAN_POINT ( 'NONE',  ( 23.37663577498192780, 18.06424101906310753, 8.999999999999992895 ) ) ;
#9583=CARTESIAN_POINT ( 'NONE',  ( 2.620986760973688460E-15, 27.13750000000000284, 13.61880215351699874 ) ) ;
#9585=CARTESIAN_POINT ( 'NONE',  ( 18.86200962215296784, 21.51820700011226606, 5.746835883940462963 ) ) ;
#9586=CARTESIAN_POINT ( 'NONE',  ( -2.000000000000003997, -29.51874999877096784, 5.535898384862238508 ) ) ;
#9595=CARTESIAN_POINT ( 'NONE',  ( -1.999999999999995781, 27.34374999877097068, 5.535898384862237620 ) ) ;
#9605=( BOUNDED_CURVE ( )  B_SPLINE_CURVE ( 2, ( #15564, #19469, #11497, #19850, #3525, #7962, #23655, #17513, #17775 ),
 .UNSPECIFIED., .F., .T. ) 
 B_SPLINE_CURVE_WITH_KNOTS ( ( 3, 2, 2, 2, 3 ),
 ( 0.2750000000000000222, 0.2833333333333333259, 0.2999999999999999889, 0.3166666666666666519, 0.3250000000000000111 ),
 .UNSPECIFIED. ) 
 CURVE ( )  GEOMETRIC_REPRESENTATION_ITEM ( )  RATIONAL_B_SPLINE_CURVE ( ( 0.9330127018922194093, 0.9330127018922196314, 1.000000000000000000, 0.8660254037844387076, 1.000000000000000000, 0.8660254037844387076, 1.000000000000000000, 0.9330127018922191873, 0.9330127018922194093 ) ) 
 REPRESENTATION_ITEM ( '' )  );
#9609=ADVANCED_FACE ( 'NONE', ( #23580 ), #5661, .T. ) ;
#9610=FACE_OUTER_BOUND ( 'NONE', #22921, .T. ) ;
#9614=CARTESIAN_POINT ( 'NONE',  ( -3.756430356249995661, 28.92812499938548143, 6.831223922626973533 ) ) ;
#9616=CARTESIAN_POINT ( 'NONE',  ( 1.999999999999995781, -28.69374999877096855, 5.535898384862237620 ) ) ;
#9619=CARTESIAN_POINT ( 'NONE',  ( -4.000000000000003553, -29.73213749463701561, 8.999999999999992895 ) ) ;
#9620=CARTESIAN_POINT ( 'NONE',  ( 18.87091222291602222, 18.87091222291595827, 13.61880215351699874 ) ) ;
#9621=CARTESIAN_POINT ( 'NONE',  ( 16.95054783869437642, 22.26294259461305103, 8.999999999999992895 ) ) ;
#9627=DIRECTION ( 'NONE',  ( 0.000000000000000000, 0.000000000000000000, 1.000000000000000000 ) ) ;
#9632=CARTESIAN_POINT ( 'NONE',  ( 1.999999999999995781, -25.60000000000000142, 5.535898384862237620 ) ) ;
#9638=CARTESIAN_POINT ( 'NONE',  ( 22.56362157461193618, 13.02991752792604174, 20.00001200000000168 ) ) ;
#9639=CARTESIAN_POINT ( 'NONE',  ( 0.000000000000000000, 0.000000000000000000, 19.59999999999999787 ) ) ;
#9650=CARTESIAN_POINT ( 'NONE',  ( -2.000000000000003997, -27.32500000000000284, 5.535898384862238508 ) ) ;
#9651=VECTOR ( 'NONE', #3094, 1000.000000000000000 ) ;
#9657=CARTESIAN_POINT ( 'NONE',  ( 15.30652457243565223, 20.61891932835433394, 11.16877607737301226 ) ) ;
#9665=CARTESIAN_POINT ( 'NONE',  ( -3.999999999999996447, 26.51874999877097139, 8.999999999999992895 ) ) ;
#9670=CARTESIAN_POINT ( 'NONE',  ( 0.000000000000000000, 0.000000000000000000, 19.00000000000000000 ) ) ;
#9675=EDGE_LOOP ( 'NONE', ( #6704, #14321, #19847, #8875 ) ) ;
#9676=ORIENTED_EDGE ( 'NONE', *, *, #15880, .T. ) ;
#9685=ADVANCED_FACE ( 'NONE', ( #5778 ), #17954, .F. ) ;
#9687=CARTESIAN_POINT ( 'NONE',  ( 3.756430356250002323, 29.26562499938548356, 11.16877607737301226 ) ) ;
#9690=DIRECTION ( 'NONE',  ( -0.7071067811865487940, -0.7071067811865463515, 0.000000000000000000 ) ) ;
#9693=CARTESIAN_POINT ( 'NONE',  ( 20.62100150635272300, 20.62100150635266260, 4.999999999999992006 ) ) ;
#9695=CARTESIAN_POINT ( 'NONE',  ( 3.999999999999997335, -25.65624999877097068, 11.30940107675849404 ) ) ;
#9698=CARTESIAN_POINT ( 'NONE',  ( 3.756430356250002323, 27.46562499938548640, 11.16877607737301226 ) ) ;
#9709=CARTESIAN_POINT ( 'NONE',  ( 3.756430356249997882, -26.86562499938548498, 11.16877607737301226 ) ) ;
#9719=CARTESIAN_POINT ( 'NONE',  ( 20.48178985837210320, 20.48178985837202859, 4.662447845253954171 ) ) ;
#9724=CARTESIAN_POINT ( 'NONE',  ( 4.000000000000001776, 29.01249999999999929, 11.30940107675849760 ) ) ;
#9727=CARTESIAN_POINT ( 'NONE',  ( 19.28627369086489551, 21.94247106882419729, 12.25316411605951927 ) ) ;
#9738=VECTOR ( 'NONE', #6849, 1000.000000000000000 ) ;
#9742=DIRECTION ( 'NONE',  ( 0.000000000000000000, 0.000000000000000000, -1.000000000000000000 ) ) ;
#9744=CARTESIAN_POINT ( 'NONE',  ( -4.000000000000001776, -26.76250000000000284, 11.30940107675849760 ) ) ;
#9746=DIRECTION ( 'NONE',  ( 0.000000000000000000, 1.000000000000000000, -0.000000000000000000 ) ) ;
#9752=CARTESIAN_POINT ( 'NONE',  ( 15.64473753375240506, 21.30159178324472080, 8.999999999999992895 ) ) ;
#9753=CARTESIAN_POINT ( 'NONE',  ( 19.49840572522085935, 22.15460310318015758, 5.746835883940462963 ) ) ;
#9754=CARTESIAN_POINT ( 'NONE',  ( -4.000000000000003553, -29.73213749463701561, 8.999999999999992895 ) ) ;
#9757=CARTESIAN_POINT ( 'NONE',  ( 22.10958068494259621, 20.27866814047594346, 5.206367449752296039 ) ) ;
#9759=FACE_OUTER_BOUND ( 'NONE', #15058, .T. ) ;
#9762=CARTESIAN_POINT ( 'NONE',  ( 3.999999999999997335, -27.06250000000000000, 11.30940107675849404 ) ) ;
#9767=( BOUNDED_CURVE ( )  B_SPLINE_CURVE ( 2, ( #827, #12600, #20706 ),
 .UNSPECIFIED., .F., .F. ) 
 B_SPLINE_CURVE_WITH_KNOTS ( ( 3, 3 ),
 ( 0.9889400238386636399, 1.000000000000000000 ),
 .UNSPECIFIED. ) 
 CURVE ( )  GEOMETRIC_REPRESENTATION_ITEM ( )  RATIONAL_B_SPLINE_CURVE ( ( 0.9401842259098239785, 0.9110946495778740051, 1.000000000000000000 ) ) 
 REPRESENTATION_ITEM ( '' )  );
#9769=CARTESIAN_POINT ( 'NONE',  ( 3.403349963601422168, 25.83240171513484285, 20.00001200000000523 ) ) ;
#9772=ORIENTED_EDGE ( 'NONE', *, *, #24990, .F. ) ;
#9777=FACE_OUTER_BOUND ( 'NONE', #5281, .T. ) ;
#9779=CARTESIAN_POINT ( 'NONE',  ( 20.73590635829554429, 17.90747923354928162, 5.535898384862238508 ) ) ;
#9780=CARTESIAN_POINT ( 'NONE',  ( -3.999999999999997335, 26.61250000000000071, 11.30940107675849404 ) ) ;
#9782=CARTESIAN_POINT ( 'NONE',  ( 20.77801835412135745, 15.46562359820254784, 6.831223922626973533 ) ) ;
#9783=CARTESIAN_POINT ( 'NONE',  ( 16.26787538380399312, 21.92472963329630176, 11.30940107675849404 ) ) ;
#9786=CARTESIAN_POINT ( 'NONE',  ( 0.5258040994055174222, 29.99650528990839859, 5.025965267902964939 ) ) ;
#9802=ORIENTED_EDGE ( 'NONE', *, *, #7229, .F. ) ;
#9803=CARTESIAN_POINT ( 'NONE',  ( 21.21320343559646915, 21.21320343559638744, 8.999999999999992895 ) ) ;
#9804=CARTESIAN_POINT ( 'NONE',  ( -3.834746474454188013E-15, -28.20624999877096428, 4.999999999999992006 ) ) ;
#9809=CARTESIAN_POINT ( 'NONE',  ( 20.51285331117640709, 15.20045855525759393, 8.999999999999992895 ) ) ;
#9810=CARTESIAN_POINT ( 'NONE',  ( 1.878215178125000939, 29.22812499938548569, 12.25316411605952283 ) ) ;
#9816=CARTESIAN_POINT ( 'NONE',  ( 3.999999999999996003, -27.83124999877096784, 6.690598923241487306 ) ) ;
#9817=CARTESIAN_POINT ( 'NONE',  ( 3.756430356250002323, 27.91562499938548569, 11.16877607737301226 ) ) ;
#9818=FACE_OUTER_BOUND ( 'NONE', #2981, .T. ) ;
#9826=LINE ( 'NONE', #17811, #5377 ) ;
#9828=CARTESIAN_POINT ( 'NONE',  ( 3.756430356249996994, -27.27812499938548640, 8.999999999999992895 ) ) ;
#9830=ORIENTED_EDGE ( 'NONE', *, *, #17987, .F. ) ;
#9839=CARTESIAN_POINT ( 'NONE',  ( 18.24985654912466515, 23.56225130504333976, 11.16877607737301226 ) ) ;
#9843=CARTESIAN_POINT ( 'NONE',  ( 4.000000000000003553, 27.28749999999999787, 6.690598923241489970 ) ) ;
#9845=CARTESIAN_POINT ( 'NONE',  ( 22.76675617620853131, 17.45436142028971460, 6.831223922626973533 ) ) ;
#9854=CARTESIAN_POINT ( 'NONE',  ( -3.756430356249997882, 26.86562499938548498, 11.16877607737301226 ) ) ;
#9859=ADVANCED_FACE ( 'NONE', ( #6305 ), #22516, .F. ) ;
#9860=CARTESIAN_POINT ( 'NONE',  ( 1.999999999999995781, -25.60000000000000142, 5.535898384862237620 ) ) ;
#9862=LINE ( 'NONE', #3710, #25601 ) ;
#9868=CARTESIAN_POINT ( 'NONE',  ( 2.672651547586948120E-15, 26.37812499938548427, 13.33755215474602984 ) ) ;
#9869=CARTESIAN_POINT ( 'NONE',  ( 3.999999999999995559, -28.73124999877096997, 6.690598923241487306 ) ) ;
#9870=CARTESIAN_POINT ( 'NONE',  ( 1.859271017917182139E-15, 27.08124999877096784, 12.99999999999999289 ) ) ;
#9871=CARTESIAN_POINT ( 'NONE',  ( 17.64231419060439876, 20.47074131535051933, 5.535898384862237620 ) ) ;
#9872=CARTESIAN_POINT ( 'NONE',  ( 18.64987758779700044, 21.30607496575630222, 12.25316411605951927 ) ) ;
#9873=CARTESIAN_POINT ( 'NONE',  ( -4.000000000000001776, -28.50624999877096855, 11.30940107675849760 ) ) ;
#9880=CARTESIAN_POINT ( 'NONE',  ( -3.752267015613588906E-15, -26.91250000000000142, 4.381197846482986158 ) ) ;
#9885=CARTESIAN_POINT ( 'NONE',  ( -8.377607117416806304, 24.67207871933483787, 20.00001200000000168 ) ) ;
#9893=CARTESIAN_POINT ( 'NONE',  ( 3.834746474454188013E-15, 25.56250000000000000, 4.999999999999992006 ) ) ;
#9898=CARTESIAN_POINT ( 'NONE',  ( 21.12923450446149687, 15.47238025496904612, 6.690598923241489970 ) ) ;
#9901=CARTESIAN_POINT ( 'NONE',  ( 19.63547142920491595, 16.80704430445866393, 12.46410161513774817 ) ) ;
#9903=CARTESIAN_POINT ( 'NONE',  ( -8.831537335106614961E-15, -27.13750000000000284, 12.99999999999999112 ) ) ;
#9905=( BOUNDED_CURVE ( )  B_SPLINE_CURVE ( 2, ( #23493, #3872, #17738, #7790, #3731 ),
 .UNSPECIFIED., .F., .F. ) 
 B_SPLINE_CURVE_WITH_KNOTS ( ( 3, 2, 3 ),
 ( 0.000000000000000000, 0.01666666666666666644, 0.02500000000000001180 ),
 .UNSPECIFIED. ) 
 CURVE ( )  GEOMETRIC_REPRESENTATION_ITEM ( )  RATIONAL_B_SPLINE_CURVE ( ( 1.000000000000000000, 0.8660254037844387076, 1.000000000000000000, 0.9330127018922191873, 0.9330127018922192983 ) ) 
 REPRESENTATION_ITEM ( '' )  );
#9909=CARTESIAN_POINT ( 'NONE',  ( 21.21320343559646915, 21.21320343559638744, 4.999999999999992006 ) ) ;
#9910=ORIENTED_EDGE ( 'NONE', *, *, #11672, .T. ) ;
#9911=DIRECTION ( 'NONE',  ( 0.000000000000000000, -1.000000000000000000, 0.000000000000000000 ) ) ;
#9915=ORIENTED_EDGE ( 'NONE', *, *, #18201, .F. ) ;
#9919=CARTESIAN_POINT ( 'NONE',  ( -4.000000000000003553, -29.73213749463701561, 8.999999999999992895 ) ) ;
#9920=EDGE_CURVE ( 'NONE', #22706, #24134, #25795, .T. ) ;
#9928=CARTESIAN_POINT ( 'NONE',  ( -3.756430356249996994, 27.27812499938548640, 8.999999999999992895 ) ) ;
#9929=CARTESIAN_POINT ( 'NONE',  ( 18.92274273964848064, 20.43849226750045389, 4.999999999999992006 ) ) ;
#9937=CARTESIAN_POINT ( 'NONE',  ( 3.999999999999996447, -29.66874999877096997, 8.999999999999992895 ) ) ;
#9938=CARTESIAN_POINT ( 'NONE',  ( -3.756430356249995661, 27.24062499938548498, 6.831223922626973533 ) ) ;
#9941=DIRECTION ( 'NONE',  ( 0.000000000000000000, 0.000000000000000000, -1.000000000000000000 ) ) ;
#9942=CARTESIAN_POINT ( 'NONE',  ( 1.626862140677534194E-14, 28.03750000000000497, 12.99999999999999289 ) ) ;
#9945=CARTESIAN_POINT ( 'NONE',  ( 3.834746474454188013E-15, 28.26249999999999929, 4.999999999999992006 ) ) ;
#9947=ORIENTED_EDGE ( 'NONE', *, *, #6827, .F. ) ;
#9951=CARTESIAN_POINT ( 'NONE',  ( -3.756430356250004099, -26.07812499938548356, 6.831223922626973533 ) ) ;
#9956=CARTESIAN_POINT ( 'NONE',  ( -3.756430356249996105, 26.34062499938548285, 6.831223922626973533 ) ) ;
#9961=CARTESIAN_POINT ( 'NONE',  ( 19.28854716511979461, 19.28854716511973066, 13.33755215474602984 ) ) ;
#9962=EDGE_CURVE ( 'NONE', #3427, #20963, #12746, .T. ) ;
#9965=AXIS2_PLACEMENT_3D ( 'NONE', #4958, #12939, #3003 ) ;
#9966=EDGE_CURVE ( 'NONE', #22105, #25114, #8505, .T. ) ;
#9967=CARTESIAN_POINT ( 'NONE',  ( -1.999999999999995781, 27.85000000000000142, 5.535898384862237620 ) ) ;
#9970=CARTESIAN_POINT ( 'NONE',  ( 21.67730602587931088, 19.02110864791986344, 12.25316411605952283 ) ) ;
#9977=CARTESIAN_POINT ( 'NONE',  ( 2.620986760973688460E-15, 29.78124999877096712, 13.61880215351699874 ) ) ;
#9979=LINE ( 'NONE', #13921, #6776 ) ;
#9991=CARTESIAN_POINT ( 'NONE',  ( 3.756430356250003655, 26.04062499938548569, 8.999999999999992895 ) ) ;
#9998=CARTESIAN_POINT ( 'NONE',  ( 17.23572779142213918, 22.89258204091444782, 8.999999999999992895 ) ) ;
#9999=CARTESIAN_POINT ( 'NONE',  ( 22.31370212894720240, 19.65750475098775496, 12.25316411605952283 ) ) ;
#10000=CARTESIAN_POINT ( 'NONE',  ( -4.000000000000002665, -29.73213749463701205, 9.470295877454901756 ) ) ;
#10003=CARTESIAN_POINT ( 'NONE',  ( -1.878215178125000939, -25.96562499938548285, 12.25316411605952283 ) ) ;
#10004=CARTESIAN_POINT ( 'NONE',  ( 21.91595456452976975, 19.25975718657032232, 12.25316411605952283 ) ) ;
#10008=CARTESIAN_POINT ( 'NONE',  ( -2.000000000000003997, -27.77500000000000213, 5.535898384862238508 ) ) ;
#10010=ORIENTED_EDGE ( 'NONE', *, *, #17656, .F. ) ;
#10014=FACE_OUTER_BOUND ( 'NONE', #22250, .T. ) ;
#10030=CARTESIAN_POINT ( 'NONE',  ( 17.84560739019554276, 23.50246163968784430, 6.690598923241487306 ) ) ;
#10031=FACE_OUTER_BOUND ( 'NONE', #285, .T. ) ;
#10032=CARTESIAN_POINT ( 'NONE',  ( 19.29959570814131808, 22.12802283288743155, 12.46410161513774639 ) ) ;
#10038=DIRECTION ( 'NONE',  ( -0.7071067811865487940, -0.7071067811865463515, 0.000000000000000000 ) ) ;
#10040=CARTESIAN_POINT ( 'NONE',  ( 2.000000000000003997, 29.06874999877096855, 5.535898384862238508 ) ) ;
#10044=CARTESIAN_POINT ( 'NONE',  ( 21.21320343559646915, 21.21320343559638744, 8.999999999999992895 ) ) ;
#10061=CARTESIAN_POINT ( 'NONE',  ( 1.878215178125004048, 26.11562499938548498, 5.746835883940462963 ) ) ;
#10068=CARTESIAN_POINT ( 'NONE',  ( -2.620986760973688460E-15, -28.43124999877096926, 13.61880215351699874 ) ) ;
#10070=CARTESIAN_POINT ( 'NONE',  ( 3.735045420075836212E-15, 28.51562499938549067, 4.662447845253954171 ) ) ;
#10072=CARTESIAN_POINT ( 'NONE',  ( 3.999999999999997335, -26.16250000000000142, 11.30940107675849404 ) ) ;
#10078=ORIENTED_EDGE ( 'NONE', *, *, #3191, .T. ) ;
#10081=EDGE_LOOP ( 'NONE', ( #52, #7261, #19853, #23152 ) ) ;
#10084=CARTESIAN_POINT ( 'NONE',  ( 22.75999951944203303, 17.10314526994957518, 6.690598923241489970 ) ) ;
#10088=CARTESIAN_POINT ( 'NONE',  ( -1.878215178124995832, 26.75312499938548783, 5.746835883940462963 ) ) ;
#10092=CARTESIAN_POINT ( 'NONE',  ( 18.81125008781888042, 18.81125008781880581, 4.662447845253954171 ) ) ;
#10099=CARTESIAN_POINT ( 'NONE',  ( -1.999999999999998224, 28.90000000000000213, 12.46410161513774639 ) ) ;
#10100=CARTESIAN_POINT ( 'NONE',  ( -3.756430356249997438, 28.10312499938548569, 11.16877607737301048 ) ) ;
#10101=CARTESIAN_POINT ( 'NONE',  ( 23.65168074169088186, 18.16705623898524280, 8.999999999999992895 ) ) ;
#10102=CARTESIAN_POINT ( 'NONE',  ( 21.99550407741325486, 19.33930669945380743, 12.25316411605952283 ) ) ;
#10108=VECTOR ( 'NONE', #7185, 999.9999999999998863 ) ;
#10110=ORIENTED_EDGE ( 'NONE', *, *, #3092, .F. ) ;
#10112=CARTESIAN_POINT ( 'NONE',  ( 1.878215178125004048, 25.77812499938548640, 5.746835883940462963 ) ) ;
#10119=DIRECTION ( 'NONE',  ( 0.000000000000000000, 1.000000000000000000, 0.000000000000000000 ) ) ;
#10122=CARTESIAN_POINT ( 'NONE',  ( -27.10000000000000497, -0.5999999999999998668, 19.59999999999999787 ) ) ;
#10125=CARTESIAN_POINT ( 'NONE',  ( -4.000000000000003553, -26.80000000000000071, 8.999999999999992895 ) ) ;
#10126=CARTESIAN_POINT ( 'NONE',  ( -3.137519842735244810E-15, 26.46249999999999858, 4.999999999999991118 ) ) ;
#10127=CARTESIAN_POINT ( 'NONE',  ( 3.347751660414011177, 29.81285215011482137, 11.20140010723572388 ) ) ;
#10129=LINE ( 'NONE', #8174, #20974 ) ;
#10133=CARTESIAN_POINT ( 'NONE',  ( -3.756430356250002323, -25.55312499938548498, 11.16877607737301403 ) ) ;
#10134=VECTOR ( 'NONE', #14561, 1000.000000000000000 ) ;
#10138=CARTESIAN_POINT ( 'NONE',  ( -2.620986760973688460E-15, -28.48750000000000071, 13.61880215351699874 ) ) ;
#10143=CARTESIAN_POINT ( 'NONE',  ( 1.071796769724492338, 26.20134618820330275, 12.99999999999999467 ) ) ;
#10149=CARTESIAN_POINT ( 'NONE',  ( -4.000000000000003553, -28.99374999877096926, 8.999999999999992895 ) ) ;
#10162=CARTESIAN_POINT ( 'NONE',  ( 20.72498534553237093, 15.41259058961355954, 11.16877607737301226 ) ) ;
#10163=CARTESIAN_POINT ( 'NONE',  ( 17.22246953840583217, 22.87932378789814436, 11.30940107675849404 ) ) ;
#10168=CARTESIAN_POINT ( 'NONE',  ( -0.2646063747045178660, 30.00000000000000000, 4.999999999999992895 ) ) ;
#10171=FACE_OUTER_BOUND ( 'NONE', #7251, .T. ) ;
#10172=CARTESIAN_POINT ( 'NONE',  ( -1.999999999999995781, 26.44374999877096855, 5.535898384862237620 ) ) ;
#10173=CARTESIAN_POINT ( 'NONE',  ( -3.756430356250002323, -26.45312499938548356, 11.16877607737301226 ) ) ;
#10174=DIRECTION ( 'NONE',  ( 0.000000000000000000, 0.000000000000000000, 1.000000000000000000 ) ) ;
#10182=ADVANCED_FACE ( 'NONE', ( #9397 ), #1153, .F. ) ;
#10187=CARTESIAN_POINT ( 'NONE',  ( -1.878215178124995832, 25.74062499938548498, 5.746835883940462963 ) ) ;
#10194=CARTESIAN_POINT ( 'NONE',  ( 15.30002297792396071, 20.95687722741627468, 6.690598923241487306 ) ) ;
#10195=CARTESIAN_POINT ( 'NONE',  ( 3.756430356249997882, -25.51562499938548356, 11.16877607737301226 ) ) ;
#10197=CARTESIAN_POINT ( 'NONE',  ( 3.999999999999995559, -26.08749999999999503, 6.690598923241487306 ) ) ;
#10198=CARTESIAN_POINT ( 'NONE',  ( 3.794751686895379894, -29.75919970560060079, 7.708599238039753665 ) ) ;
#10204=ORIENTED_EDGE ( 'NONE', *, *, #15730, .T. ) ;
#10210=CARTESIAN_POINT ( 'NONE',  ( 3.735045420075836212E-15, 26.71562499938548285, 4.662447845253954171 ) ) ;
#10213=EDGE_CURVE ( 'NONE', #2722, #6155, #11213, .T. ) ;
#10216=CARTESIAN_POINT ( 'NONE',  ( 18.57032807491351178, 21.22652545287281356, 12.25316411605951927 ) ) ;
#10217=DIRECTION ( 'NONE',  ( 1.000000000000000000, 0.000000000000000000, 0.000000000000000000 ) ) ;
#10221=DIRECTION ( 'NONE',  ( 0.000000000000000000, 1.000000000000000000, 0.000000000000000000 ) ) ;
#10227=VERTEX_POINT ( 'NONE', #11599 ) ;
#10232=CARTESIAN_POINT ( 'NONE',  ( 19.95366948073886348, 17.12524235599260791, 12.46410161513774817 ) ) ;
#10242=CARTESIAN_POINT ( 'NONE',  ( 1.071796769724492338, 29.35134618820330488, 12.99999999999999467 ) ) ;
#10243=CARTESIAN_POINT ( 'NONE',  ( 3.213722874945784014, 29.82775332956657266, 11.39306173506716924 ) ) ;
#10246=CARTESIAN_POINT ( 'NONE',  ( 3.756430356250003655, 25.59062499938548285, 8.999999999999992895 ) ) ;
#10249=CARTESIAN_POINT ( 'NONE',  ( 17.52740933866159168, 23.18426358815389676, 6.690598923241487306 ) ) ;
#10253=CARTESIAN_POINT ( 'NONE',  ( 4.000000000000003553, 25.00000000000000000, 8.999999999999992895 ) ) ;
#10254=CARTESIAN_POINT ( 'NONE',  ( 1.878215178124995832, -26.19062499938548427, 5.746835883940462963 ) ) ;
#10265=ORIENTED_EDGE ( 'NONE', *, *, #22721, .T. ) ;
#10267=CARTESIAN_POINT ( 'NONE',  ( 1.878215178124998497, -26.90312499938548285, 12.25316411605951927 ) ) ;
#10269=LINE ( 'NONE', #18391, #16389 ) ;
#10276=CARTESIAN_POINT ( 'NONE',  ( 20.58122674904192451, 20.58122674904186411, 4.999999999999992006 ) ) ;
#10277=CARTESIAN_POINT ( 'NONE',  ( 20.62984034111755705, 17.80141321637130147, 12.46410161513774817 ) ) ;
#10280=CARTESIAN_POINT ( 'NONE',  ( 18.65215106205190310, 18.65215106205183915, 13.33755215474602984 ) ) ;
#10281=CARTESIAN_POINT ( 'NONE',  ( 21.33252770405263732, 18.50410057930636754, 5.535898384862238508 ) ) ;
#10285=CARTESIAN_POINT ( 'NONE',  ( 3.872397317694597163, 29.74907003676636563, 7.964378325765101962 ) ) ;
#10287=ADVANCED_FACE ( 'NONE', ( #13320 ), #19333, .F. ) ;
#10288=CARTESIAN_POINT ( 'NONE',  ( -3.871726839561290490, 29.74915783848840434, 10.03836643961818886 ) ) ;
#10290=CARTESIAN_POINT ( 'NONE',  ( 17.19146985159974150, 19.84766722955904683, 5.746835883940462963 ) ) ;
#10291=CARTESIAN_POINT ( 'NONE',  ( 1.071796769724481901, -28.01740381056766438, 12.99999999999999645 ) ) ;
#10292=ORIENTED_EDGE ( 'NONE', *, *, #6643, .F. ) ;
#10294=CARTESIAN_POINT ( 'NONE',  ( -1.999999999999998224, 26.59374999877096712, 12.46410161513774639 ) ) ;
#10295=CARTESIAN_POINT ( 'NONE',  ( -3.756430356250002323, -27.35312499938547859, 11.16877607737301226 ) ) ;
#10298=EDGE_LOOP ( 'NONE', ( #1731, #13405 ) ) ;
#10306=CARTESIAN_POINT ( 'NONE',  ( -3.756430356249995661, 27.12812499938548427, 6.831223922626973533 ) ) ;
#10314=CARTESIAN_POINT ( 'NONE',  ( 3.999999999999996447, -28.76874999877096784, 8.999999999999992895 ) ) ;
#10315=LINE ( 'NONE', #20382, #13599 ) ;
#10318=CARTESIAN_POINT ( 'NONE',  ( -1.999999999999995781, 29.59374999877096712, 5.535898384862237620 ) ) ;
#10319=CARTESIAN_POINT ( 'NONE',  ( -8.000000000000000000, 10.00000000000000178, 15.00000000000000178 ) ) ;
#10332=CARTESIAN_POINT ( 'NONE',  ( -3.756430356249996994, 26.37812499938548783, 8.999999999999992895 ) ) ;
#10335=CARTESIAN_POINT ( 'NONE',  ( 16.20808571844850121, 21.52048047436717937, 6.831223922626973533 ) ) ;
#10340=CARTESIAN_POINT ( 'NONE',  ( -3.756430356249997438, 29.45312499938548356, 11.16877607737301048 ) ) ;
#10342=CARTESIAN_POINT ( 'NONE',  ( 30.00000000000000355, 3.673940397442059967E-15, 20.00000000000000000 ) ) ;
#10350=ORIENTED_EDGE ( 'NONE', *, *, #3301, .F. ) ;
#10351=CARTESIAN_POINT ( 'NONE',  ( -3.999999999999995559, 26.08749999999999503, 6.690598923241487306 ) ) ;
#10352=ORIENTED_EDGE ( 'NONE', *, *, #670, .T. ) ;
#10356=ORIENTED_EDGE ( 'NONE', *, *, #19639, .F. ) ;
#10357=CYLINDRICAL_SURFACE ( 'NONE', #23106, 4.000000000000000000 ) ;
#10365=CARTESIAN_POINT ( 'NONE',  ( -3.756430356249995661, 28.02812499938548640, 6.831223922626973533 ) ) ;
#10366=CARTESIAN_POINT ( 'NONE',  ( 20.53936981547090568, 15.22697505955208896, 6.831223922626973533 ) ) ;
#10368=VECTOR ( 'NONE', #25438, 1000.000000000000000 ) ;
#10369=CARTESIAN_POINT ( 'NONE',  ( 22.22083059878729117, 19.39240347404102849, 12.46410161513774817 ) ) ;
#10371=CARTESIAN_POINT ( 'NONE',  ( 30.00000000000000355, 3.673940397442059967E-15, 20.00000000000000000 ) ) ;
#10373=CARTESIAN_POINT ( 'NONE',  ( 3.756430356249997438, -25.40312499938548285, 11.16877607737301048 ) ) ;
#10378=CARTESIAN_POINT ( 'NONE',  ( 20.90826363534070254, 18.07983651059444696, 12.46410161513774817 ) ) ;
#10383=EDGE_CURVE ( 'NONE', #24134, #9107, #1815, .T. ) ;
#10387=EDGE_LOOP ( 'NONE', ( #16258, #15307, #22428, #20695 ) ) ;
#10389=CARTESIAN_POINT ( 'NONE',  ( 1.878215178124998497, -26.45312499938548711, 12.25316411605951927 ) ) ;
#10391=CARTESIAN_POINT ( 'NONE',  ( 4.000000000000003553, 28.13124999877096855, 6.690598923241489970 ) ) ;
#10395=AXIS2_PLACEMENT_3D ( 'NONE', #19009, #9067, #17050 ) ;
#10396=CARTESIAN_POINT ( 'NONE',  ( 23.30358785661012888, 17.64673360711768169, 11.30940107675849760 ) ) ;
#10398=CARTESIAN_POINT ( 'NONE',  ( 3.999999999999995559, -28.33750000000000213, 6.690598923241487306 ) ) ;
#10400=CARTESIAN_POINT ( 'NONE',  ( 26.00000000000000355, 3.184081677783117796E-15, 19.59999999999999787 ) ) ;
#10401=AXIS2_PLACEMENT_3D ( 'NONE', #10844, #10590, #22242 ) ;
#10403=CARTESIAN_POINT ( 'NONE',  ( 17.93393197184562027, 20.59012934980492560, 12.25316411605951927 ) ) ;
#10405=CARTESIAN_POINT ( 'NONE',  ( 19.30843454290614858, 19.30843454290607042, 4.381197846482986158 ) ) ;
#10406=CARTESIAN_POINT ( 'NONE',  ( -3.999999999999995559, 28.33750000000000213, 6.690598923241487306 ) ) ;
#10409=VECTOR ( 'NONE', #13550, 1000.000000000000000 ) ;
#10414=CARTESIAN_POINT ( 'NONE',  ( 3.999999999999995559, -27.88750000000000284, 6.690598923241487306 ) ) ;
#10416=DIRECTION ( 'NONE',  ( -0.000000000000000000, -0.000000000000000000, 1.000000000000000000 ) ) ;
#10417=CARTESIAN_POINT ( 'NONE',  ( 4.000000000000001776, 26.25624999877096499, 11.30940107675849760 ) ) ;
#10418=CARTESIAN_POINT ( 'NONE',  ( -1.878215178125000939, -26.86562499938548498, 12.25316411605952283 ) ) ;
#10425=CARTESIAN_POINT ( 'NONE',  ( -1.878215178125004048, -29.37812499938548783, 5.746835883940462963 ) ) ;
#10429=EDGE_CURVE ( 'NONE', #15184, #22105, #12592, .T. ) ;
#10431=( BOUNDED_CURVE ( )  B_SPLINE_CURVE ( 2, ( #11487, #25100, #17128, #15554, #13586, #7430, #7313, #15290, #25348 ),
 .UNSPECIFIED., .F., .F. ) 
 B_SPLINE_CURVE_WITH_KNOTS ( ( 3, 2, 2, 2, 3 ),
 ( 0.4750000000000000333, 0.4833333333333333370, 0.5000000000000000000, 0.5166666666666667185, 0.5250000000000000222 ),
 .UNSPECIFIED. ) 
 CURVE ( )  GEOMETRIC_REPRESENTATION_ITEM ( )  RATIONAL_B_SPLINE_CURVE ( ( 0.9330127018922194093, 0.9330127018922196314, 1.000000000000000000, 0.8660254037844387076, 1.000000000000000000, 0.8660254037844387076, 1.000000000000000000, 0.9330127018922194093, 0.9330127018922194093 ) ) 
 REPRESENTATION_ITEM ( '' )  );
#10434=CARTESIAN_POINT ( 'NONE',  ( -25.99307600111999150, 0.6000000000000000888, 20.00001200000000168 ) ) ;
#10436=( BOUNDED_CURVE ( )  B_SPLINE_CURVE ( 2, ( #23849, #3974, #8159, #8032, #22144, #16016, #7765, #15747, #14047 ),
 .UNSPECIFIED., .F., .F. ) 
 B_SPLINE_CURVE_WITH_KNOTS ( ( 3, 2, 2, 2, 3 ),
 ( 0.1249999999999999861, 0.1333333333333333315, 0.1499999999999999944, 0.1666666666666666574, 0.1750000000000000167 ),
 .UNSPECIFIED. ) 
 CURVE ( )  GEOMETRIC_REPRESENTATION_ITEM ( )  RATIONAL_B_SPLINE_CURVE ( ( 0.9330127018922194093, 0.9330127018922192983, 1.000000000000000000, 0.8660254037844387076, 1.000000000000000000, 0.8660254037844387076, 1.000000000000000000, 0.9330127018922191873, 0.9330127018922194093 ) ) 
 REPRESENTATION_ITEM ( '' )  );
#10441=CARTESIAN_POINT ( 'NONE',  ( -1.878215178124995832, 25.29062499938548569, 5.746835883940462963 ) ) ;
#10448=CARTESIAN_POINT ( 'NONE',  ( 18.23451611984813425, 18.23451611984805609, 12.99999999999999112 ) ) ;
#10449=CARTESIAN_POINT ( 'NONE',  ( -4.000000000000001776, -28.05624999877096926, 11.30940107675849760 ) ) ;
#10454=CARTESIAN_POINT ( 'NONE',  ( 18.07541709408115693, 18.07541709408108233, 4.999999999999992006 ) ) ;
#10465=CARTESIAN_POINT ( 'NONE',  ( 0.7500000000000001110, 0.000000000000000000, 15.00000000000000178 ) ) ;
#10466=AXIS2_PLACEMENT_3D ( 'NONE', #17259, #5467, #23516 ) ;
#10467=ORIENTED_EDGE ( 'NONE', *, *, #10740, .F. ) ;
#10470=CARTESIAN_POINT ( 'NONE',  ( 1.878215178125000939, 26.52812499938548285, 12.25316411605952283 ) ) ;
#10474=CARTESIAN_POINT ( 'NONE',  ( 21.67957950013421353, 16.36718474421539682, 11.16877607737301226 ) ) ;
#10475=EDGE_CURVE ( 'NONE', #23470, #10990, #14605, .T. ) ;
#10484=VECTOR ( 'NONE', #15137, 1000.000000000000000 ) ;
#10486=CARTESIAN_POINT ( 'NONE',  ( -3.756430356250003655, -29.69687499938548569, 8.999999999999992895 ) ) ;
#10489=ORIENTED_EDGE ( 'NONE', *, *, #9092, .F. ) ;
#10501=VERTEX_POINT ( 'NONE', #22322 ) ;
#10508=DIRECTION ( 'NONE',  ( -1.000000000000000000, 0.000000000000000000, 0.000000000000000000 ) ) ;
#10510=CARTESIAN_POINT ( 'NONE',  ( 2.672651547586948120E-15, 28.17812499938548143, 13.33755215474602984 ) ) ;
#10513=EDGE_CURVE ( 'NONE', #25114, #256, #6243, .T. ) ;
#10518=CARTESIAN_POINT ( 'NONE',  ( -3.999999999999996447, 29.21874999877096712, 8.999999999999992895 ) ) ;
#10520=CARTESIAN_POINT ( 'NONE',  ( 1.878215178124998497, -26.79062499938548214, 12.25316411605951927 ) ) ;
#10524=CARTESIAN_POINT ( 'NONE',  ( 1.999999999999998224, -28.90000000000000213, 12.46410161513774639 ) ) ;
#10527=ORIENTED_EDGE ( 'NONE', *, *, #5334, .F. ) ;
#10531=ORIENTED_EDGE ( 'NONE', *, *, #7588, .T. ) ;
#10533=CARTESIAN_POINT ( 'NONE',  ( -3.756430356250002323, -27.91562499938548569, 11.16877607737301403 ) ) ;
#10541=CARTESIAN_POINT ( 'NONE',  ( 19.34820930021694352, 19.34820930021687246, 4.999999999999992006 ) ) ;
#10542=CARTESIAN_POINT ( 'NONE',  ( 3.959305671612554781E-15, 30.00000000000000355, 12.99999999999999289 ) ) ;
#10545=CARTESIAN_POINT ( 'NONE',  ( 20.74922837557196331, 18.09303099761251588, 5.746835883940462963 ) ) ;
#10546=CARTESIAN_POINT ( 'NONE',  ( 20.90826363534070254, 18.07983651059444696, 12.46410161513774817 ) ) ;
#10548=DIRECTION ( 'NONE',  ( 0.000000000000000000, 1.000000000000000000, 0.000000000000000000 ) ) ;
#10551=CARTESIAN_POINT ( 'NONE',  ( -0.2612076306139402004, 30.00000000000001066, 12.99999999999999467 ) ) ;
#10554=CARTESIAN_POINT ( 'NONE',  ( 19.77367586078540995, 18.25792633293329104, 4.999999999999989342 ) ) ;
#10557=CARTESIAN_POINT ( 'NONE',  ( -3.999999999999997335, 25.65624999877097068, 11.30940107675849404 ) ) ;
#10558=CARTESIAN_POINT ( 'NONE',  ( -3.756430356250004099, -25.62812499938548072, 6.831223922626973533 ) ) ;
#10559=FACE_OUTER_BOUND ( 'NONE', #1278, .T. ) ;
#10560=VERTEX_POINT ( 'NONE', #10400 ) ;
#10561=CARTESIAN_POINT ( 'NONE',  ( -3.469446951953614189E-15, -30.00000000000000355, 8.999999999999992895 ) ) ;
#10564=CARTESIAN_POINT ( 'NONE',  ( -3.735045420075836212E-15, -26.15312499938548285, 4.662447845253954171 ) ) ;
#10573=CARTESIAN_POINT ( 'NONE',  ( 1.878215178125004048, 25.66562499938548569, 5.746835883940462963 ) ) ;
#10574=EDGE_CURVE ( 'NONE', #6983, #17557, #15419, .T. ) ;
#10575=CARTESIAN_POINT ( 'NONE',  ( 19.05342146176823093, 20.56917098962020418, 12.99999999999999645 ) ) ;
#10582=CARTESIAN_POINT ( 'NONE',  ( -1.878215178125000939, -26.52812499938548285, 12.25316411605952283 ) ) ;
#10586=CARTESIAN_POINT ( 'NONE',  ( 3.834746474454188013E-15, 25.95624999877096428, 4.999999999999992006 ) ) ;
#10587=CARTESIAN_POINT ( 'NONE',  ( 3.999903055931597784, -29.73215053696358368, 8.737301635141733414 ) ) ;
#10588=EDGE_LOOP ( 'NONE', ( #11044, #21090, #11372, #6057 ) ) ;
#10590=DIRECTION ( 'NONE',  ( 0.000000000000000000, -1.000000000000000000, 0.000000000000000000 ) ) ;
#10600=( BOUNDED_CURVE ( )  B_SPLINE_CURVE ( 2, ( #14379, #22338, #20361, #514, #24823, #5320, #16858, #891, #1138 ),
 .UNSPECIFIED., .F., .F. ) 
 B_SPLINE_CURVE_WITH_KNOTS ( ( 3, 2, 2, 2, 3 ),
 ( 0.02500000000000000139, 0.03333333333333333287, 0.05000000000000000278, 0.06666666666666666574, 0.07500000000000001110 ),
 .UNSPECIFIED. ) 
 CURVE ( )  GEOMETRIC_REPRESENTATION_ITEM ( )  RATIONAL_B_SPLINE_CURVE ( ( 0.9330127018922194093, 0.9330127018922194093, 1.000000000000000000, 0.8660254037844387076, 1.000000000000000000, 0.8660254037844387076, 1.000000000000000000, 0.9330127018922191873, 0.9330127018922192983 ) ) 
 REPRESENTATION_ITEM ( '' )  );
#10604=CARTESIAN_POINT ( 'NONE',  ( 1.878215178125000939, 28.32812499938548711, 12.25316411605952283 ) ) ;
#10607=CARTESIAN_POINT ( 'NONE',  ( 22.23415261606371374, 19.57795523810426630, 12.25316411605952283 ) ) ;
#10609=CARTESIAN_POINT ( 'NONE',  ( 24.67207871933483432, -8.377607117416795646, 20.00001200000000523 ) ) ;
#10614=CARTESIAN_POINT ( 'NONE',  ( 3.999999999999996447, -25.61874999877096926, 8.999999999999992895 ) ) ;
#10633=CARTESIAN_POINT ( 'NONE',  ( 1.859271017917182139E-15, 26.68750000000000000, 12.99999999999999289 ) ) ;
#10634=CARTESIAN_POINT ( 'NONE',  ( 15.93641908099185933, 21.59327333048416619, 6.690598923241487306 ) ) ;
#10636=B_SPLINE_CURVE_WITH_KNOTS ( 'NONE', 3,
 ( #18932, #24935, #9103, #7014, #15001, #1649, #1521, #15768, #17235, #21405, #21646, #23353, #5313, #9757, #17736, #25707, #15262, #3485 ),
 .UNSPECIFIED., .F., .F.,
 ( 4, 2, 2, 2, 2, 2, 2, 2, 4 ),
 ( 0.01878087663358380885, 0.01956282976579720376, 0.02034478289801060213, 0.02112673603022399704, 0.02190868916243739195, 0.02269064229465078686, 0.02347259542686418177, 0.02425454855907758014, 0.02503650169129097505 ),
 .UNSPECIFIED. ) ;
#10637=CARTESIAN_POINT ( 'NONE',  ( 1.878215178125004048, 28.36562499938548143, 5.746835883940462963 ) ) ;
#10642=CARTESIAN_POINT ( 'NONE',  ( 3.756430356249997438, -27.65312499938548640, 11.16877607737301048 ) ) ;
#10647=CARTESIAN_POINT ( 'NONE',  ( 3.999999999999996447, -29.27500000000000213, 8.999999999999992895 ) ) ;
#10649=ORIENTED_EDGE ( 'NONE', *, *, #18730, .T. ) ;
#10653=EDGE_LOOP ( 'NONE', ( #16917, #9472, #20117, #20638 ) ) ;
#10654=CARTESIAN_POINT ( 'NONE',  ( -3.735045420075836212E-15, -25.81562499938548783, 4.662447845253954171 ) ) ;
#10655=CYLINDRICAL_SURFACE ( 'NONE', #522, 4.000000000000000000 ) ;
#10656=CARTESIAN_POINT ( 'NONE',  ( -1.071796769724492338, -28.90134618820330203, 12.99999999999999467 ) ) ;
#10660=( BOUNDED_CURVE ( )  B_SPLINE_CURVE ( 2, ( #2256, #20020, #24211, #22376, #22116, #15995, #14027, #13900, #24349, #6162, #20280, #4459, #12041, #34, #12434, #18089, #424, #4070, #6431, #6299, #14417, #3955, #20401, #2124, #4204, #168, #18470, #12182, #14292, #9956, #10332, #11920, #2502, #20156, #10470, #559, #8261, #15854, #23826, #10210, #10088, #23962, #5912, #16239, #22257, #21872, #16118, #292, #19890, #8140, #18210, #1989, #24080, #17948, #4338, #12313, #14150, #8009, #21993, #2377, #18327, #8393, #6044, #16384, #10856, #13098, #8777, #18709, #3027, #19095, #16626, #4591, #2761, #1062, #12712, #5122, #23035, #12570, #22649, #20549, #2642, #21073, #10604, #4737, #6820, #22507, #18593, #14532, #10723, #20679, #3151, #941, #16901, #10997, #681, #18979, #8530, #8648, #18851, #14803, #24591, #11116, #9036, #6678, #799, #2886, #22778, #20944, #4855, #17020, #14669, #15060, #16766, #24735, #12830, #20805, #8921, #4984, #24985, #24865, #6947 ),
 .UNSPECIFIED., .F., .F. ) 
 B_SPLINE_CURVE_WITH_KNOTS ( ( 3, 2, 2, 2, 2, 2, 2, 2, 2, 2, 2, 2, 2, 2, 2, 2, 2, 2, 2, 2, 2, 2, 2, 2, 2, 2, 2, 2, 2, 2, 2, 2, 2, 2, 2, 2, 2, 2, 2, 2, 2, 2, 2, 2, 2, 2, 2, 2, 2, 2, 2, 2, 2, 2, 2, 2, 2, 2, 2, 2, 3 ),
 ( 0.000000000000000000, 0.01666666666666666644, 0.03333333333333333287, 0.05000000000000000278, 0.06666666666666666574, 0.08333333333333332871, 0.1000000000000000056, 0.1166666666666666685, 0.1333333333333333315, 0.1499999999999999944, 0.1666666666666666574, 0.1833333333333333204, 0.2000000000000000111, 0.2166666666666666741, 0.2333333333333333370, 0.2500000000000000000, 0.2666666666666666630, 0.2833333333333333259, 0.2999999999999999889, 0.3166666666666666519, 0.3333333333333333148, 0.3499999999999999778, 0.3666666666666666408, 0.3833333333333333592, 0.4000000000000000222, 0.4166666666666666852, 0.4333333333333333481, 0.4500000000000000111, 0.4666666666666666741, 0.4833333333333333370, 0.5000000000000000000, 0.5166666666666667185, 0.5333333333333333259, 0.5500000000000000444, 0.5666666666666666519, 0.5833333333333333703, 0.5999999999999999778, 0.6166666666666666963, 0.6333333333333333037, 0.6500000000000000222, 0.6666666666666666297, 0.6833333333333333481, 0.6999999999999999556, 0.7166666666666666741, 0.7333333333333332815, 0.7500000000000000000, 0.7666666666666667185, 0.7833333333333333259, 0.8000000000000000444, 0.8166666666666666519, 0.8333333333333333703, 0.8499999999999999778, 0.8666666666666666963, 0.8833333333333333037, 0.9000000000000000222, 0.9166666666666666297, 0.9333333333333333481, 0.9499999999999999556, 0.9666666666666666741, 0.9833333333333332815, 1.000000000000000000 ),
 .UNSPECIFIED. ) 
 CURVE ( )  GEOMETRIC_REPRESENTATION_ITEM ( )  RATIONAL_B_SPLINE_CURVE ( ( 1.000000000000000000, 0.8660254037844387076, 1.000000000000000000, 0.8660254037844387076, 1.000000000000000000, 0.8660254037844387076, 1.000000000000000000, 0.8660254037844387076, 1.000000000000000000, 0.8660254037844387076, 1.000000000000000000, 0.8660254037844387076, 1.000000000000000000, 0.8660254037844387076, 1.000000000000000000, 0.8660254037844387076, 1.000000000000000000, 0.8660254037844387076, 1.000000000000000000, 0.8660254037844387076, 1.000000000000000000, 0.8660254037844387076, 1.000000000000000000, 0.8660254037844387076, 1.000000000000000000, 0.8660254037844387076, 1.000000000000000000, 0.8660254037844387076, 1.000000000000000000, 0.8660254037844387076, 1.000000000000000000, 0.8660254037844387076, 1.000000000000000000, 0.8660254037844387076, 1.000000000000000000, 0.8660254037844387076, 1.000000000000000000, 0.8660254037844387076, 1.000000000000000000, 0.8660254037844387076, 1.000000000000000000, 0.8660254037844387076, 1.000000000000000000, 0.8660254037844387076, 1.000000000000000000, 0.8660254037844387076, 1.000000000000000000, 0.8660254037844387076, 1.000000000000000000, 0.8660254037844387076, 1.000000000000000000, 0.8660254037844387076, 1.000000000000000000, 0.8660254037844387076, 1.000000000000000000, 0.8660254037844387076, 1.000000000000000000, 0.8660254037844387076, 1.000000000000000000, 0.8660254037844387076, 1.000000000000000000, 0.8660254037844387076, 1.000000000000000000, 0.8660254037844387076, 1.000000000000000000, 0.8660254037844387076, 1.000000000000000000, 0.8660254037844387076, 1.000000000000000000, 0.8660254037844387076, 1.000000000000000000, 0.8660254037844387076, 1.000000000000000000, 0.8660254037844387076, 1.000000000000000000, 0.8660254037844387076, 1.000000000000000000, 0.8660254037844387076, 1.000000000000000000, 0.8660254037844387076, 1.000000000000000000, 0.8660254037844387076, 1.000000000000000000, 0.8660254037844387076, 1.000000000000000000, 0.8660254037844387076, 1.000000000000000000, 0.8660254037844387076, 1.000000000000000000, 0.8660254037844387076, 1.000000000000000000, 0.8660254037844387076, 1.000000000000000000, 0.8660254037844387076, 1.000000000000000000, 0.8660254037844387076, 1.000000000000000000, 0.8660254037844387076, 1.000000000000000000, 0.8660254037844387076, 1.000000000000000000, 0.8660254037844387076, 1.000000000000000000, 0.8660254037844387076, 1.000000000000000000, 0.8660254037844387076, 1.000000000000000000, 0.8660254037844387076, 1.000000000000000000, 0.8660254037844387076, 1.000000000000000000, 0.8660254037844387076, 1.000000000000000000, 0.8660254037844387076, 1.000000000000000000, 0.8660254037844387076, 1.000000000000000000, 0.8660254037844387076, 1.000000000000000000, 0.8660254037844387076, 1.000000000000000000 ) ) 
 REPRESENTATION_ITEM ( '' )  );
#10661=CARTESIAN_POINT ( 'NONE',  ( 3.878215178125003604, 25.32343749907822783, 8.999999999999992895 ) ) ;
#10665=CARTESIAN_POINT ( 'NONE',  ( -1.878215178124998497, 25.44062499938548427, 12.25316411605951927 ) ) ;
#10667=CARTESIAN_POINT ( 'NONE',  ( 17.21571288163933389, 22.52810763755800849, 11.16877607737301226 ) ) ;
#10668=CARTESIAN_POINT ( 'NONE',  ( 23.67481891673307715, 18.01796466724061574, 6.690598923241489970 ) ) ;
#10669=DIRECTION ( 'NONE',  ( 0.000000000000000000, 0.000000000000000000, -1.000000000000000000 ) ) ;
#10675=CARTESIAN_POINT ( 'NONE',  ( 15.57168961538060969, 20.88408437129928785, 6.831223922626973533 ) ) ;
#10678=ORIENTED_EDGE ( 'NONE', *, *, #15223, .T. ) ;
#10680=CARTESIAN_POINT ( 'NONE',  ( -1.999999999999995781, 27.34374999877097068, 5.535898384862237620 ) ) ;
#10681=CARTESIAN_POINT ( 'NONE',  ( -3.756430356250003655, -26.94062499938548427, 8.999999999999992895 ) ) ;
#10687=CARTESIAN_POINT ( 'NONE',  ( -3.756430356250004099, -26.97812499938548569, 6.831223922626973533 ) ) ;
#10690=ORIENTED_EDGE ( 'NONE', *, *, #14808, .T. ) ;
#10694=CARTESIAN_POINT ( 'NONE',  ( 2.000000000000000888, 27.62500000000000000, 12.46410161513774817 ) ) ;
#10697=CARTESIAN_POINT ( 'NONE',  ( 3.756430356250003655, 27.39062499938548356, 8.999999999999992895 ) ) ;
#10699=CARTESIAN_POINT ( 'NONE',  ( 1.057460391440397258E-14, -28.71250000000000213, 4.999999999999992006 ) ) ;
#10700=UNCERTAINTY_MEASURE_WITH_UNIT (LENGTH_MEASURE( 1.000000000000000082E-05 ), #1847, 'distance_accuracy_value', 'NONE');
#10702=LINE ( 'NONE', #6657, #24652 ) ;
#10703=CARTESIAN_POINT ( 'NONE',  ( 1.071796769724494558, 25.93615380933863435, 4.999999999999992895 ) ) ;
#10704=CARTESIAN_POINT ( 'NONE',  ( -1.071796769724487230, 28.67634618820330417, 4.999999999999992006 ) ) ;
#10705=CARTESIAN_POINT ( 'NONE',  ( -1.878215178125000939, -27.42812499938548498, 12.25316411605952283 ) ) ;
#10706=CARTESIAN_POINT ( 'NONE',  ( 1.878215178125004048, 29.37812499938548783, 5.746835883940462963 ) ) ;
#10707=DIRECTION ( 'NONE',  ( 0.000000000000000000, 1.000000000000000000, 0.000000000000000000 ) ) ;
#10708=CARTESIAN_POINT ( 'NONE',  ( -5.577813053751546416E-15, -25.33750000000000213, 12.99999999999999289 ) ) ;
#10709=CARTESIAN_POINT ( 'NONE',  ( -1.999999999999998224, 28.00000000000000000, 12.46410161513774639 ) ) ;
#10710=EDGE_LOOP ( 'NONE', ( #9354, #338, #15749, #22804, #19348, #19905 ) ) ;
#10711=CARTESIAN_POINT ( 'NONE',  ( 3.469446951953614189E-15, 30.00000000000000355, 8.999999999999992895 ) ) ;
#10713=EDGE_LOOP ( 'NONE', ( #20297, #645, #24228, #15115 ) ) ;
#10719=CARTESIAN_POINT ( 'NONE',  ( 3.469446951953614189E-15, 30.00000000000000355, 8.999999999999992895 ) ) ;
#10723=CARTESIAN_POINT ( 'NONE',  ( -1.878215178124995832, 28.55312499938548498, 5.746835883940462963 ) ) ;
#10725=DIRECTION ( 'NONE',  ( 0.000000000000000000, 0.000000000000000000, 1.000000000000000000 ) ) ;
#10726=CARTESIAN_POINT ( 'NONE',  ( 19.10065816080342671, 21.75685553876272493, 5.746835883940462963 ) ) ;
#10729=CARTESIAN_POINT ( 'NONE',  ( 25.83240171513484285, -3.403349963601437267, 20.00001200000000168 ) ) ;
#10732=CARTESIAN_POINT ( 'NONE',  ( -1.071796769724481901, 27.96115380933863293, 12.99999999999999645 ) ) ;
#10733=CARTESIAN_POINT ( 'NONE',  ( 2.620986760973688460E-15, 29.38749999999999929, 13.61880215351699874 ) ) ;
#10734=( BOUNDED_CURVE ( )  B_SPLINE_CURVE ( 2, ( #10276, #1934, #11736, #4141, #21811, #24142, #23639, #356, #11981 ),
 .UNSPECIFIED., .F., .F. ) 
 B_SPLINE_CURVE_WITH_KNOTS ( ( 3, 2, 2, 2, 3 ),
 ( 0.8250000000000000666, 0.8333333333333333703, 0.8499999999999999778, 0.8666666666666666963, 0.8750000000000000000 ),
 .UNSPECIFIED. ) 
 CURVE ( )  GEOMETRIC_REPRESENTATION_ITEM ( )  RATIONAL_B_SPLINE_CURVE ( ( 0.9330127018922194093, 0.9330127018922198534, 1.000000000000000000, 0.8660254037844387076, 1.000000000000000000, 0.8660254037844387076, 1.000000000000000000, 0.9330127018922194093, 0.9330127018922194093 ) ) 
 REPRESENTATION_ITEM ( '' )  );
#10737=CARTESIAN_POINT ( 'NONE',  ( -1.071796769724494558, -28.24240381056766580, 4.999999999999992895 ) ) ;
#10740=EDGE_CURVE ( 'NONE', #19876, #20539, #22789, .T. ) ;
#10743=( BOUNDED_CURVE ( )  B_SPLINE_CURVE ( 2, ( #12786, #11327, #3352, #13048, #15264, #8869, #13294, #1405, #23232 ),
 .UNSPECIFIED., .F., .F. ) 
 B_SPLINE_CURVE_WITH_KNOTS ( ( 3, 2, 2, 2, 3 ),
 ( 0.5750000000000000666, 0.5833333333333333703, 0.5999999999999999778, 0.6166666666666666963, 0.6250000000000000000 ),
 .UNSPECIFIED. ) 
 CURVE ( )  GEOMETRIC_REPRESENTATION_ITEM ( )  RATIONAL_B_SPLINE_CURVE ( ( 0.9330127018922194093, 0.9330127018922198534, 1.000000000000000000, 0.8660254037844387076, 1.000000000000000000, 0.8660254037844387076, 1.000000000000000000, 0.9330127018922194093, 0.9330127018922194093 ) ) 
 REPRESENTATION_ITEM ( '' )  );
#10745=DIRECTION ( 'NONE',  ( 0.000000000000000000, 0.000000000000000000, 1.000000000000000000 ) ) ;
#10747=CARTESIAN_POINT ( 'NONE',  ( 3.756430356249997882, -25.96562499938548640, 11.16877607737301226 ) ) ;
#10748=VERTEX_POINT ( 'NONE', #4865 ) ;
#10752=EDGE_CURVE ( 'NONE', #125, #21679, #10867, .T. ) ;
#10758=CARTESIAN_POINT ( 'NONE',  ( 16.92403133439988139, 22.23642609031855244, 6.831223922626973533 ) ) ;
#10761=CARTESIAN_POINT ( 'NONE',  ( 2.672651547586948120E-15, 29.07812499938548001, 13.33755215474602984 ) ) ;
#10762=CARTESIAN_POINT ( 'NONE',  ( 16.74068927859332234, 19.39688665655263122, 12.25316411605951927 ) ) ;
#10768=CARTESIAN_POINT ( 'NONE',  ( -3.756430356250003655, -26.94062499938548427, 8.999999999999992895 ) ) ;
#10771=CYLINDRICAL_SURFACE ( 'NONE', #5436, 4.000000000000000000 ) ;
#10777=EDGE_LOOP ( 'NONE', ( #2783, #11141, #12205, #22891 ) ) ;
#10778=CARTESIAN_POINT ( 'NONE',  ( -1.878215178125000939, -26.07812499938548356, 12.25316411605952283 ) ) ;
#10783=ADVANCED_FACE ( 'NONE', ( #21084 ), #1755, .F. ) ;
#10786=VECTOR ( 'NONE', #18549, 1000.000000000000000 ) ;
#10788=VECTOR ( 'NONE', #24147, 1000.000000000000000 ) ;
#10790=CARTESIAN_POINT ( 'NONE',  ( 3.999999999999996447, -28.37500000000000000, 8.999999999999992895 ) ) ;
#10794=CARTESIAN_POINT ( 'NONE',  ( -3.756430356249996105, 25.32812499938548356, 6.831223922626973533 ) ) ;
#10797=CARTESIAN_POINT ( 'NONE',  ( 21.73261250872320716, 16.42021775280438689, 6.831223922626973533 ) ) ;
#10798=CARTESIAN_POINT ( 'NONE',  ( 23.93998395967802750, 18.28312971018556965, 11.30940107675849760 ) ) ;
#10803=CARTESIAN_POINT ( 'NONE',  ( 19.79463422097012426, 17.13843684301067682, 5.746835883940462963 ) ) ;
#10804=CARTESIAN_POINT ( 'NONE',  ( 3.469446951953614189E-15, 30.00000000000000355, 8.999999999999992895 ) ) ;
#10807=CARTESIAN_POINT ( 'NONE',  ( -3.999999999999996003, 26.93124999877096926, 6.690598923241487306 ) ) ;
#10808=CARTESIAN_POINT ( 'NONE',  ( -3.756430356250002323, -27.80312499938548143, 11.16877607737301226 ) ) ;
#10811=CARTESIAN_POINT ( 'NONE',  ( 3.959305671612554781E-15, 30.00000000000000355, 12.99999999999999289 ) ) ;
#10814=CARTESIAN_POINT ( 'NONE',  ( -1.878215178125004048, -26.11562499938548498, 5.746835883940462963 ) ) ;
#10815=ORIENTED_EDGE ( 'NONE', *, *, #2794, .F. ) ;
#10827=CARTESIAN_POINT ( 'NONE',  ( 3.756430356250003655, 27.84062499938548640, 8.999999999999992895 ) ) ;
#10828=CARTESIAN_POINT ( 'NONE',  ( 22.00869856443133088, 19.18027143968506465, 5.535898384862238508 ) ) ;
#10832=CARTESIAN_POINT ( 'NONE',  ( 3.469446951953614189E-15, 30.00000000000000355, 8.999999999999992895 ) ) ;
#10834=CARTESIAN_POINT ( 'NONE',  ( 17.67766952966372429, 17.67766952966365679, 8.999999999999992895 ) ) ;
#10835=CARTESIAN_POINT ( 'NONE',  ( -2.672651547586948120E-15, -27.84062499938548640, 13.33755215474602984 ) ) ;
#10842=CARTESIAN_POINT ( 'NONE',  ( -2.000000000000003997, -28.67500000000000426, 5.535898384862238508 ) ) ;
#10843=VERTEX_POINT ( 'NONE', #13587 ) ;
#10844=CARTESIAN_POINT ( 'NONE',  ( -3.469446951953614189E-15, -25.00000000000000000, 8.999999999999992895 ) ) ;
#10856=CARTESIAN_POINT ( 'NONE',  ( -1.878215178124995832, 27.65312499938548640, 5.746835883940462963 ) ) ;
#10860=CARTESIAN_POINT ( 'NONE',  ( 22.56362157461194329, -13.02991752792603819, 20.00001200000000523 ) ) ;
#10863=EDGE_CURVE ( 'NONE', #22864, #5788, #11539, .T. ) ;
#10867=LINE ( 'NONE', #18867, #18018 ) ;
#10871=VERTEX_POINT ( 'NONE', #5991 ) ;
#10875=ORIENTED_EDGE ( 'NONE', *, *, #5541, .F. ) ;
#10878=CARTESIAN_POINT ( 'NONE',  ( -3.756430356250004099, -26.64062499938549067, 6.831223922626973533 ) ) ;
#10880=CARTESIAN_POINT ( 'NONE',  ( 3.469446951953614189E-15, 30.00000000000000355, 8.999999999999992895 ) ) ;
#10882=ORIENTED_EDGE ( 'NONE', *, *, #15492, .T. ) ;
#10889=CARTESIAN_POINT ( 'NONE',  ( -1.071796769724481901, 28.41115380933862866, 12.99999999999999645 ) ) ;
#10890=CARTESIAN_POINT ( 'NONE',  ( 19.68629472953723436, 19.68629472953716686, 13.33755215474602984 ) ) ;
#10893=CARTESIAN_POINT ( 'NONE',  ( 1.878215178125000939, 27.76562499938548356, 12.25316411605952283 ) ) ;
#10894=( BOUNDED_CURVE ( )  B_SPLINE_CURVE ( 2, ( #11009, #5134, #3159, #9434, #9172 ),
 .UNSPECIFIED., .F., .F. ) 
 B_SPLINE_CURVE_WITH_KNOTS ( ( 3, 2, 3 ),
 ( 0.9749999999999999778, 0.9833333333333332815, 1.000000000000000000 ),
 .UNSPECIFIED. ) 
 CURVE ( )  GEOMETRIC_REPRESENTATION_ITEM ( )  RATIONAL_B_SPLINE_CURVE ( ( 0.9330127018922194093, 0.9330127018922194093, 1.000000000000000000, 0.8660254037844387076, 1.000000000000000000 ) ) 
 REPRESENTATION_ITEM ( '' )  );
#10896=CARTESIAN_POINT ( 'NONE',  ( 20.40451381974352074, 17.74831644178408041, 12.25316411605952283 ) ) ;
#10902=B_SPLINE_CURVE_WITH_KNOTS ( 'NONE', 3,
 ( #21041, #19443, #16985, #7029, #1030, #3231, #24949, #9006, #15017, #13451, #7546, #7300, #3501, #7416, #1146, #3117, #17109, #9118, #9391, #5327, #22997, #10959, #21420, #11473, #15279, #5082, #11082, #1537, #19063, #25084, #7171, #11202, #15160, #5211 ),
 .UNSPECIFIED., .F., .F.,
 ( 4, 2, 2, 2, 2, 2, 2, 2, 2, 2, 2, 2, 2, 2, 2, 2, 4 ),
 ( 0.000000000000000000, 0.0007824850735655044642, 0.001564970147131008928, 0.002347455220696513176, 0.003129940294262017857, 0.003912425367827522538, 0.004694910441393026351, 0.005477395514958531032, 0.006259880588524035713, 0.007042365662089540394, 0.007824850735655045075, 0.008607335809220548889, 0.009389820882786052703, 0.01017230595635155825, 0.01095479102991706206, 0.01173727610348256761, 0.01251976117704807143 ),
 .UNSPECIFIED. ) ;
#10904=CARTESIAN_POINT ( 'NONE',  ( -1.878215178125000939, -27.31562499938548427, 12.25316411605952283 ) ) ;
#10908=CARTESIAN_POINT ( 'NONE',  ( 0.2902671272941750868, 30.00000000000000355, 12.99999999999999112 ) ) ;
#10911=ORIENTED_EDGE ( 'NONE', *, *, #15065, .T. ) ;
#10912=ORIENTED_EDGE ( 'NONE', *, *, #20906, .F. ) ;
#10913=DIRECTION ( 'NONE',  ( 0.000000000000000000, 0.000000000000000000, -1.000000000000000000 ) ) ;
#10916=ORIENTED_EDGE ( 'NONE', *, *, #6754, .T. ) ;
#10917=B_SPLINE_CURVE_WITH_KNOTS ( 'NONE', 3,
 ( #18306, #12811, #20783, #18827, #2356, #8509, #916, #777, #16742, #24710 ),
 .UNSPECIFIED., .F., .F.,
 ( 4, 2, 2, 2, 4 ),
 ( 0.01251976117704807143, 0.01338929815772731124, 0.01425883513840654933, 0.01512837211908578741, 0.01599790909976502723 ),
 .UNSPECIFIED. ) ;
#10918=CARTESIAN_POINT ( 'NONE',  ( 3.756430356249996994, -29.07812499938548356, 8.999999999999992895 ) ) ;
#10923=CARTESIAN_POINT ( 'NONE',  ( -1.071796769724494558, -26.38615380933864074, 4.999999999999992895 ) ) ;
#10931=VECTOR ( 'NONE', #22270, 1000.000000000000000 ) ;
#10933=CARTESIAN_POINT ( 'NONE',  ( 3.735045420075836212E-15, 25.25312499938548427, 4.662447845253954171 ) ) ;
#10935=CARTESIAN_POINT ( 'NONE',  ( 20.50609665440990526, 14.84924240491746339, 8.999999999999992895 ) ) ;
#10936=CARTESIAN_POINT ( 'NONE',  ( 21.81216202160668871, 16.49976726568787200, 6.831223922626973533 ) ) ;
#10942=CARTESIAN_POINT ( 'NONE',  ( 22.31597560320210505, 17.00358084728328478, 11.16877607737301403 ) ) ;
#10946=CARTESIAN_POINT ( 'NONE',  ( 4.000000000000001776, 27.15624999877097423, 11.30940107675849760 ) ) ;
#10947=CARTESIAN_POINT ( 'NONE',  ( 3.756430356249996994, -28.51562499938548356, 8.999999999999992895 ) ) ;
#10949=CARTESIAN_POINT ( 'NONE',  ( 5.577813053751546416E-15, 25.73124999877097352, 12.99999999999999289 ) ) ;
#10952=CARTESIAN_POINT ( 'NONE',  ( 18.67203843983824996, 18.67203843983818246, 4.999999999999991118 ) ) ;
#10956=CARTESIAN_POINT ( 'NONE',  ( 1.878215178124995832, -27.09062499938548640, 5.746835883940462963 ) ) ;
#10959=CARTESIAN_POINT ( 'NONE',  ( 18.51809052069471306, 23.60276563550342388, 10.77252090037689136 ) ) ;
#10965=CARTESIAN_POINT ( 'NONE',  ( 23.26836714124207361, 18.93629030671969460, 11.57226653943512851 ) ) ;
#10966=CARTESIAN_POINT ( 'NONE',  ( -3.756430356249995661, 28.02812499938548640, 6.831223922626973533 ) ) ;
#10969=CARTESIAN_POINT ( 'NONE',  ( 1.071796769724493448, -28.73259618943232852, 4.999999999999995559 ) ) ;
#10972=CYLINDRICAL_SURFACE ( 'NONE', #4967, 4.000000000000000000 ) ;
#10976=CYLINDRICAL_SURFACE ( 'NONE', #17212, 4.000000000000000000 ) ;
#10977=CARTESIAN_POINT ( 'NONE',  ( -1.878215178125000939, -27.87812499938548427, 12.25316411605952283 ) ) ;
#10981=CARTESIAN_POINT ( 'NONE',  ( -24.00000000000000355, 2.939152317953648289E-15, 19.00000000000000000 ) ) ;
#10983=CARTESIAN_POINT ( 'NONE',  ( 2.440392720584789288, -29.90136469312441037, 12.17998752022640296 ) ) ;
#10984=ORIENTED_EDGE ( 'NONE', *, *, #14381, .F. ) ;
#10985=CARTESIAN_POINT ( 'NONE',  ( 20.47307855473466631, 15.16068379881585138, 8.999999999999992895 ) ) ;
#10988=EDGE_CURVE ( 'NONE', #22563, #446, #17941, .T. ) ;
#10990=VERTEX_POINT ( 'NONE', #4532 ) ;
#10994=CARTESIAN_POINT ( 'NONE',  ( -1.626862140677534194E-14, -27.58750000000000213, 12.99999999999999289 ) ) ;
#10997=CARTESIAN_POINT ( 'NONE',  ( 2.672651547586948120E-15, 28.74062499938548854, 13.33755215474603162 ) ) ;
#11002=CARTESIAN_POINT ( 'NONE',  ( 8.000000000000000000, 10.00000000000000000, 17.00000000000000000 ) ) ;
#11003=CARTESIAN_POINT ( 'NONE',  ( 1.878215178125000939, 25.62812499938548783, 12.25316411605952283 ) ) ;
#11007=CARTESIAN_POINT ( 'NONE',  ( -3.878215178125003604, -25.07031249969274356, 8.999999999999992895 ) ) ;
#11009=CARTESIAN_POINT ( 'NONE',  ( -1.859271017917182139E-15, -29.38749999999999929, 12.99999999999999289 ) ) ;
#11012=LINE ( 'NONE', #21086, #16222 ) ;
#11016=ORIENTED_EDGE ( 'NONE', *, *, #21604, .T. ) ;
#11021=DIRECTION ( 'NONE',  ( 0.000000000000000000, 0.000000000000000000, 1.000000000000000000 ) ) ;
#11030=CARTESIAN_POINT ( 'NONE',  ( 19.76811771667562567, 17.11192033871618534, 12.25316411605952283 ) ) ;
#11033=CARTESIAN_POINT ( 'NONE',  ( 4.000000000000001776, 25.41250000000000142, 11.30940107675849760 ) ) ;
#11034=CARTESIAN_POINT ( 'NONE',  ( 19.84539375530421168, 19.84539375530412997, 4.662447845253954171 ) ) ;
#11038=CARTESIAN_POINT ( 'NONE',  ( -3.756430356250002323, -26.90312499938548285, 11.16877607737301403 ) ) ;
#11044=ORIENTED_EDGE ( 'NONE', *, *, #24557, .T. ) ;
#11045=DIRECTION ( 'NONE',  ( 0.000000000000000000, -1.000000000000000000, 0.000000000000000000 ) ) ;
#11047=CARTESIAN_POINT ( 'NONE',  ( 19.46753356867312235, 19.46753356867304063, 12.99999999999999112 ) ) ;
#11048=VERTEX_POINT ( 'NONE', #16460 ) ;
#11049=CARTESIAN_POINT ( 'NONE',  ( -3.756430356250003655, -28.40312499938548640, 8.999999999999992895 ) ) ;
#11050=DIRECTION ( 'NONE',  ( 0.000000000000000000, 1.000000000000000000, 0.000000000000000000 ) ) ;
#11059=EDGE_CURVE ( 'NONE', #25112, #2876, #22977, .T. ) ;
#11060=LINE ( 'NONE', #5055, #10409 ) ;
#11062=CARTESIAN_POINT ( 'NONE',  ( -3.756430356249996994, 25.81562499938548427, 8.999999999999992895 ) ) ;
#11064=CARTESIAN_POINT ( 'NONE',  ( 15.30002297792396071, 20.95687722741627468, 6.690598923241487306 ) ) ;
#11065=CARTESIAN_POINT ( 'NONE',  ( 22.28712185865447637, 19.45869473390820659, 5.535898384862238508 ) ) ;
#11069=CARTESIAN_POINT ( 'NONE',  ( 15.94292067550354730, 21.25531543142222901, 11.16877607737301048 ) ) ;
#11070=DIRECTION ( 'NONE',  ( 0.000000000000000000, 0.000000000000000000, 1.000000000000000000 ) ) ;
#11073=CARTESIAN_POINT ( 'NONE',  ( 4.000000000000003553, 28.58124999877096784, 6.690598923241489970 ) ) ;
#11074=CARTESIAN_POINT ( 'NONE',  ( -2.000000000000000888, -25.37500000000000000, 12.46410161513774817 ) ) ;
#11079=CARTESIAN_POINT ( 'NONE',  ( 1.878215178124995832, -27.99062499938548143, 5.746835883940462963 ) ) ;
#11082=CARTESIAN_POINT ( 'NONE',  ( 19.41783949975652845, 22.86907598272403419, 12.17998752022640474 ) ) ;
#11091=CARTESIAN_POINT ( 'NONE',  ( -1.878215178124995832, 29.34062499938548285, 5.746835883940462963 ) ) ;
#11092=EDGE_CURVE ( 'NONE', #7736, #24890, #22451, .T. ) ;
#11097=CARTESIAN_POINT ( 'NONE',  ( -1.859271017917182139E-15, -25.78750000000000142, 12.99999999999999289 ) ) ;
#11101=CARTESIAN_POINT ( 'NONE',  ( -1.878215178125000939, -26.07812499938548356, 12.25316411605952283 ) ) ;
#11105=CARTESIAN_POINT ( 'NONE',  ( -1.071796769724487675, -28.69240381056766509, 4.999999999999988454 ) ) ;
#11116=CARTESIAN_POINT ( 'NONE',  ( -3.756430356249996105, 29.04062499938548569, 6.831223922626973533 ) ) ;
#11120=CARTESIAN_POINT ( 'NONE',  ( 1.859271017917182139E-15, 29.38749999999999929, 12.99999999999999289 ) ) ;
#11121=CARTESIAN_POINT ( 'NONE',  ( 2.672651547586948120E-15, 25.59062499938548640, 13.33755215474602984 ) ) ;
#11123=CARTESIAN_POINT ( 'NONE',  ( 25.16843286583315020, -6.741346781237215424, 20.00001200000000168 ) ) ;
#11126=CARTESIAN_POINT ( 'NONE',  ( 21.21320343559646915, 21.21320343559638744, 8.999999999999992895 ) ) ;
#11132=CARTESIAN_POINT ( 'NONE',  ( -1.071796769724494336, -25.35759618943234628, 12.99999999999999467 ) ) ;
#11138=CARTESIAN_POINT ( 'NONE',  ( -2.672651547586948120E-15, -26.49062499938548143, 13.33755215474602984 ) ) ;
#11141=ORIENTED_EDGE ( 'NONE', *, *, #6265, .T. ) ;
#11147=CARTESIAN_POINT ( 'NONE',  ( 16.63234978716043244, 21.94474454307910705, 8.999999999999992895 ) ) ;
#11150=CARTESIAN_POINT ( 'NONE',  ( 2.620986760973688460E-15, 26.23750000000000071, 13.61880215351699874 ) ) ;
#11152=CARTESIAN_POINT ( 'NONE',  ( 20.19238178538755690, 17.53618440742811302, 5.746835883940462963 ) ) ;
#11153=CARTESIAN_POINT ( 'NONE',  ( 4.000000000000001776, 26.70624999877097139, 11.30940107675849760 ) ) ;
#11162=ORIENTED_EDGE ( 'NONE', *, *, #14205, .T. ) ;
#11168=CARTESIAN_POINT ( 'NONE',  ( 3.756430356249997438, -28.21562499938548640, 11.16877607737301048 ) ) ;
#11175=DIRECTION ( 'NONE',  ( -0.7071067811865487940, -0.7071067811865463515, 0.000000000000000000 ) ) ;
#11177=EDGE_CURVE ( 'NONE', #1111, #1657, #20610, .T. ) ;
#11178=AXIS2_PLACEMENT_3D ( 'NONE', #25381, #13621, #7849 ) ;
#11179=CARTESIAN_POINT ( 'NONE',  ( 2.672651547586948120E-15, 27.72812499938548569, 13.33755215474603162 ) ) ;
#11180=CARTESIAN_POINT ( 'NONE',  ( -3.182002658620821212, -29.83112730774910659, 6.562149109989046103 ) ) ;
#11181=CARTESIAN_POINT ( 'NONE',  ( 19.67524618651571799, 16.84681906176946242, 12.46410161513774817 ) ) ;
#11182=CARTESIAN_POINT ( 'NONE',  ( 21.05852382634284936, 21.05852382634278186, 13.61880215351699874 ) ) ;
#11183=CARTESIAN_POINT ( 'NONE',  ( 18.24657187926979063, 19.76232140712176744, 4.999999999999992895 ) ) ;
#11187=CARTESIAN_POINT ( 'NONE',  ( 18.46426205773553164, 21.12045943569482986, 5.746835883940462963 ) ) ;
#11188=CARTESIAN_POINT ( 'NONE',  ( 20.89942480057588980, 20.89942480057579033, 4.999999999999992006 ) ) ;
#11190=EDGE_LOOP ( 'NONE', ( #11681, #15944, #5389, #25681 ) ) ;
#11192=CARTESIAN_POINT ( 'NONE',  ( 3.756430356250004099, 25.29062499938548569, 6.831223922626973533 ) ) ;
#11193=CARTESIAN_POINT ( 'NONE',  ( 3.756430356249997882, -29.45312499938548356, 11.16877607737301226 ) ) ;
#11198=CARTESIAN_POINT ( 'NONE',  ( 3.756430356249995661, -27.57812499938548356, 6.831223922626973533 ) ) ;
#11202=CARTESIAN_POINT ( 'NONE',  ( 20.83838200801861973, 21.58304260418841380, 12.97381592328244082 ) ) ;
#11204=VECTOR ( 'NONE', #3247, 1000.000000000000000 ) ;
#11211=LINE ( 'NONE', #25226, #16795 ) ;
#11213=LINE ( 'NONE', #17379, #23028 ) ;
#11218=CARTESIAN_POINT ( 'NONE',  ( 0.000000000000000000, 0.000000000000000000, 19.00000000000000000 ) ) ;
#11219=CARTESIAN_POINT ( 'NONE',  ( -3.756430356250002323, -29.26562499938548356, 11.16877607737301226 ) ) ;
#11222=ADVANCED_FACE ( 'NONE', ( #19044 ), #9245, .F. ) ;
#11234=AXIS2_PLACEMENT_3D ( 'NONE', #1302, #15179, #25238 ) ;
#11237=EDGE_CURVE ( 'NONE', #14695, #22241, #23279, .T. ) ;
#11239=DIRECTION ( 'NONE',  ( -0.7071067811865487940, -0.7071067811865463515, 0.000000000000000000 ) ) ;
#11245=CARTESIAN_POINT ( 'NONE',  ( 3.735045420075836212E-15, 26.26562499938548356, 4.662447845253954171 ) ) ;
#11248=CARTESIAN_POINT ( 'NONE',  ( 1.626862140677534194E-14, 28.43124999877096570, 12.99999999999999289 ) ) ;
#11252=CARTESIAN_POINT ( 'NONE',  ( 20.42212772327495784, 20.42212772327488679, 12.99999999999999289 ) ) ;
#11253=CARTESIAN_POINT ( 'NONE',  ( 1.999999999999995781, -27.79374999877096997, 5.535898384862237620 ) ) ;
#11257=DIRECTION ( 'NONE',  ( 0.000000000000000000, 1.000000000000000000, 0.000000000000000000 ) ) ;
#11258=ORIENTED_EDGE ( 'NONE', *, *, #769, .T. ) ;
#11259=CARTESIAN_POINT ( 'NONE',  ( -1.071796769724492338, -28.95759618943233704, 12.99999999999999467 ) ) ;
#11260=EDGE_LOOP ( 'NONE', ( #11162, #20574, #9116, #19117 ) ) ;
#11263=ORIENTED_EDGE ( 'NONE', *, *, #24863, .T. ) ;
#11264=CARTESIAN_POINT ( 'NONE',  ( -3.756430356250002323, -28.81562499938548427, 11.16877607737301226 ) ) ;
#11273=CARTESIAN_POINT ( 'NONE',  ( 0.000000000000000000, 10.00000000000000000, 13.00000000000000178 ) ) ;
#11275=VECTOR ( 'NONE', #20729, 1000.000000000000000 ) ;
#11278=CARTESIAN_POINT ( 'NONE',  ( 20.51057983692150444, 17.85438245896205700, 5.746835883940462963 ) ) ;
#11279=( BOUNDED_CURVE ( )  B_SPLINE_CURVE ( 2, ( #6176, #16525, #12198, #24485, #22526, #4607, #957, #24752, #13366 ),
 .UNSPECIFIED., .F., .F. ) 
 B_SPLINE_CURVE_WITH_KNOTS ( ( 3, 2, 2, 2, 3 ),
 ( 0.4750000000000000333, 0.4833333333333333370, 0.5000000000000000000, 0.5166666666666667185, 0.5250000000000000222 ),
 .UNSPECIFIED. ) 
 CURVE ( )  GEOMETRIC_REPRESENTATION_ITEM ( )  RATIONAL_B_SPLINE_CURVE ( ( 0.9330127018922194093, 0.9330127018922196314, 1.000000000000000000, 0.8660254037844387076, 1.000000000000000000, 0.8660254037844387076, 1.000000000000000000, 0.9330127018922194093, 0.9330127018922194093 ) ) 
 REPRESENTATION_ITEM ( '' )  );
#11283=CARTESIAN_POINT ( 'NONE',  ( -1.999999999999995781, 25.15000000000000213, 5.535898384862237620 ) ) ;
#11286=CARTESIAN_POINT ( 'NONE',  ( 15.96943717979804056, 21.28183193571671694, 6.831223922626973533 ) ) ;
#11291=CARTESIAN_POINT ( 'NONE',  ( 1.071796769724498999, 28.05759618943233491, 12.99999999999998757 ) ) ;
#11293=DIRECTION ( 'NONE',  ( 0.000000000000000000, 0.000000000000000000, -1.000000000000000000 ) ) ;
#11299=CYLINDRICAL_SURFACE ( 'NONE', #22517, 4.000000000000000000 ) ;
#11304=EDGE_LOOP ( 'NONE', ( #9086, #15654, #2370, #10204 ) ) ;
#11306=CARTESIAN_POINT ( 'NONE',  ( -2.672651547586948120E-15, -29.64062499938548356, 13.33755215474603162 ) ) ;
#11318=CARTESIAN_POINT ( 'NONE',  ( -3.756430356249996105, 25.77812499938548285, 6.831223922626973533 ) ) ;
#11320=CARTESIAN_POINT ( 'NONE',  ( 17.79907597611823533, 23.11147073203690283, 6.831223922626973533 ) ) ;
#11321=CARTESIAN_POINT ( 'NONE',  ( 22.10157009459123856, 19.44537271663178757, 5.746835883940462963 ) ) ;
#11322=CARTESIAN_POINT ( 'NONE',  ( 19.37161951330217136, 20.88736904115415172, 12.99999999999999289 ) ) ;
#11326=CARTESIAN_POINT ( 'NONE',  ( 17.50739442887878639, 22.81978918479745744, 8.999999999999992895 ) ) ;
#11327=CARTESIAN_POINT ( 'NONE',  ( 20.55781653595669667, 19.04206700810457065, 12.99999999999998757 ) ) ;
#11330=CARTESIAN_POINT ( 'NONE',  ( 4.000000000000003553, 29.48124999877096997, 6.690598923241489970 ) ) ;
#11331=CARTESIAN_POINT ( 'NONE',  ( -4.000000000000003553, -25.03749999999999787, 6.690598923241489970 ) ) ;
#11332=LINE ( 'NONE', #11848, #20371 ) ;
#11333=ORIENTED_EDGE ( 'NONE', *, *, #23220, .T. ) ;
#11336=CARTESIAN_POINT ( 'NONE',  ( 26.00000000000000711, 1.701696020694481559, 20.00001200000000523 ) ) ;
#11337=CARTESIAN_POINT ( 'NONE',  ( -3.756430356250002323, -27.80312499938548143, 11.16877607737301226 ) ) ;
#11350=CARTESIAN_POINT ( 'NONE',  ( 3.999999999999995559, -27.38124999877096855, 6.690598923241487306 ) ) ;
#11354=CARTESIAN_POINT ( 'NONE',  ( -3.959305739469038251E-15, -30.00000000000000355, 12.99999999999999289 ) ) ;
#11357=FACE_OUTER_BOUND ( 'NONE', #23816, .T. ) ;
#11360=CARTESIAN_POINT ( 'NONE',  ( 1.878215178124995832, -29.45312499938548356, 5.746835883940462963 ) ) ;
#11362=CARTESIAN_POINT ( 'NONE',  ( -3.756430356250003655, -25.14062499938548356, 8.999999999999992895 ) ) ;
#11372=ORIENTED_EDGE ( 'NONE', *, *, #3328, .F. ) ;
#11379=EDGE_CURVE ( 'NONE', #7733, #20732, #4410, .T. ) ;
#11382=EDGE_CURVE ( 'NONE', #5606, #990, #19932, .T. ) ;
#11387=CARTESIAN_POINT ( 'NONE',  ( -3.756430356249996994, 27.72812499938548569, 8.999999999999992895 ) ) ;
#11388=CARTESIAN_POINT ( 'NONE',  ( 4.000000000000003553, 29.73213749463701561, 8.999999999999992895 ) ) ;
#11389=CARTESIAN_POINT ( 'NONE',  ( 19.61779375967526562, 22.44622088442137908, 12.46410161513774639 ) ) ;
#11395=CARTESIAN_POINT ( 'NONE',  ( -4.000000000000003553, -26.74374999877096926, 8.999999999999992895 ) ) ;
#11399=CARTESIAN_POINT ( 'NONE',  ( -4.000000000000003553, -25.00000000000000000, 8.999999999999992895 ) ) ;
#11400=CARTESIAN_POINT ( 'NONE',  ( 0.000000000000000000, 0.000000000000000000, 17.00000000000000000 ) ) ;
#11408=CARTESIAN_POINT ( 'NONE',  ( -3.735045420075836212E-15, -28.06562499938548427, 4.662447845253954171 ) ) ;
#11417=CARTESIAN_POINT ( 'NONE',  ( 3.834746474454188013E-15, 28.20624999877096428, 4.999999999999992006 ) ) ;
#11418=CARTESIAN_POINT ( 'NONE',  ( 20.32269083260512588, 20.32269083260505838, 13.33755215474602984 ) ) ;
#11421=CARTESIAN_POINT ( 'NONE',  ( 4.000000000000001776, 26.76249999999999929, 11.30940107675849760 ) ) ;
#11422=ADVANCED_FACE ( 'NONE', ( #6079 ), #20195, .T. ) ;
#11423=CARTESIAN_POINT ( 'NONE',  ( 19.52719570377026059, 19.52719570377018599, 4.662447845253954171 ) ) ;
#11429=DIRECTION ( 'NONE',  ( -0.7071067811865487940, -0.7071067811865463515, 0.000000000000000000 ) ) ;
#11430=CIRCLE ( 'NONE', #13107, 30.00000000000000355 ) ;
#11434=CARTESIAN_POINT ( 'NONE',  ( 17.14423315256455282, 18.65998268041653674, 12.99999999999999467 ) ) ;
#11436=EDGE_LOOP ( 'NONE', ( #12363, #3175, #19180, #17179, #8807, #23029, #15493, #20795, #1888, #3050, #5910, #10875, #15906, #21730, #14415, #17806, #17480, #25659, #7507, #2366, #22647, #23196, #10010, #22106 ) ) ;
#11437=( BOUNDED_CURVE ( )  B_SPLINE_CURVE ( 2, ( #3658, #17534, #25508, #1185, #17672, #5504, #9306, #13225, #13494 ),
 .UNSPECIFIED., .F., .F. ) 
 B_SPLINE_CURVE_WITH_KNOTS ( ( 3, 2, 2, 2, 3 ),
 ( 0.2750000000000000222, 0.2833333333333333259, 0.2999999999999999889, 0.3166666666666666519, 0.3250000000000000111 ),
 .UNSPECIFIED. ) 
 CURVE ( )  GEOMETRIC_REPRESENTATION_ITEM ( )  RATIONAL_B_SPLINE_CURVE ( ( 0.9330127018922194093, 0.9330127018922196314, 1.000000000000000000, 0.8660254037844387076, 1.000000000000000000, 0.8660254037844387076, 1.000000000000000000, 0.9330127018922191873, 0.9330127018922194093 ) ) 
 REPRESENTATION_ITEM ( '' )  );
#11440=CARTESIAN_POINT ( 'NONE',  ( -3.999999999999995559, 25.63749999999999929, 6.690598923241487306 ) ) ;
#11449=EDGE_CURVE ( 'NONE', #13483, #25775, #2164, .T. ) ;
#11451=CARTESIAN_POINT ( 'NONE',  ( -1.878215178124995832, 27.54062499938548214, 5.746835883940462963 ) ) ;
#11453=CARTESIAN_POINT ( 'NONE',  ( 22.07057040778514789, 16.41371615829269359, 11.30940107675849760 ) ) ;
#11454=CARTESIAN_POINT ( 'NONE',  ( 18.54381157061901675, 21.20000894857831852, 5.746835883940462963 ) ) ;
#11458=CARTESIAN_POINT ( 'NONE',  ( 15.88988766691455368, 21.20228242283322828, 6.831223922626973533 ) ) ;
#11462=CARTESIAN_POINT ( 'NONE',  ( -1.878215178124995832, 26.75312499938548783, 5.746835883940462963 ) ) ;
#11463=CARTESIAN_POINT ( 'NONE',  ( -4.000000000000001776, -26.31250000000000000, 11.30940107675849760 ) ) ;
#11466=ADVANCED_FACE ( 'NONE', ( #3867 ), #19928, .F. ) ;
#11469=CARTESIAN_POINT ( 'NONE',  ( -13.02991752792604707, 22.56362157461192908, 20.00001199999999812 ) ) ;
#11470=CARTESIAN_POINT ( 'NONE',  ( 3.756430356249995661, -28.92812499938548143, 6.831223922626973533 ) ) ;
#11473=CARTESIAN_POINT ( 'NONE',  ( 18.84476222413640301, 23.34301068176857896, 11.43940974718624659 ) ) ;
#11482=CARTESIAN_POINT ( 'NONE',  ( 1.071796769724487675, 28.69240381056766509, 4.999999999999988454 ) ) ;
#11486=ORIENTED_EDGE ( 'NONE', *, *, #6278, .T. ) ;
#11487=CARTESIAN_POINT ( 'NONE',  ( -8.831537335106614961E-15, -27.53124999877097068, 12.99999999999999112 ) ) ;
#11488=CARTESIAN_POINT ( 'NONE',  ( -3.756430356250002323, -29.71562499938548640, 11.16877607737301226 ) ) ;
#11497=CARTESIAN_POINT ( 'NONE',  ( -2.000000000000000888, -26.27499999999999858, 12.46410161513774817 ) ) ;
#11503=ORIENTED_EDGE ( 'NONE', *, *, #2543, .F. ) ;
#11511=CARTESIAN_POINT ( 'NONE',  ( -3.756430356249995661, 27.69062499938548427, 6.831223922626973533 ) ) ;
#11518=CARTESIAN_POINT ( 'NONE',  ( -3.752267015613588906E-15, -26.85624999877096641, 4.381197846482986158 ) ) ;
#11521=EDGE_CURVE ( 'NONE', #8734, #15394, #13588, .T. ) ;
#11529=DIRECTION ( 'NONE',  ( -0.000000000000000000, -0.000000000000000000, 1.000000000000000000 ) ) ;
#11531=CARTESIAN_POINT ( 'NONE',  ( -2.672651547586948120E-15, -28.74062499938548498, 13.33755215474602984 ) ) ;
#11539=B_SPLINE_CURVE_WITH_KNOTS ( 'NONE', 3,
 ( #11607, #19581, #17643, #10285, #24032, #17890, #119, #11989, #15938, #23910, #22062, #13842, #22328, #14233, #25863, #9786, #7818, #6378 ),
 .UNSPECIFIED., .F., .F.,
 ( 4, 2, 2, 2, 2, 2, 2, 2, 4 ),
 ( 0.01878087663358380885, 0.01956282976579720376, 0.02034478289801060213, 0.02112673603022399704, 0.02190868916243739195, 0.02269064229465078686, 0.02347259542686418177, 0.02425454855907758014, 0.02503650169129097505 ),
 .UNSPECIFIED. ) ;
#11541=CARTESIAN_POINT ( 'NONE',  ( 23.03192121915348878, 17.71952646323466496, 11.16877607737301226 ) ) ;
#11542=DIRECTION ( 'NONE',  ( 0.000000000000000000, 0.000000000000000000, -1.000000000000000000 ) ) ;
#11544=CARTESIAN_POINT ( 'NONE',  ( 2.000000000000000888, 26.72500000000000142, 12.46410161513774817 ) ) ;
#11545=CARTESIAN_POINT ( 'NONE',  ( 22.10157009459123856, 19.44537271663178757, 5.746835883940462963 ) ) ;
#11546=CARTESIAN_POINT ( 'NONE',  ( -2.000000000000000888, -29.36874999877096926, 12.46410161513774817 ) ) ;
#11553=CARTESIAN_POINT ( 'NONE',  ( 15.03485793497900680, 20.69171218447132077, 11.30940107675849404 ) ) ;
#11563=EDGE_CURVE ( 'NONE', #9293, #20546, #18109, .T. ) ;
#11566=CARTESIAN_POINT ( 'NONE',  ( 1.878215178125000939, 27.76562499938548356, 12.25316411605952283 ) ) ;
#11571=CARTESIAN_POINT ( 'NONE',  ( 21.05410440982949183, 18.22567728508322205, 5.535898384862238508 ) ) ;
#11572=CARTESIAN_POINT ( 'NONE',  ( 16.65886629145492748, 21.97126104737360919, 11.16877607737301226 ) ) ;
#11576=CARTESIAN_POINT ( 'NONE',  ( 0.000000000000000000, 0.000000000000000000, 17.00000000000000000 ) ) ;
#11580=CARTESIAN_POINT ( 'NONE',  ( -2.000000000000000888, -27.17500000000000071, 12.46410161513774817 ) ) ;
#11588=VERTEX_POINT ( 'NONE', #7319 ) ;
#11599=CARTESIAN_POINT ( 'NONE',  ( 20.74032577480890183, 20.74032577480883077, 12.99999999999999289 ) ) ;
#11607=CARTESIAN_POINT ( 'NONE',  ( 4.000000000000003553, 29.73213749463701561, 8.999999999999992895 ) ) ;
#11609=CARTESIAN_POINT ( 'NONE',  ( 19.67524618651571799, 16.84681906176946242, 12.46410161513774817 ) ) ;
#11613=CARTESIAN_POINT ( 'NONE',  ( 3.137519842735244810E-15, -26.85624999877096641, 4.999999999999991118 ) ) ;
#11619=ORIENTED_EDGE ( 'NONE', *, *, #25079, .F. ) ;
#11626=EDGE_CURVE ( 'NONE', #20014, #256, #3389, .T. ) ;
#11632=CARTESIAN_POINT ( 'NONE',  ( -1.878215178124995832, 29.00312499938548427, 5.746835883940462963 ) ) ;
#11635=VECTOR ( 'NONE', #18795, 1000.000000000000000 ) ;
#11640=CARTESIAN_POINT ( 'NONE',  ( 3.999999999999995559, -25.58124999877096784, 6.690598923241487306 ) ) ;
#11642=CARTESIAN_POINT ( 'NONE',  ( -2.620986760973688460E-15, -27.53124999877097068, 13.61880215351699874 ) ) ;
#11643=CARTESIAN_POINT ( 'NONE',  ( -3.756430356249995661, 28.59062499938548640, 6.831223922626973533 ) ) ;
#11651=ORIENTED_EDGE ( 'NONE', *, *, #19707, .F. ) ;
#11654=CARTESIAN_POINT ( 'NONE',  ( -3.756430356250003655, -27.50312499938548427, 8.999999999999992895 ) ) ;
#11657=AXIS2_PLACEMENT_3D ( 'NONE', #20536, #14406, #2628 ) ;
#11658=EDGE_LOOP ( 'NONE', ( #2849, #8127, #8800, #8993 ) ) ;
#11659=( BOUNDED_CURVE ( )  B_SPLINE_CURVE ( 2, ( #4624, #9064, #12607, #22684, #709, #20582, #972, #19123, #8954 ),
 .UNSPECIFIED., .F., .F. ) 
 B_SPLINE_CURVE_WITH_KNOTS ( ( 3, 2, 2, 2, 3 ),
 ( 0.4250000000000000444, 0.4333333333333333481, 0.4500000000000000111, 0.4666666666666666741, 0.4750000000000000333 ),
 .UNSPECIFIED. ) 
 CURVE ( )  GEOMETRIC_REPRESENTATION_ITEM ( )  RATIONAL_B_SPLINE_CURVE ( ( 0.9330127018922194093, 0.9330127018922196314, 1.000000000000000000, 0.8660254037844387076, 1.000000000000000000, 0.8660254037844387076, 1.000000000000000000, 0.9330127018922191873, 0.9330127018922194093 ) ) 
 REPRESENTATION_ITEM ( '' )  );
#11667=CARTESIAN_POINT ( 'NONE',  ( 21.99550407741325486, 19.33930669945380743, 12.25316411605952283 ) ) ;
#11671=CARTESIAN_POINT ( 'NONE',  ( -1.999999999999998224, 27.10000000000000142, 12.46410161513774639 ) ) ;
#11672=EDGE_CURVE ( 'NONE', #17557, #8943, #8097, .T. ) ;
#11675=CARTESIAN_POINT ( 'NONE',  ( 17.61346044605677008, 22.92585520197543758, 11.16877607737301048 ) ) ;
#11677=ORIENTED_EDGE ( 'NONE', *, *, #8562, .F. ) ;
#11681=ORIENTED_EDGE ( 'NONE', *, *, #5656, .F. ) ;
#11682=CARTESIAN_POINT ( 'NONE',  ( 2.000000000000000888, 26.27499999999999858, 12.46410161513774817 ) ) ;
#11683=AXIS2_PLACEMENT_3D ( 'NONE', #15722, #11529, #23569 ) ;
#11687=EDGE_LOOP ( 'NONE', ( #18675, #23575, #20847 ) ) ;
#11690=ORIENTED_EDGE ( 'NONE', *, *, #5988, .F. ) ;
#11696=( BOUNDED_SURFACE ( )  B_SPLINE_SURFACE ( 1, 2, ( 
 ( #13123, #3051, #965, #6844, #16650, #2784, #5007, #6703, #4877, #7098, #14698, #17178, #6966, #22678, #22799, #9057, #12990, #4763, #12732, #10747, #825, #1084, #20970, #8947, #21093, #15215, #12852, #3171, #20826, #16922, #8803, #15083, #24762, #11138, #19116, #19000, #2914, #10878, #25009, #1205, #18877, #9188, #25146, #9709, #7478, #15468, #23686, #17555, #13376, #23302, #1598, #11795, #5650, #5388, #9828, #21350, #25660, #15847, #21599, #3678, #11654, #25392, #23819, #19631, #13630, #15724, #1736, #23436, #17813, #15333, #7860, #1475, #1867, #5524, #17691, #11408, #15599, #23572, #7741, #13513, #25778, #3434, #5906, #9447, #21213, #21483, #5768, #19381, #13752, #21731, #3556, #3292, #3815, #11531, #19771, #11264, #19251, #19499, #1349, #9326, #17311, #9567, #25275, #7615, #7357, #17427, #25531, #19883, #3949, #761, #10425, #20769, #16339, #520, #18423, #16721, #20641, #22341, #11915, #2459, #14499 ),
 ( #14383, #24308, #6514, #14765, #18676, #644, #24552, #6394, #6639, #22741, #8733, #8490, #4819, #4424, #2847, #24694, #14629, #12529, #16476, #24828, #12399, #16593, #1984, #24438, #6780, #9951, #10814, #10564, #8879, #22467, #2723, #8612, #21866, #16863, #13893, #17938, #12672, #22609, #20505, #12795, #896, #4547, #18808, #2604, #18561, #8003, #28, #20364, #4694, #10687, #13185, #18944, #10956, #5324, #21155, #12922, #9503, #19321, #21279, #19058, #1142, #9388, #3227, #24946, #9002, #11198, #23369, #17249, #16981, #21417, #7026, #11337, #1532, #7297, #15276, #23241, #11079, #17484, #13305, #25217, #1415, #15393, #19179, #1276, #3361, #15014, #17368, #25335, #9115, #25081, #2986, #23125, #6904, #7167, #22994, #1027, #7413, #4938, #5455, #13448, #3498, #11470, #19440, #14887, #22862, #9260, #20898, #5079, #13060, #21038, #3114, #17106, #15157, #5208, #7799, #21535, #13570, #3617, #18010, #12105, #11854 ) ),
 .UNSPECIFIED., .F., .F., .T. ) 
 B_SPLINE_SURFACE_WITH_KNOTS ( ( 2, 2 ),
 ( 3, 2, 2, 2, 2, 2, 2, 2, 2, 2, 2, 2, 2, 2, 2, 2, 2, 2, 2, 2, 2, 2, 2, 2, 2, 2, 2, 2, 2, 2, 2, 2, 2, 2, 2, 2, 2, 2, 2, 2, 2, 2, 2, 2, 2, 2, 2, 2, 2, 2, 2, 2, 2, 2, 2, 2, 2, 2, 2, 2, 3 ),
 ( 0.000000000000000000, 1.000000000000000000 ),
 ( 0.000000000000000000, 0.01666666666666666644, 0.03333333333333333287, 0.05000000000000000278, 0.06666666666666666574, 0.08333333333333332871, 0.1000000000000000056, 0.1166666666666666685, 0.1333333333333333315, 0.1499999999999999944, 0.1666666666666666574, 0.1833333333333333204, 0.2000000000000000111, 0.2166666666666666741, 0.2333333333333333370, 0.2500000000000000000, 0.2666666666666666630, 0.2833333333333333259, 0.2999999999999999889, 0.3166666666666666519, 0.3333333333333333148, 0.3499999999999999778, 0.3666666666666666408, 0.3833333333333333592, 0.4000000000000000222, 0.4166666666666666852, 0.4333333333333333481, 0.4500000000000000111, 0.4666666666666666741, 0.4833333333333333370, 0.5000000000000000000, 0.5166666666666667185, 0.5333333333333333259, 0.5500000000000000444, 0.5666666666666666519, 0.5833333333333333703, 0.5999999999999999778, 0.6166666666666666963, 0.6333333333333333037, 0.6500000000000000222, 0.6666666666666666297, 0.6833333333333333481, 0.6999999999999999556, 0.7166666666666666741, 0.7333333333333332815, 0.7500000000000000000, 0.7666666666666667185, 0.7833333333333333259, 0.8000000000000000444, 0.8166666666666666519, 0.8333333333333333703, 0.8499999999999999778, 0.8666666666666666963, 0.8833333333333333037, 0.9000000000000000222, 0.9166666666666666297, 0.9333333333333333481, 0.9499999999999999556, 0.9666666666666666741, 0.9833333333333332815, 1.000000000000000000 ),
 .UNSPECIFIED. ) 
 GEOMETRIC_REPRESENTATION_ITEM ( )  RATIONAL_B_SPLINE_SURFACE ( (
 ( 1.000000000000000000, 0.8660254037844387076, 1.000000000000000000, 0.8660254037844387076, 1.000000000000000000, 0.8660254037844387076, 1.000000000000000000, 0.8660254037844387076, 1.000000000000000000, 0.8660254037844387076, 1.000000000000000000, 0.8660254037844387076, 1.000000000000000000, 0.8660254037844387076, 1.000000000000000000, 0.8660254037844387076, 1.000000000000000000, 0.8660254037844387076, 1.000000000000000000, 0.8660254037844387076, 1.000000000000000000, 0.8660254037844387076, 1.000000000000000000, 0.8660254037844387076, 1.000000000000000000, 0.8660254037844387076, 1.000000000000000000, 0.8660254037844387076, 1.000000000000000000, 0.8660254037844387076, 1.000000000000000000, 0.8660254037844387076, 1.000000000000000000, 0.8660254037844387076, 1.000000000000000000, 0.8660254037844387076, 1.000000000000000000, 0.8660254037844387076, 1.000000000000000000, 0.8660254037844387076, 1.000000000000000000, 0.8660254037844387076, 1.000000000000000000, 0.8660254037844387076, 1.000000000000000000, 0.8660254037844387076, 1.000000000000000000, 0.8660254037844387076, 1.000000000000000000, 0.8660254037844387076, 1.000000000000000000, 0.8660254037844387076, 1.000000000000000000, 0.8660254037844387076, 1.000000000000000000, 0.8660254037844387076, 1.000000000000000000, 0.8660254037844387076, 1.000000000000000000, 0.8660254037844387076, 1.000000000000000000, 0.8660254037844387076, 1.000000000000000000, 0.8660254037844387076, 1.000000000000000000, 0.8660254037844387076, 1.000000000000000000, 0.8660254037844387076, 1.000000000000000000, 0.8660254037844387076, 1.000000000000000000, 0.8660254037844387076, 1.000000000000000000, 0.8660254037844387076, 1.000000000000000000, 0.8660254037844387076, 1.000000000000000000, 0.8660254037844387076, 1.000000000000000000, 0.8660254037844387076, 1.000000000000000000, 0.8660254037844387076, 1.000000000000000000, 0.8660254037844387076, 1.000000000000000000, 0.8660254037844387076, 1.000000000000000000, 0.8660254037844387076, 1.000000000000000000, 0.8660254037844387076, 1.000000000000000000, 0.8660254037844387076, 1.000000000000000000, 0.8660254037844387076, 1.000000000000000000, 0.8660254037844387076, 1.000000000000000000, 0.8660254037844387076, 1.000000000000000000, 0.8660254037844387076, 1.000000000000000000, 0.8660254037844387076, 1.000000000000000000, 0.8660254037844387076, 1.000000000000000000, 0.8660254037844387076, 1.000000000000000000, 0.8660254037844387076, 1.000000000000000000, 0.8660254037844387076, 1.000000000000000000, 0.8660254037844387076, 1.000000000000000000, 0.8660254037844387076, 1.000000000000000000, 0.8660254037844387076, 1.000000000000000000, 0.8660254037844387076, 1.000000000000000000, 0.8660254037844387076, 1.000000000000000000),
 ( 1.000000000000000000, 0.8660254037844387076, 1.000000000000000000, 0.8660254037844387076, 1.000000000000000000, 0.8660254037844387076, 1.000000000000000000, 0.8660254037844387076, 1.000000000000000000, 0.8660254037844387076, 1.000000000000000000, 0.8660254037844387076, 1.000000000000000000, 0.8660254037844387076, 1.000000000000000000, 0.8660254037844387076, 1.000000000000000000, 0.8660254037844387076, 1.000000000000000000, 0.8660254037844387076, 1.000000000000000000, 0.8660254037844387076, 1.000000000000000000, 0.8660254037844387076, 1.000000000000000000, 0.8660254037844387076, 1.000000000000000000, 0.8660254037844387076, 1.000000000000000000, 0.8660254037844387076, 1.000000000000000000, 0.8660254037844387076, 1.000000000000000000, 0.8660254037844387076, 1.000000000000000000, 0.8660254037844387076, 1.000000000000000000, 0.8660254037844387076, 1.000000000000000000, 0.8660254037844387076, 1.000000000000000000, 0.8660254037844387076, 1.000000000000000000, 0.8660254037844387076, 1.000000000000000000, 0.8660254037844387076, 1.000000000000000000, 0.8660254037844387076, 1.000000000000000000, 0.8660254037844387076, 1.000000000000000000, 0.8660254037844387076, 1.000000000000000000, 0.8660254037844387076, 1.000000000000000000, 0.8660254037844387076, 1.000000000000000000, 0.8660254037844387076, 1.000000000000000000, 0.8660254037844387076, 1.000000000000000000, 0.8660254037844387076, 1.000000000000000000, 0.8660254037844387076, 1.000000000000000000, 0.8660254037844387076, 1.000000000000000000, 0.8660254037844387076, 1.000000000000000000, 0.8660254037844387076, 1.000000000000000000, 0.8660254037844387076, 1.000000000000000000, 0.8660254037844387076, 1.000000000000000000, 0.8660254037844387076, 1.000000000000000000, 0.8660254037844387076, 1.000000000000000000, 0.8660254037844387076, 1.000000000000000000, 0.8660254037844387076, 1.000000000000000000, 0.8660254037844387076, 1.000000000000000000, 0.8660254037844387076, 1.000000000000000000, 0.8660254037844387076, 1.000000000000000000, 0.8660254037844387076, 1.000000000000000000, 0.8660254037844387076, 1.000000000000000000, 0.8660254037844387076, 1.000000000000000000, 0.8660254037844387076, 1.000000000000000000, 0.8660254037844387076, 1.000000000000000000, 0.8660254037844387076, 1.000000000000000000, 0.8660254037844387076, 1.000000000000000000, 0.8660254037844387076, 1.000000000000000000, 0.8660254037844387076, 1.000000000000000000, 0.8660254037844387076, 1.000000000000000000, 0.8660254037844387076, 1.000000000000000000, 0.8660254037844387076, 1.000000000000000000, 0.8660254037844387076, 1.000000000000000000, 0.8660254037844387076, 1.000000000000000000, 0.8660254037844387076, 1.000000000000000000, 0.8660254037844387076, 1.000000000000000000) ) ) 
 REPRESENTATION_ITEM ( '' )  SURFACE ( )  );
#11699=EDGE_CURVE ( 'NONE', #14590, #23126, #8942, .T. ) ;
#11701=ADVANCED_FACE ( 'NONE', ( #2453 ), #20358, .F. ) ;
#11705=FACE_OUTER_BOUND ( 'NONE', #3613, .T. ) ;
#11706=CARTESIAN_POINT ( 'NONE',  ( 18.55271417138207468, 18.55271417138200718, 13.61880215351699874 ) ) ;
#11707=CARTESIAN_POINT ( 'NONE',  ( 23.35011927068743276, 18.03772451476861605, 11.16877607737301226 ) ) ;
#11714=CARTESIAN_POINT ( 'NONE',  ( 19.52492222951535439, 22.18111960747465261, 12.25316411605951927 ) ) ;
#11718=CARTESIAN_POINT ( 'NONE',  ( -2.000000000000000888, -26.72500000000000142, 12.46410161513774817 ) ) ;
#11724=CARTESIAN_POINT ( 'NONE',  ( 6.741346781237198549, 25.16843286583315020, 20.00001200000000168 ) ) ;
#11728=( LENGTH_UNIT ( ) NAMED_UNIT ( * ) SI_UNIT ( .MILLI., .METRE. ) );
#11733=DIRECTION ( 'NONE',  ( -0.000000000000000000, 1.000000000000000000, 0.000000000000000000 ) ) ;
#11734=DIRECTION ( 'NONE',  ( -0.000000000000000000, -0.000000000000000000, -1.000000000000000000 ) ) ;
#11735=VECTOR ( 'NONE', #19924, 1000.000000000000000 ) ;
#11736=CARTESIAN_POINT ( 'NONE',  ( 19.19352969096333439, 22.02195681570944785, 5.535898384862237620 ) ) ;
#11738=CARTESIAN_POINT ( 'NONE',  ( -1.071796769724488563, 26.66740381056766651, 12.99999999999999289 ) ) ;
#11742=VERTEX_POINT ( 'NONE', #24160 ) ;
#11743=FACE_BOUND ( 'NONE', #7349, .T. ) ;
#11744=CARTESIAN_POINT ( 'NONE',  ( 3.756430356249997882, -29.56562499938549138, 11.16877607737301226 ) ) ;
#11747=ADVANCED_FACE ( 'NONE', ( #10171 ), #4298, .T. ) ;
#11749=VECTOR ( 'NONE', #24771, 1000.000000000000000 ) ;
#11751=CARTESIAN_POINT ( 'NONE',  ( 3.756430356250003655, 29.75312499938548783, 8.999999999999992895 ) ) ;
#11755=CARTESIAN_POINT ( 'NONE',  ( 1.071796769724485454, -26.61115380933863150, 12.99999999999999467 ) ) ;
#11771=CARTESIAN_POINT ( 'NONE',  ( 1.878215178125004048, 28.02812499938548640, 5.746835883940462963 ) ) ;
#11775=EDGE_CURVE ( 'NONE', #13481, #15567, #12601, .T. ) ;
#11777=AXIS2_PLACEMENT_3D ( 'NONE', #5806, #9360, #9742 ) ;
#11779=DIRECTION ( 'NONE',  ( 0.000000000000000000, -1.000000000000000000, 0.000000000000000000 ) ) ;
#11781=CARTESIAN_POINT ( 'NONE',  ( -4.000000000000003553, -27.68124999877096926, 6.690598923241489970 ) ) ;
#11782=VECTOR ( 'NONE', #22315, 1000.000000000000000 ) ;
#11783=CARTESIAN_POINT ( 'NONE',  ( 2.672651547586948120E-15, 27.84062499938548640, 13.33755215474602984 ) ) ;
#11784=ADVANCED_FACE ( 'NONE', ( #24300 ), #6386, .F. ) ;
#11795=CARTESIAN_POINT ( 'NONE',  ( -3.735045420075836212E-15, -27.16562499938548569, 4.662447845253954171 ) ) ;
#11800=ORIENTED_EDGE ( 'NONE', *, *, #22350, .F. ) ;
#11805=CARTESIAN_POINT ( 'NONE',  ( 15.25349156384666216, 20.56588631976534387, 6.831223922626973533 ) ) ;
#11808=CARTESIAN_POINT ( 'NONE',  ( 27.09999999999999787, -0.5999999999999998668, 19.59999999999999787 ) ) ;
#11810=CARTESIAN_POINT ( 'NONE',  ( 4.000000000000003553, 29.08750000000000213, 6.690598923241489970 ) ) ;
#11813=CARTESIAN_POINT ( 'NONE',  ( 23.35011927068743276, 18.03772451476861605, 11.16877607737301403 ) ) ;
#11822=DIRECTION ( 'NONE',  ( -0.7071067811865487940, -0.7071067811865463515, 0.000000000000000000 ) ) ;
#11823=CARTESIAN_POINT ( 'NONE',  ( 14.98182492639001673, 20.63867917588233070, 6.690598923241487306 ) ) ;
#11824=ORIENTED_EDGE ( 'NONE', *, *, #1130, .T. ) ;
#11834=CARTESIAN_POINT ( 'NONE',  ( -3.756430356249995661, 26.22812499938548214, 6.831223922626973533 ) ) ;
#11838=CARTESIAN_POINT ( 'NONE',  ( 22.73348301514753800, 17.07662876565508370, 8.999999999999992895 ) ) ;
#11839=CARTESIAN_POINT ( 'NONE',  ( 22.74023967191403628, 17.42784491599521601, 8.999999999999992895 ) ) ;
#11840=CARTESIAN_POINT ( 'NONE',  ( -4.000000000000003553, -28.58124999877096784, 6.690598923241489970 ) ) ;
#11841=DIRECTION ( 'NONE',  ( 0.000000000000000000, 0.000000000000000000, -1.000000000000000000 ) ) ;
#11844=CARTESIAN_POINT ( 'NONE',  ( 20.72043839702256207, 20.72043839702248036, 4.662447845253954171 ) ) ;
#11847=CARTESIAN_POINT ( 'NONE',  ( 1.999999999999995781, -26.05000000000000071, 5.535898384862237620 ) ) ;
#11848=CARTESIAN_POINT ( 'NONE',  ( 20.64868662990473069, 15.16406212719910052, 8.999999999999992895 ) ) ;
#11854=CARTESIAN_POINT ( 'NONE',  ( -3.756430356250003655, -29.64062499938548356, 8.999999999999992895 ) ) ;
#11855=VERTEX_POINT ( 'NONE', #2594 ) ;
#11865=CARTESIAN_POINT ( 'NONE',  ( -3.959305671612554781E-15, -25.00000000000000000, 12.99999999999999289 ) ) ;
#11868=CARTESIAN_POINT ( 'NONE',  ( 18.81908170618357090, 17.30333217833144843, 4.999999999999993783 ) ) ;
#11870=CARTESIAN_POINT ( 'NONE',  ( 15.57168961538060969, 20.88408437129928785, 6.831223922626973533 ) ) ;
#11871=CARTESIAN_POINT ( 'NONE',  ( 16.75401129586974491, 19.58243842061586548, 12.46410161513774639 ) ) ;
#11873=CARTESIAN_POINT ( 'NONE',  ( 3.469446951953614189E-15, 25.00000000000000000, 8.999999999999992895 ) ) ;
#11877=CARTESIAN_POINT ( 'NONE',  ( 3.469446951953614189E-15, 25.00000000000000000, 4.999999999999992006 ) ) ;
#11879=ORIENTED_EDGE ( 'NONE', *, *, #8610, .T. ) ;
#11883=ORIENTED_EDGE ( 'NONE', *, *, #4219, .F. ) ;
#11896=CARTESIAN_POINT ( 'NONE',  ( 3.756430356250004099, 27.09062499938548285, 6.831223922626973533 ) ) ;
#11901=CARTESIAN_POINT ( 'NONE',  ( 2.000000000000000888, 25.76874999877096784, 12.46410161513774817 ) ) ;
#11902=DIRECTION ( 'NONE',  ( 0.000000000000000000, 1.000000000000000000, 0.000000000000000000 ) ) ;
#11903=CARTESIAN_POINT ( 'NONE',  ( 1.999999999999998224, -29.74374999877096926, 12.46410161513774639 ) ) ;
#11904=CARTESIAN_POINT ( 'NONE',  ( -1.878215178124998497, 27.80312499938548498, 12.25316411605951927 ) ) ;
#11906=FACE_OUTER_BOUND ( 'NONE', #16104, .T. ) ;
#11915=CARTESIAN_POINT ( 'NONE',  ( -1.878215178125000939, -29.67812499938548498, 12.25316411605952283 ) ) ;
#11917=FACE_OUTER_BOUND ( 'NONE', #16509, .T. ) ;
#11920=CARTESIAN_POINT ( 'NONE',  ( -3.756430356249997438, 26.41562499938548569, 11.16877607737301048 ) ) ;
#11924=CARTESIAN_POINT ( 'NONE',  ( 22.31370212894720240, 19.65750475098775496, 12.25316411605952283 ) ) ;
#11928=CARTESIAN_POINT ( 'NONE',  ( 2.000000000000003997, 28.67500000000000426, 5.535898384862238508 ) ) ;
#11938=CARTESIAN_POINT ( 'NONE',  ( -1.999999999999995781, 29.59374999877096712, 5.535898384862237620 ) ) ;
#11941=VERTEX_POINT ( 'NONE', #2839 ) ;
#11944=CARTESIAN_POINT ( 'NONE',  ( -3.469446951953614189E-15, -30.00000000000000355, 8.999999999999992895 ) ) ;
#11949=CARTESIAN_POINT ( 'NONE',  ( 0.000000000000000000, 0.000000000000000000, 19.59999999999999787 ) ) ;
#11952=CARTESIAN_POINT ( 'NONE',  ( -1.878215178124995832, 26.64062499938548711, 5.746835883940462963 ) ) ;
#11955=DIRECTION ( 'NONE',  ( 0.000000000000000000, 0.000000000000000000, -1.000000000000000000 ) ) ;
#11957=CARTESIAN_POINT ( 'NONE',  ( 17.74838020778238246, 20.57680733252850303, 12.46410161513774639 ) ) ;
#11958=CARTESIAN_POINT ( 'NONE',  ( 20.95908693567302450, 20.95908693567294989, 13.33755215474602984 ) ) ;
#11961=CARTESIAN_POINT ( 'NONE',  ( 3.756430356249996994, -25.36562499938548498, 8.999999999999992895 ) ) ;
#11962=CARTESIAN_POINT ( 'NONE',  ( 23.29708626209844269, 17.98469150617961887, 8.999999999999992895 ) ) ;
#11965=CARTESIAN_POINT ( 'NONE',  ( -4.000000000000001776, -27.66249999999999787, 11.30940107675849760 ) ) ;
#11967=ORIENTED_EDGE ( 'NONE', *, *, #12980, .T. ) ;
#11974=CARTESIAN_POINT ( 'NONE',  ( -1.878215178125004048, -25.32812499938548356, 5.746835883940462963 ) ) ;
#11981=CARTESIAN_POINT ( 'NONE',  ( 20.74032577480890183, 20.74032577480883077, 12.99999999999999289 ) ) ;
#11983=CARTESIAN_POINT ( 'NONE',  ( 18.07541709408115693, 18.07541709408108588, 4.999999999999992006 ) ) ;
#11985=CARTESIAN_POINT ( 'NONE',  ( 16.55507374853184999, 19.21127112649115531, 5.746835883940462963 ) ) ;
#11986=CARTESIAN_POINT ( 'NONE',  ( 20.37793354945079471, 17.54950642470453204, 5.535898384862238508 ) ) ;
#11989=CARTESIAN_POINT ( 'NONE',  ( 3.182002658620821212, 29.83112730774910659, 6.562149109989046103 ) ) ;
#11991=CARTESIAN_POINT ( 'NONE',  ( -4.000096396247766251, 29.73212452601126188, 9.259737768674039415 ) ) ;
#11994=ORIENTED_EDGE ( 'NONE', *, *, #15864, .T. ) ;
#11995=CARTESIAN_POINT ( 'NONE',  ( 3.469446951953614189E-15, 30.00000000000000355, 8.999999999999992895 ) ) ;
#11996=CARTESIAN_POINT ( 'NONE',  ( -3.999999999999996447, 26.06874999877096855, 8.999999999999992895 ) ) ;
#12000=ORIENTED_EDGE ( 'NONE', *, *, #25820, .T. ) ;
#12011=CARTESIAN_POINT ( 'NONE',  ( -1.878215178124998497, 29.60312499938548569, 12.25316411605951927 ) ) ;
#12016=CARTESIAN_POINT ( 'NONE',  ( -3.469446951953614189E-15, -30.00000000000000355, 8.999999999999992895 ) ) ;
#12019=EDGE_CURVE ( 'NONE', #18087, #19408, #16953, .T. ) ;
#12020=CARTESIAN_POINT ( 'NONE',  ( -2.620986760973688460E-15, -29.33124999877096784, 13.61880215351699874 ) ) ;
#12021=CARTESIAN_POINT ( 'NONE',  ( 3.756430356250004099, 28.44062499938548783, 6.831223922626973533 ) ) ;
#12024=CARTESIAN_POINT ( 'NONE',  ( 17.67766952966372429, 17.67766952966365679, 8.999999999999992895 ) ) ;
#12032=CARTESIAN_POINT ( 'NONE',  ( 17.28434138175965273, 20.11276850650576975, 5.535898384862237620 ) ) ;
#12039=VERTEX_POINT ( 'NONE', #7158 ) ;
#12041=CARTESIAN_POINT ( 'NONE',  ( 3.756430356250003655, 25.70312499938548356, 8.999999999999992895 ) ) ;
#12046=CARTESIAN_POINT ( 'NONE',  ( 21.38789795289476103, 16.07550319697594432, 8.999999999999992895 ) ) ;
#12049=VECTOR ( 'NONE', #25345, 1000.000000000000000 ) ;
#12051=CARTESIAN_POINT ( 'NONE',  ( -3.999999999999996447, 28.82499999999999929, 8.999999999999992895 ) ) ;
#12052=CARTESIAN_POINT ( 'NONE',  ( -1.878215178124995832, 29.34062499938548285, 5.746835883940462963 ) ) ;
#12054=CARTESIAN_POINT ( 'NONE',  ( 20.16359180683815921, 20.16359180683808106, 4.662447845253954171 ) ) ;
#12060=EDGE_CURVE ( 'NONE', #13988, #3291, #9979, .T. ) ;
#12063=CARTESIAN_POINT ( 'NONE',  ( 2.000000000000003997, 26.42500000000000071, 5.535898384862238508 ) ) ;
#12064=CARTESIAN_POINT ( 'NONE',  ( -1.878215178124995832, 25.40312499938548640, 5.746835883940462963 ) ) ;
#12069=EDGE_CURVE ( 'NONE', #21212, #3297, #10436, .T. ) ;
#12084=CARTESIAN_POINT ( 'NONE',  ( 3.756430356250002323, 26.00312499938548427, 11.16877607737301226 ) ) ;
#12086=CARTESIAN_POINT ( 'NONE',  ( 1.071796769724487230, -28.67634618820330417, 4.999999999999992006 ) ) ;
#12092=FACE_OUTER_BOUND ( 'NONE', #12531, .T. ) ;
#12094=EDGE_CURVE ( 'NONE', #18284, #13049, #13783, .T. ) ;
#12095=CARTESIAN_POINT ( 'NONE',  ( 23.32360276639294128, 18.01120801047411391, 6.831223922626973533 ) ) ;
#12097=EDGE_LOOP ( 'NONE', ( #9262, #25460 ) ) ;
#12099=CARTESIAN_POINT ( 'NONE',  ( 1.999999999999995781, -29.19999999999999929, 5.535898384862237620 ) ) ;
#12105=CARTESIAN_POINT ( 'NONE',  ( -3.756430356250002323, -29.60312499938548569, 11.16877607737301226 ) ) ;
#12106=ORIENTED_EDGE ( 'NONE', *, *, #25028, .F. ) ;
#12108=CARTESIAN_POINT ( 'NONE',  ( -1.878215178125000939, -25.62812499938548783, 12.25316411605952283 ) ) ;
#12110=CARTESIAN_POINT ( 'NONE',  ( 22.03079565047434585, 16.37394140098189865, 11.30940107675849760 ) ) ;
#12111=VECTOR ( 'NONE', #4663, 1000.000000000000000 ) ;
#12119=AXIS2_PLACEMENT_3D ( 'NONE', #21648, #3488, #13561 ) ;
#12124=CARTESIAN_POINT ( 'NONE',  ( 22.66719175354224092, 17.01033750404978306, 11.30940107675849760 ) ) ;
#12134=CARTESIAN_POINT ( 'NONE',  ( 4.000000000000003553, 26.33124999877097139, 6.690598923241489970 ) ) ;
#12135=CARTESIAN_POINT ( 'NONE',  ( -3.735045420075836212E-15, -25.25312499938548783, 4.662447845253954171 ) ) ;
#12139=ORIENTED_EDGE ( 'NONE', *, *, #9299, .T. ) ;
#12154=CARTESIAN_POINT ( 'NONE',  ( 3.735045420075836212E-15, 26.60312499938547859, 4.662447845253954171 ) ) ;
#12160=CARTESIAN_POINT ( 'NONE',  ( -3.756430356250004099, -25.29062499938548569, 6.831223922626973533 ) ) ;
#12162=CARTESIAN_POINT ( 'NONE',  ( 3.756430356250003655, 29.75312499938548783, 8.999999999999992895 ) ) ;
#12165=CARTESIAN_POINT ( 'NONE',  ( 23.65505907007413811, 18.34266431415531073, 8.999999999999992895 ) ) ;
#12167=CARTESIAN_POINT ( 'NONE',  ( 4.000000000000003553, 25.43124999877097281, 6.690598923241489970 ) ) ;
#12170=VECTOR ( 'NONE', #14741, 1000.000000000000000 ) ;
#12179=ORIENTED_EDGE ( 'NONE', *, *, #8568, .T. ) ;
#12180=ADVANCED_FACE ( 'NONE', ( #7215 ), #5368, .F. ) ;
#12182=CARTESIAN_POINT ( 'NONE',  ( 3.735045420075836212E-15, 26.26562499938548356, 4.662447845253954171 ) ) ;
#12187=CARTESIAN_POINT ( 'NONE',  ( 19.60674521665374215, 19.60674521665367820, 13.33755215474602984 ) ) ;
#12188=EDGE_CURVE ( 'NONE', #14283, #17328, #8619, .T. ) ;
#12189=AXIS2_PLACEMENT_3D ( 'NONE', #11218, #23646, #19339 ) ;
#12197=LINE ( 'NONE', #10486, #10931 ) ;
#12198=CARTESIAN_POINT ( 'NONE',  ( 2.000000000000000888, 27.56874999877096855, 12.46410161513774817 ) ) ;
#12205=ORIENTED_EDGE ( 'NONE', *, *, #6465, .T. ) ;
#12209=VERTEX_POINT ( 'NONE', #13358 ) ;
#12214=DIRECTION ( 'NONE',  ( -0.7071067811865487940, -0.7071067811865463515, 0.000000000000000000 ) ) ;
#12218=CARTESIAN_POINT ( 'NONE',  ( 1.071796769724492338, 26.70759618943233704, 12.99999999999999467 ) ) ;
#12221=EDGE_CURVE ( 'NONE', #1657, #25409, #23284, .T. ) ;
#12222=EDGE_CURVE ( 'NONE', #3647, #20357, #3428, .T. ) ;
#12223=CARTESIAN_POINT ( 'NONE',  ( -3.756430356249997882, 25.40312499938548285, 11.16877607737301226 ) ) ;
#12229=CARTESIAN_POINT ( 'NONE',  ( 21.54465973840859760, 18.71623261366233848, 12.46410161513774817 ) ) ;
#12230=CARTESIAN_POINT ( 'NONE',  ( -2.672651547586948120E-15, -25.92812499938548498, 13.33755215474603162 ) ) ;
#12243=CARTESIAN_POINT ( 'NONE',  ( -3.756430356250003211, -26.19062499938548783, 6.831223922626973533 ) ) ;
#12258=CARTESIAN_POINT ( 'NONE',  ( 18.81125008781888042, 18.81125008781880581, 4.662447845253954171 ) ) ;
#12259=CARTESIAN_POINT ( 'NONE',  ( 23.01190630937068349, 17.35505205987822919, 8.999999999999992895 ) ) ;
#12267=LINE ( 'NONE', #2212, #24245 ) ;
#12268=ORIENTED_EDGE ( 'NONE', *, *, #24499, .F. ) ;
#12270=CARTESIAN_POINT ( 'NONE',  ( 2.000000000000000888, 25.76874999877096784, 12.46410161513774817 ) ) ;
#12271=CARTESIAN_POINT ( 'NONE',  ( -1.878215178125000939, -26.41562499938548214, 12.25316411605952283 ) ) ;
#12278=ORIENTED_EDGE ( 'NONE', *, *, #21544, .T. ) ;
#12280=( BOUNDED_CURVE ( )  B_SPLINE_CURVE ( 2, ( #6113, #18277, #20229, #8335, #365, #14096, #22061, #4148, #9903 ),
 .UNSPECIFIED., .F., .F. ) 
 B_SPLINE_CURVE_WITH_KNOTS ( ( 3, 2, 2, 2, 3 ),
 ( 0.4250000000000000444, 0.4333333333333333481, 0.4500000000000000111, 0.4666666666666666741, 0.4750000000000000333 ),
 .UNSPECIFIED. ) 
 CURVE ( )  GEOMETRIC_REPRESENTATION_ITEM ( )  RATIONAL_B_SPLINE_CURVE ( ( 0.9330127018922194093, 0.9330127018922196314, 1.000000000000000000, 0.8660254037844387076, 1.000000000000000000, 0.8660254037844387076, 1.000000000000000000, 0.9330127018922191873, 0.9330127018922194093 ) ) 
 REPRESENTATION_ITEM ( '' )  );
#12284=( BOUNDED_CURVE ( )  B_SPLINE_CURVE ( 2, ( #25624, #15948, #21690, #3776, #17393, #25490, #23778, #11755, #25743 ),
 .UNSPECIFIED., .F., .F. ) 
 B_SPLINE_CURVE_WITH_KNOTS ( ( 3, 2, 2, 2, 3 ),
 ( 0.2250000000000000056, 0.2333333333333333370, 0.2500000000000000000, 0.2666666666666666630, 0.2750000000000000222 ),
 .UNSPECIFIED. ) 
 CURVE ( )  GEOMETRIC_REPRESENTATION_ITEM ( )  RATIONAL_B_SPLINE_CURVE ( ( 0.9330127018922194093, 0.9330127018922194093, 1.000000000000000000, 0.8660254037844387076, 1.000000000000000000, 0.8660254037844387076, 1.000000000000000000, 0.9330127018922191873, 0.9330127018922194093 ) ) 
 REPRESENTATION_ITEM ( '' )  );
#12287=CARTESIAN_POINT ( 'NONE',  ( 1.878215178125004048, 27.01562499938548711, 5.746835883940462963 ) ) ;
#12294=CARTESIAN_POINT ( 'NONE',  ( -1.878215178125000939, -25.62812499938548783, 12.25316411605952283 ) ) ;
#12299=DIRECTION ( 'NONE',  ( 0.7071067811865463515, -0.7071067811865487940, 0.000000000000000000 ) ) ;
#12301=CYLINDRICAL_SURFACE ( 'NONE', #22126, 4.000000000000000000 ) ;
#12307=ORIENTED_EDGE ( 'NONE', *, *, #10752, .T. ) ;
#12309=ORIENTED_EDGE ( 'NONE', *, *, #10863, .F. ) ;
#12313=CARTESIAN_POINT ( 'NONE',  ( -3.756430356249997438, 27.31562499938548427, 11.16877607737301048 ) ) ;
#12316=CARTESIAN_POINT ( 'NONE',  ( 16.52628376998245230, 21.83867852590112690, 6.831223922626973533 ) ) ;
#12323=CARTESIAN_POINT ( 'NONE',  ( 3.756430356250003211, 29.22812499938548569, 6.831223922626973533 ) ) ;
#12330=ORIENTED_EDGE ( 'NONE', *, *, #9035, .F. ) ;
#12335=CARTESIAN_POINT ( 'NONE',  ( 20.05973549791684718, 17.23130837317058806, 5.535898384862238508 ) ) ;
#12342=DIRECTION ( 'NONE',  ( 0.000000000000000000, 1.000000000000000000, 0.000000000000000000 ) ) ;
#12347=EDGE_CURVE ( 'NONE', #21476, #8528, #2353, .T. ) ;
#12350=CARTESIAN_POINT ( 'NONE',  ( 2.672651547586948120E-15, 27.72812499938548569, 13.33755215474602984 ) ) ;
#12355=DIRECTION ( 'NONE',  ( 0.000000000000000000, 0.000000000000000000, -1.000000000000000000 ) ) ;
#12356=CARTESIAN_POINT ( 'NONE',  ( 1.878215178124995832, -25.29062499938548569, 5.746835883940462963 ) ) ;
#12360=CARTESIAN_POINT ( 'NONE',  ( 3.999999999999997335, -28.41249999999999787, 11.30940107675849404 ) ) ;
#12363=ORIENTED_EDGE ( 'NONE', *, *, #8016, .F. ) ;
#12371=CARTESIAN_POINT ( 'NONE',  ( -3.756430356250003655, -27.50312499938548427, 8.999999999999992895 ) ) ;
#12380=FACE_OUTER_BOUND ( 'NONE', #25274, .T. ) ;
#12381=CARTESIAN_POINT ( 'NONE',  ( 16.84448182151639628, 22.15687657743507089, 6.831223922626973533 ) ) ;
#12382=CARTESIAN_POINT ( 'NONE',  ( 21.65072575558658130, 18.82229863084031507, 5.535898384862238508 ) ) ;
#12386=CARTESIAN_POINT ( 'NONE',  ( -0.5247320085691752345, 29.99650235037416834, 5.025996973432255821 ) ) ;
#12388=CARTESIAN_POINT ( 'NONE',  ( 15.59820611967510295, 20.91060087559377934, 8.999999999999992895 ) ) ;
#12393=CARTESIAN_POINT ( 'NONE',  ( 1.878215178124998497, -26.34062499938548285, 12.25316411605951927 ) ) ;
#12398=ORIENTED_EDGE ( 'NONE', *, *, #19243, .F. ) ;
#12399=CARTESIAN_POINT ( 'NONE',  ( 1.878215178124998497, -25.89062499938548356, 12.25316411605951927 ) ) ;
#12401=ORIENTED_EDGE ( 'NONE', *, *, #9329, .T. ) ;
#12404=CARTESIAN_POINT ( 'NONE',  ( 3.834746474454188013E-15, 27.81249999999999645, 4.999999999999992006 ) ) ;
#12407=CARTESIAN_POINT ( 'NONE',  ( 3.756430356250003655, 26.94062499938548427, 8.999999999999992895 ) ) ;
#12408=CARTESIAN_POINT ( 'NONE',  ( 20.62100150635272300, 20.62100150635266260, 4.999999999999992006 ) ) ;
#12414=CARTESIAN_POINT ( 'NONE',  ( -4.000000000000003553, -28.58124999877096784, 6.690598923241489970 ) ) ;
#12418=CARTESIAN_POINT ( 'NONE',  ( 1.036406108997123487, -29.98318460927812268, 5.127803451112008304 ) ) ;
#12426=EDGE_LOOP ( 'NONE', ( #19934, #16133, #12599, #697, #2391, #17096, #6845, #17575, #16197, #20822, #5675, #10882, #18906, #1600, #16196, #13404, #15691, #17578, #17140, #589, #19351, #16467, #6068, #19722, #1312 ) ) ;
#12430=CARTESIAN_POINT ( 'NONE',  ( -4.000000000000001776, -27.66249999999999787, 11.30940107675849760 ) ) ;
#12434=CARTESIAN_POINT ( 'NONE',  ( 1.878215178125004048, 25.77812499938548640, 5.746835883940462963 ) ) ;
#12437=DIRECTION ( 'NONE',  ( 1.000000000000000000, 0.000000000000000000, -0.000000000000000000 ) ) ;
#12438=CARTESIAN_POINT ( 'NONE',  ( 21.70609600442870857, 16.39370124850988830, 8.999999999999992895 ) ) ;
#12445=CARTESIAN_POINT ( 'NONE',  ( -3.756430356249996105, 28.92812499938548498, 6.831223922626973533 ) ) ;
#12447=CARTESIAN_POINT ( 'NONE',  ( -3.959305671612554781E-15, -30.00000000000000355, 12.99999999999999289 ) ) ;
#12450=ORIENTED_EDGE ( 'NONE', *, *, #16872, .F. ) ;
#12452=ORIENTED_EDGE ( 'NONE', *, *, #8826, .F. ) ;
#12454=ORIENTED_EDGE ( 'NONE', *, *, #4105, .T. ) ;
#12457=CARTESIAN_POINT ( 'NONE',  ( 3.999999999999997335, -29.70624999877096784, 11.30940107675849404 ) ) ;
#12460=EDGE_CURVE ( 'NONE', #20546, #7614, #1450, .T. ) ;
#12462=DIRECTION ( 'NONE',  ( 0.000000000000000000, 0.000000000000000000, -1.000000000000000000 ) ) ;
#12465=VECTOR ( 'NONE', #5514, 1000.000000000000000 ) ;
#12468=EDGE_CURVE ( 'NONE', #17328, #1348, #5119, .T. ) ;
#12469=CARTESIAN_POINT ( 'NONE',  ( -3.756430356249997882, 28.10312499938548569, 11.16877607737301226 ) ) ;
#12475=DIRECTION ( 'NONE',  ( 1.000000000000000000, 0.000000000000000000, 0.000000000000000000 ) ) ;
#12477=CARTESIAN_POINT ( 'NONE',  ( -1.878215178125004048, -25.66562499938548569, 5.746835883940462963 ) ) ;
#12478=LINE ( 'NONE', #22172, #7078 ) ;
#12483=CARTESIAN_POINT ( 'NONE',  ( 1.999999999999998224, -28.44999999999999929, 12.46410161513774639 ) ) ;
#12486=EDGE_LOOP ( 'NONE', ( #20937, #20427, #18970, #20672 ) ) ;
#12488=DIRECTION ( 'NONE',  ( 0.000000000000000000, 0.000000000000000000, -1.000000000000000000 ) ) ;
#12492=CARTESIAN_POINT ( 'NONE',  ( -3.756430356250003655, -25.70312499938548356, 8.999999999999992895 ) ) ;
#12500=AXIS2_PLACEMENT_3D ( 'NONE', #24783, #13401, #25176 ) ;
#12501=CYLINDRICAL_SURFACE ( 'NONE', #7934, 4.000000000000000000 ) ;
#12509=CARTESIAN_POINT ( 'NONE',  ( 21.38789795289476103, 16.07550319697594432, 8.999999999999992895 ) ) ;
#12510=CARTESIAN_POINT ( 'NONE',  ( 22.37551020630278842, 16.71865595681033412, 8.999999999999992895 ) ) ;
#12511=CARTESIAN_POINT ( 'NONE',  ( 1.859271017917182139E-15, 28.48749999999999716, 12.99999999999999289 ) ) ;
#12514=CARTESIAN_POINT ( 'NONE',  ( -2.439210544738880326, 29.90146712018378494, 5.819033386899011617 ) ) ;
#12515=VERTEX_POINT ( 'NONE', #653 ) ;
#12518=CARTESIAN_POINT ( 'NONE',  ( 21.80540536484019043, 16.14855111534773968, 6.690598923241489970 ) ) ;
#12519=ORIENTED_EDGE ( 'NONE', *, *, #13214, .F. ) ;
#12521=CARTESIAN_POINT ( 'NONE',  ( -3.999999999999996003, 25.58124999877097139, 6.690598923241487306 ) ) ;
#12522=CARTESIAN_POINT ( 'NONE',  ( 3.756430356249996994, -25.36562499938548498, 8.999999999999992895 ) ) ;
#12523=CARTESIAN_POINT ( 'NONE',  ( 15.64473753375240506, 21.30159178324472080, 8.999999999999992895 ) ) ;
#12529=CARTESIAN_POINT ( 'NONE',  ( 3.756430356249995661, -25.77812499938548640, 6.831223922626973533 ) ) ;
#12530=ORIENTED_EDGE ( 'NONE', *, *, #10475, .F. ) ;
#12531=EDGE_LOOP ( 'NONE', ( #5678, #9075, #17390, #18523 ) ) ;
#12536=CARTESIAN_POINT ( 'NONE',  ( -3.063240906311874401, -29.84319947910909931, 11.57226653943513028 ) ) ;
#12538=AXIS2_PLACEMENT_3D ( 'NONE', #25446, #21790, #7668 ) ;
#12541=CARTESIAN_POINT ( 'NONE',  ( 22.93879470346832150, 19.24746537414215908, 12.11182326528050623 ) ) ;
#12542=CARTESIAN_POINT ( 'NONE',  ( 1.878215178125004048, 25.21562499938548285, 5.746835883940462963 ) ) ;
#12546=CARTESIAN_POINT ( 'NONE',  ( 16.85123847828290167, 22.50809272777520675, 6.690598923241487306 ) ) ;
#12548=CARTESIAN_POINT ( 'NONE',  ( 17.33175248197874652, 18.84750200983072332, 4.999999999999991118 ) ) ;
#12549=CARTESIAN_POINT ( 'NONE',  ( 3.756430356249996994, -26.37812499938548783, 8.999999999999992895 ) ) ;
#12553=CARTESIAN_POINT ( 'NONE',  ( 3.013274039476890653, -29.84885987243285399, 6.356496494711869616 ) ) ;
#12566=DIRECTION ( 'NONE',  ( 0.000000000000000000, -1.000000000000000000, 0.000000000000000000 ) ) ;
#12570=CARTESIAN_POINT ( 'NONE',  ( -3.756430356249996105, 28.14062499938548356, 6.831223922626973533 ) ) ;
#12571=EDGE_CURVE ( 'NONE', #21735, #20241, #16734, .T. ) ;
#12574=CARTESIAN_POINT ( 'NONE',  ( 17.93393197184562027, 20.59012934980492560, 12.25316411605951927 ) ) ;
#12575=AXIS2_PLACEMENT_3D ( 'NONE', #7400, #15142, #7664 ) ;
#12576=CARTESIAN_POINT ( 'NONE',  ( 19.55913884271638281, 21.07488837056833830, 4.999999999999987566 ) ) ;
#12579=LINE ( 'NONE', #16775, #8363 ) ;
#12592=( BOUNDED_CURVE ( )  B_SPLINE_CURVE ( 2, ( #14090, #1935, #10277, #5717, #18157, #234, #9779, #24287, #24670 ),
 .UNSPECIFIED., .F., .F. ) 
 B_SPLINE_CURVE_WITH_KNOTS ( ( 3, 2, 2, 2, 3 ),
 ( 0.4750000000000000333, 0.4833333333333333370, 0.5000000000000000000, 0.5166666666666667185, 0.5250000000000000222 ),
 .UNSPECIFIED. ) 
 CURVE ( )  GEOMETRIC_REPRESENTATION_ITEM ( )  RATIONAL_B_SPLINE_CURVE ( ( 0.9330127018922194093, 0.9330127018922196314, 1.000000000000000000, 0.8660254037844387076, 1.000000000000000000, 0.8660254037844387076, 1.000000000000000000, 0.9330127018922194093, 0.9330127018922194093 ) ) 
 REPRESENTATION_ITEM ( '' )  );
#12593=EDGE_CURVE ( 'NONE', #17199, #21622, #4826, .T. ) ;
#12594=VECTOR ( 'NONE', #5704, 1000.000000000000000 ) ;
#12595=ORIENTED_EDGE ( 'NONE', *, *, #25631, .T. ) ;
#12598=CARTESIAN_POINT ( 'NONE',  ( -1.071796769724485454, 26.21740381056766367, 12.99999999999999467 ) ) ;
#12599=ORIENTED_EDGE ( 'NONE', *, *, #17756, .T. ) ;
#12600=CARTESIAN_POINT ( 'NONE',  ( 23.94977458897859890, 18.29292033948614105, 10.45670610619353980 ) ) ;
#12601=CIRCLE ( 'NONE', #5486, 30.00000000000000355 ) ;
#12604=VERTEX_POINT ( 'NONE', #8502 ) ;
#12607=CARTESIAN_POINT ( 'NONE',  ( 17.64231419060439876, 20.47074131535051933, 5.535898384862237620 ) ) ;
#12611=CARTESIAN_POINT ( 'NONE',  ( 15.33304107673014727, 20.64543583264882542, 6.831223922626973533 ) ) ;
#12613=CARTESIAN_POINT ( 'NONE',  ( 3.756430356250002323, 28.70312499938548356, 11.16877607737301226 ) ) ;
#12617=CARTESIAN_POINT ( 'NONE',  ( 16.63462326141533865, 19.29082063937464397, 5.746835883940462963 ) ) ;
#12619=CARTESIAN_POINT ( 'NONE',  ( 23.07819757097597702, 17.42134332148352627, 6.690598923241489970 ) ) ;
#12623=AXIS2_PLACEMENT_3D ( 'NONE', #4921, #22450, #10669 ) ;
#12624=CARTESIAN_POINT ( 'NONE',  ( 3.756430356249996994, -27.61562499938548143, 8.999999999999992895 ) ) ;
#12629=CARTESIAN_POINT ( 'NONE',  ( -2.000000000000000888, -29.42500000000000071, 12.46410161513774817 ) ) ;
#12632=ORIENTED_EDGE ( 'NONE', *, *, #4746, .F. ) ;
#12633=LINE ( 'NONE', #18645, #2464 ) ;
#12637=CARTESIAN_POINT ( 'NONE',  ( -1.878215178125000939, -26.52812499938548285, 12.25316411605952283 ) ) ;
#12639=CARTESIAN_POINT ( 'NONE',  ( 2.000000000000003997, 28.16874999877096997, 5.535898384862238508 ) ) ;
#12640=AXIS2_PLACEMENT_3D ( 'NONE', #20819, #18726, #6695 ) ;
#12646=DIRECTION ( 'NONE',  ( -0.2588190451025209615, 0.9659258262890682012, 0.000000000000000000 ) ) ;
#12648=EDGE_CURVE ( 'NONE', #8071, #18519, #11211, .T. ) ;
#12650=CARTESIAN_POINT ( 'NONE',  ( 20.37793354945079471, 17.54950642470453204, 5.535898384862238508 ) ) ;
#12651=CARTESIAN_POINT ( 'NONE',  ( 18.33395301051795911, 18.33395301051789161, 13.33755215474602984 ) ) ;
#12652=CARTESIAN_POINT ( 'NONE',  ( 15.67775563255858984, 20.99015038847727155, 8.999999999999992895 ) ) ;
#12659=EDGE_CURVE ( 'NONE', #2116, #12039, #23135, .T. ) ;
#12660=CARTESIAN_POINT ( 'NONE',  ( 19.37037015225818948, 16.71417277429875625, 12.25316411605952283 ) ) ;
#12661=CARTESIAN_POINT ( 'NONE',  ( 1.999999999999995781, -27.85000000000000142, 5.535898384862237620 ) ) ;
#12664=CARTESIAN_POINT ( 'NONE',  ( 4.000000000000003553, 28.54374999877096997, 8.999999999999992895 ) ) ;
#12665=CARTESIAN_POINT ( 'NONE',  ( 3.756430356249996994, -27.61562499938548143, 8.999999999999992895 ) ) ;
#12666=FACE_OUTER_BOUND ( 'NONE', #10081, .T. ) ;
#12668=EDGE_CURVE ( 'NONE', #23953, #23031, #4945, .T. ) ;
#12672=CARTESIAN_POINT ( 'NONE',  ( -3.756430356250003655, -26.49062499938548498, 8.999999999999992895 ) ) ;
#12674=EDGE_CURVE ( 'NONE', #7614, #4649, #2284, .T. ) ;
#12676=CARTESIAN_POINT ( 'NONE',  ( -3.137519842735244810E-15, 26.91249999999999787, 4.999999999999991118 ) ) ;
#12677=CYLINDRICAL_SURFACE ( 'NONE', #104, 4.000000000000000000 ) ;
#12678=CARTESIAN_POINT ( 'NONE',  ( 1.626862140677534194E-14, 27.58750000000000213, 12.99999999999999289 ) ) ;
#12683=CARTESIAN_POINT ( 'NONE',  ( 3.735045420075836212E-15, 28.85312499938548569, 4.662447845253954171 ) ) ;
#12685=CARTESIAN_POINT ( 'NONE',  ( 21.21320343559646915, 21.21320343559638744, 4.999999999999992006 ) ) ;
#12686=STYLED_ITEM ( 'NONE', ( #9426 ), #14134 ) ;
#12689=CARTESIAN_POINT ( 'NONE',  ( 18.39361514561510091, 18.39361514561503341, 4.999999999999992006 ) ) ;
#12690=CARTESIAN_POINT ( 'NONE',  ( -3.756430356250002323, -26.11562499938548498, 11.16877607737301226 ) ) ;
#12691=CARTESIAN_POINT ( 'NONE',  ( 3.756430356250003655, 29.30312499938548498, 8.999999999999992895 ) ) ;
#12695=CARTESIAN_POINT ( 'NONE',  ( 3.796077574538131660, -29.75903253174124430, 10.28786097927510923 ) ) ;
#12703=ORIENTED_EDGE ( 'NONE', *, *, #9244, .T. ) ;
#12712=CARTESIAN_POINT ( 'NONE',  ( 1.878215178125004048, 28.02812499938548640, 5.746835883940462963 ) ) ;
#12715=CARTESIAN_POINT ( 'NONE',  ( 20.24314131972164432, 20.24314131972156972, 13.33755215474602984 ) ) ;
#12717=CARTESIAN_POINT ( 'NONE',  ( -13.02991752792603997, -22.56362157461194684, 20.00001200000000168 ) ) ;
#12726=VERTEX_POINT ( 'NONE', #19452 ) ;
#12730=FACE_OUTER_BOUND ( 'NONE', #17486, .T. ) ;
#12732=CARTESIAN_POINT ( 'NONE',  ( 3.756430356249996994, -25.92812499938548498, 8.999999999999992895 ) ) ;
#12736=ADVANCED_FACE ( 'NONE', ( #5600 ), #19069, .F. ) ;
#12744=CARTESIAN_POINT ( 'NONE',  ( 19.87418373385361292, 17.21798635589416548, 5.746835883940462963 ) ) ;
#12745=CARTESIAN_POINT ( 'NONE',  ( -3.756430356249995661, 28.92812499938548143, 6.831223922626973533 ) ) ;
#12746=( BOUNDED_CURVE ( )  B_SPLINE_CURVE ( 2, ( #10699, #10969, #20655, #18954, #4830, #24449, #6527, #12806, #8625 ),
 .UNSPECIFIED., .F., .F. ) 
 B_SPLINE_CURVE_WITH_KNOTS ( ( 3, 2, 2, 2, 3 ),
 ( 0.8250000000000000666, 0.8333333333333333703, 0.8499999999999999778, 0.8666666666666666963, 0.8750000000000000000 ),
 .UNSPECIFIED. ) 
 CURVE ( )  GEOMETRIC_REPRESENTATION_ITEM ( )  RATIONAL_B_SPLINE_CURVE ( ( 0.9330127018922194093, 0.9330127018922198534, 1.000000000000000000, 0.8660254037844387076, 1.000000000000000000, 0.8660254037844387076, 1.000000000000000000, 0.9330127018922194093, 0.9330127018922194093 ) ) 
 REPRESENTATION_ITEM ( '' )  );
#12753=CARTESIAN_POINT ( 'NONE',  ( 3.756430356249996994, -28.06562499938548427, 8.999999999999992895 ) ) ;
#12757=CARTESIAN_POINT ( 'NONE',  ( 2.875168806925156861, 29.86250404960532379, 11.79623638833883525 ) ) ;
#12761=EDGE_LOOP ( 'NONE', ( #6546, #5446, #9256 ) ) ;
#12766=CARTESIAN_POINT ( 'NONE',  ( 3.756430356249996105, -26.34062499938548285, 6.831223922626973533 ) ) ;
#12767=CARTESIAN_POINT ( 'NONE',  ( 4.000000000000001776, 25.86250000000000071, 11.30940107675849760 ) ) ;
#12772=EDGE_CURVE ( 'NONE', #18967, #10560, #21810, .T. ) ;
#12779=CARTESIAN_POINT ( 'NONE',  ( 19.60674521665374215, 19.60674521665367820, 13.33755215474602984 ) ) ;
#12780=CARTESIAN_POINT ( 'NONE',  ( 18.15054718871317974, 23.80740143820548482, 8.999999999999992895 ) ) ;
#12785=CARTESIAN_POINT ( 'NONE',  ( -1.859271017917182139E-15, -28.48749999999999716, 12.99999999999999289 ) ) ;
#12786=CARTESIAN_POINT ( 'NONE',  ( 19.78573162020706988, 19.78573162020698462, 12.99999999999999289 ) ) ;
#12788=ORIENTED_EDGE ( 'NONE', *, *, #17860, .T. ) ;
#12789=CARTESIAN_POINT ( 'NONE',  ( -1.999999999999998224, 28.39374999877096784, 12.46410161513774639 ) ) ;
#12790=CARTESIAN_POINT ( 'NONE',  ( 3.756430356249995661, -26.22812499938548214, 6.831223922626973533 ) ) ;
#12791=CARTESIAN_POINT ( 'NONE',  ( -3.999999999999995559, 25.58124999877096784, 6.690598923241487306 ) ) ;
#12795=CARTESIAN_POINT ( 'NONE',  ( -3.735045420075836212E-15, -26.60312499938547859, 4.662447845253954171 ) ) ;
#12796=ORIENTED_EDGE ( 'NONE', *, *, #2432, .F. ) ;
#12797=EDGE_LOOP ( 'NONE', ( #15084, #3143, #6313, #7708 ) ) ;
#12803=CARTESIAN_POINT ( 'NONE',  ( -4.000000000000003553, -27.19374999877096855, 8.999999999999992895 ) ) ;
#12804=CARTESIAN_POINT ( 'NONE',  ( 1.878215178125004048, 28.36562499938548143, 5.746835883940462963 ) ) ;
#12806=CARTESIAN_POINT ( 'NONE',  ( 1.071796769724488563, -28.91740381056766651, 12.99999999999999289 ) ) ;
#12810=CYLINDRICAL_SURFACE ( 'NONE', #5039, 4.000000000000000000 ) ;
#12811=CARTESIAN_POINT ( 'NONE',  ( 21.41845328966172346, 21.00795358153114378, 12.99999999999999112 ) ) ;
#12813=CARTESIAN_POINT ( 'NONE',  ( 1.878215178124995832, -26.75312499938548783, 5.746835883940462963 ) ) ;
#12817=CARTESIAN_POINT ( 'NONE',  ( 2.439210544738880326, -29.90146712018378494, 5.819033386899011617 ) ) ;
#12827=CYLINDRICAL_SURFACE ( 'NONE', #23075, 4.000000000000000000 ) ;
#12829=DIRECTION ( 'NONE',  ( 1.000000000000000000, 0.000000000000000000, 0.000000000000000000 ) ) ;
#12830=CARTESIAN_POINT ( 'NONE',  ( -3.756430356249996994, 29.52812499938548640, 8.999999999999992895 ) ) ;
#12833=CARTESIAN_POINT ( 'NONE',  ( 1.071796769724492338, 29.40759618943233278, 12.99999999999999467 ) ) ;
#12835=CARTESIAN_POINT ( 'NONE',  ( 3.735045420075836212E-15, 25.36562499938548498, 4.662447845253954171 ) ) ;
#12836=CARTESIAN_POINT ( 'NONE',  ( 19.58805710660147170, -17.18149551509900519, 20.00001200000000523 ) ) ;
#12842=DIRECTION ( 'NONE',  ( 0.000000000000000000, -1.000000000000000000, 0.000000000000000000 ) ) ;
#12852=CARTESIAN_POINT ( 'NONE',  ( -1.878215178125004048, -26.22812499938548569, 5.746835883940462963 ) ) ;
#12854=FACE_OUTER_BOUND ( 'NONE', #11658, .T. ) ;
#12860=CARTESIAN_POINT ( 'NONE',  ( -3.999999999999996447, 28.31874999877096855, 8.999999999999992895 ) ) ;
#12861=CARTESIAN_POINT ( 'NONE',  ( 16.02247018838703241, 21.33486494430570701, 11.16877607737301226 ) ) ;
#12865=CARTESIAN_POINT ( 'NONE',  ( -3.756430356249995661, 27.12812499938548427, 6.831223922626973533 ) ) ;
#12867=CARTESIAN_POINT ( 'NONE',  ( 22.10384356884614121, 16.79144881292732450, 8.999999999999992895 ) ) ;
#12873=CARTESIAN_POINT ( 'NONE',  ( -3.735045420075836212E-15, -28.40312499938548640, 4.662447845253954171 ) ) ;
#12879=ORIENTED_EDGE ( 'NONE', *, *, #11092, .T. ) ;
#12881=ADVANCED_FACE ( 'NONE', ( #9777, #8080 ), #16058, .T. ) ;
#12885=CARTESIAN_POINT ( 'NONE',  ( -2.672651547586948120E-15, -29.19062499938548427, 13.33755215474603162 ) ) ;
#12892=VECTOR ( 'NONE', #18832, 1000.000000000000000 ) ;
#12897=CARTESIAN_POINT ( 'NONE',  ( 19.50730832598392084, 19.50730832598383913, 12.99999999999999289 ) ) ;
#12898=AXIS2_PLACEMENT_3D ( 'NONE', #10561, #22739, #18421 ) ;
#12901=CARTESIAN_POINT ( 'NONE',  ( 18.56476993080373461, 20.08051945865570787, 4.999999999999992895 ) ) ;
#12903=CARTESIAN_POINT ( 'NONE',  ( 1.071796769724494336, 25.35759618943234628, 12.99999999999999467 ) ) ;
#12904=CARTESIAN_POINT ( 'NONE',  ( 22.97888821056449515, 17.66649345464567489, 8.999999999999992895 ) ) ;
#12905=CARTESIAN_POINT ( 'NONE',  ( 20.40451381974352074, 17.74831644178408041, 12.25316411605952283 ) ) ;
#12909=CARTESIAN_POINT ( 'NONE',  ( 3.834746474454188013E-15, 27.75624999877096855, 4.999999999999992006 ) ) ;
#12910=CARTESIAN_POINT ( 'NONE',  ( 16.20808571844850121, 21.52048047436717937, 6.831223922626973533 ) ) ;
#12914=CARTESIAN_POINT ( 'NONE',  ( 2.000000000000000888, 28.01874999877096784, 12.46410161513774817 ) ) ;
#12915=CARTESIAN_POINT ( 'NONE',  ( 3.756430356249997882, -28.55312499938548498, 11.16877607737301226 ) ) ;
#12922=CARTESIAN_POINT ( 'NONE',  ( 3.756430356249997882, -27.20312499938548001, 11.16877607737301226 ) ) ;
#12924=VERTEX_POINT ( 'NONE', #2823 ) ;
#12933=CARTESIAN_POINT ( 'NONE',  ( 2.672651547586948120E-15, 28.17812499938548143, 13.33755215474602984 ) ) ;
#12939=DIRECTION ( 'NONE',  ( 0.000000000000000000, 0.000000000000000000, -1.000000000000000000 ) ) ;
#12942=CARTESIAN_POINT ( 'NONE',  ( -1.878215178125000939, -26.97812499938548569, 12.25316411605952283 ) ) ;
#12949=CARTESIAN_POINT ( 'NONE',  ( -1.859271017917182139E-15, -28.48749999999999716, 12.99999999999999289 ) ) ;
#12950=ORIENTED_EDGE ( 'NONE', *, *, #8103, .F. ) ;
#12953=VERTEX_POINT ( 'NONE', #18396 ) ;
#12960=AXIS2_PLACEMENT_3D ( 'NONE', #9432, #17413, #19485 ) ;
#12961=EDGE_LOOP ( 'NONE', ( #3289, #5028, #24584 ) ) ;
#12967=CARTESIAN_POINT ( 'NONE',  ( 17.82559248041273037, 23.13798723633140142, 8.999999999999992895 ) ) ;
#12968=CARTESIAN_POINT ( 'NONE',  ( -3.756430356249996994, 26.82812499938548711, 8.999999999999992895 ) ) ;
#12969=CARTESIAN_POINT ( 'NONE',  ( 8.377607117416804527, -24.67207871933483787, 20.00001200000000168 ) ) ;
#12972=CARTESIAN_POINT ( 'NONE',  ( 21.21320343559646915, 21.21320343559638744, 8.999999999999992895 ) ) ;
#12980=EDGE_CURVE ( 'NONE', #11742, #19703, #5260, .T. ) ;
#12981=DIRECTION ( 'NONE',  ( 1.000000000000000000, 0.000000000000000000, 0.000000000000000000 ) ) ;
#12987=ORIENTED_EDGE ( 'NONE', *, *, #8977, .T. ) ;
#12990=CARTESIAN_POINT ( 'NONE',  ( 1.878215178124995832, -25.85312499938548569, 5.746835883940462963 ) ) ;
#12991=EDGE_CURVE ( 'NONE', #22105, #20014, #748, .T. ) ;
#12994=ORIENTED_EDGE ( 'NONE', *, *, #22581, .T. ) ;
#13001=CARTESIAN_POINT ( 'NONE',  ( 18.87091222291601866, 18.87091222291595827, 12.99999999999999289 ) ) ;
#13002=CARTESIAN_POINT ( 'NONE',  ( 17.58921741601718125, 20.24541479397648303, 5.746835883940462963 ) ) ;
#13005=CARTESIAN_POINT ( 'NONE',  ( 4.000000000000003553, 25.03749999999999787, 6.690598923241489970 ) ) ;
#13006=CARTESIAN_POINT ( 'NONE',  ( 16.28763523133199342, 21.60002998725066803, 6.831223922626973533 ) ) ;
#13011=CARTESIAN_POINT ( 'NONE',  ( -2.672651547586948120E-15, -28.17812499938548143, 13.33755215474603162 ) ) ;
#13017=LINE ( 'NONE', #9080, #25493 ) ;
#13034=VECTOR ( 'NONE', #1208, 1000.000000000000000 ) ;
#13038=CYLINDRICAL_SURFACE ( 'NONE', #22616, 4.000000000000000000 ) ;
#13039=CARTESIAN_POINT ( 'NONE',  ( 3.756430356250002323, 26.45312499938548356, 11.16877607737301403 ) ) ;
#13040=CARTESIAN_POINT ( 'NONE',  ( 19.73390110347460435, 18.21815157562248544, 4.999999999999989342 ) ) ;
#13041=CARTESIAN_POINT ( 'NONE',  ( 18.14379053194667790, 23.45618528786534895, 8.999999999999992895 ) ) ;
#13042=CARTESIAN_POINT ( 'NONE',  ( 19.87418373385361292, 17.21798635589416548, 5.746835883940462963 ) ) ;
#13046=AXIS2_PLACEMENT_3D ( 'NONE', #3261, #11239, #1316 ) ;
#13047=CARTESIAN_POINT ( 'NONE',  ( 19.12944813935283150, 19.12944813935275690, 4.662447845253954171 ) ) ;
#13048=CARTESIAN_POINT ( 'NONE',  ( 22.66719175354223736, 17.01033750404978662, 11.30940107675849760 ) ) ;
#13049=VERTEX_POINT ( 'NONE', #7005 ) ;
#13051=CARTESIAN_POINT ( 'NONE',  ( -3.999999999999996447, 27.41874999877096641, 8.999999999999992895 ) ) ;
#13052=CARTESIAN_POINT ( 'NONE',  ( 1.878215178124998497, -28.14062499938548356, 12.25316411605951927 ) ) ;
#13054=ORIENTED_EDGE ( 'NONE', *, *, #18264, .T. ) ;
#13057=VECTOR ( 'NONE', #6801, 1000.000000000000000 ) ;
#13060=CARTESIAN_POINT ( 'NONE',  ( -3.756430356250003655, -29.19062499938548072, 8.999999999999992895 ) ) ;
#13066=CARTESIAN_POINT ( 'NONE',  ( 0.000000000000000000, 0.000000000000000000, 20.00000000000000000 ) ) ;
#13070=CARTESIAN_POINT ( 'NONE',  ( 1.878215178125000939, 27.31562499938548427, 12.25316411605952283 ) ) ;
#13080=CARTESIAN_POINT ( 'NONE',  ( 3.756430356249996994, -27.27812499938548640, 8.999999999999992895 ) ) ;
#13089=ORIENTED_EDGE ( 'NONE', *, *, #7830, .F. ) ;
#13098=CARTESIAN_POINT ( 'NONE',  ( -3.756430356249996105, 27.69062499938548072, 6.831223922626973533 ) ) ;
#13105=CARTESIAN_POINT ( 'NONE',  ( 1.878215178125000939, 26.97812499938548569, 12.25316411605952283 ) ) ;
#13107=AXIS2_PLACEMENT_3D ( 'NONE', #13066, #7033, #7175 ) ;
#13108=CARTESIAN_POINT ( 'NONE',  ( -8.377607117416792093, -24.67207871933483787, 20.00001200000000168 ) ) ;
#13119=ORIENTED_EDGE ( 'NONE', *, *, #25823, .T. ) ;
#13123=CARTESIAN_POINT ( 'NONE',  ( -3.756430356250003655, -25.25312499938548427, 8.999999999999992895 ) ) ;
#13126=ORIENTED_EDGE ( 'NONE', *, *, #5533, .T. ) ;
#13128=( BOUNDED_CURVE ( )  B_SPLINE_CURVE ( 2, ( #503, #2970, #2445, #10406, #18405, #14611, #2583, #8473, #12511 ),
 .UNSPECIFIED., .F., .F. ) 
 B_SPLINE_CURVE_WITH_KNOTS ( ( 3, 2, 2, 2, 3 ),
 ( 0.7249999999999999778, 0.7333333333333332815, 0.7500000000000000000, 0.7666666666666667185, 0.7750000000000000222 ),
 .UNSPECIFIED. ) 
 CURVE ( )  GEOMETRIC_REPRESENTATION_ITEM ( )  RATIONAL_B_SPLINE_CURVE ( ( 0.9330127018922194093, 0.9330127018922194093, 1.000000000000000000, 0.8660254037844387076, 1.000000000000000000, 0.8660254037844387076, 1.000000000000000000, 0.9330127018922194093, 0.9330127018922194093 ) ) 
 REPRESENTATION_ITEM ( '' )  );
#13131=EDGE_CURVE ( 'NONE', #939, #21627, #19295, .T. ) ;
#13132=LINE ( 'NONE', #21101, #1301 ) ;
#13134=CARTESIAN_POINT ( 'NONE',  ( 17.05888733012726632, 19.71508470808657520, 12.25316411605951927 ) ) ;
#13140=CARTESIAN_POINT ( 'NONE',  ( 3.752267015613588906E-15, 26.01249999999999929, 4.381197846482986158 ) ) ;
#13141=CARTESIAN_POINT ( 'NONE',  ( 21.14924941424430571, 15.83685465832548900, 8.999999999999992895 ) ) ;
#13143=VERTEX_POINT ( 'NONE', #9366 ) ;
#13157=CARTESIAN_POINT ( 'NONE',  ( -3.999999999999997335, 25.71249999999999503, 11.30940107675849404 ) ) ;
#13159=CARTESIAN_POINT ( 'NONE',  ( -1.071796769724492338, -26.20134618820330275, 12.99999999999999467 ) ) ;
#13167=CARTESIAN_POINT ( 'NONE',  ( -3.756430356249996105, 27.57812499938548356, 6.831223922626973533 ) ) ;
#13169=CARTESIAN_POINT ( 'NONE',  ( 15.35305598651295256, 21.00991023600526830, 11.30940107675849404 ) ) ;
#13170=CARTESIAN_POINT ( 'NONE',  ( 23.96650046397252609, 18.30964621448006824, 8.999999999999992895 ) ) ;
#13171=EDGE_CURVE ( 'NONE', #1111, #17932, #1638, .T. ) ;
#13175=CARTESIAN_POINT ( 'NONE',  ( 21.36138144860026600, 16.04898669268145639, 11.16877607737301403 ) ) ;
#13177=ORIENTED_EDGE ( 'NONE', *, *, #21385, .F. ) ;
#13179=CARTESIAN_POINT ( 'NONE',  ( 4.000000000000003553, 28.09374999877097068, 8.999999999999992895 ) ) ;
#13180=CARTESIAN_POINT ( 'NONE',  ( -1.878215178125004048, -28.36562499938548143, 5.746835883940462963 ) ) ;
#13184=ORIENTED_EDGE ( 'NONE', *, *, #16159, .T. ) ;
#13185=CARTESIAN_POINT ( 'NONE',  ( -1.878215178125004048, -27.01562499938548711, 5.746835883940462963 ) ) ;
#13197=CARTESIAN_POINT ( 'NONE',  ( -1.999999999999995781, 26.89374999877097139, 5.535898384862237620 ) ) ;
#13202=CARTESIAN_POINT ( 'NONE',  ( 3.756430356249997882, -28.21562499938548285, 11.16877607737301226 ) ) ;
#13206=CARTESIAN_POINT ( 'NONE',  ( 1.859271017917182139E-15, 26.18124999877096570, 12.99999999999999289 ) ) ;
#13207=CARTESIAN_POINT ( 'NONE',  ( 21.04646806692120009, 19.53071853906906341, 4.999999999999997335 ) ) ;
#13211=ORIENTED_EDGE ( 'NONE', *, *, #16872, .T. ) ;
#13214=EDGE_CURVE ( 'NONE', #13512, #421, #11060, .T. ) ;
#13220=CARTESIAN_POINT ( 'NONE',  ( 23.59283907696195115, 18.53082671639309353, 10.80044967790456845 ) ) ;
#13223=DIRECTION ( 'NONE',  ( 1.000000000000000000, 0.000000000000000000, 0.000000000000000000 ) ) ;
#13224=DIRECTION ( 'NONE',  ( 0.000000000000000000, 1.000000000000000000, 0.000000000000000000 ) ) ;
#13225=CARTESIAN_POINT ( 'NONE',  ( -1.071796769724491227, -26.83615380933863293, 4.999999999999989342 ) ) ;
#13226=CARTESIAN_POINT ( 'NONE',  ( 21.21320343559646915, 21.21320343559638744, 8.999999999999992895 ) ) ;
#13231=CARTESIAN_POINT ( 'NONE',  ( -4.000000000000001776, -26.70624999877097139, 11.30940107675849760 ) ) ;
#13233=EDGE_CURVE ( 'NONE', #4650, #22072, #21293, .T. ) ;
#13237=ORIENTED_EDGE ( 'NONE', *, *, #25353, .F. ) ;
#13239=EDGE_LOOP ( 'NONE', ( #25491, #18672, #15434, #1378 ) ) ;
#13241=PLANE ( 'NONE',  #17906 ) ;
#13242=ORIENTED_EDGE ( 'NONE', *, *, #11382, .T. ) ;
#13252=CARTESIAN_POINT ( 'NONE',  ( 15.65123912826409480, 20.96363388418277296, 6.831223922626973533 ) ) ;
#13254=CARTESIAN_POINT ( 'NONE',  ( 3.752267015613588906E-15, 25.11250000000000071, 4.381197846482986158 ) ) ;
#13255=CARTESIAN_POINT ( 'NONE',  ( 17.90741546755112523, 20.56361284551042701, 5.746835883940462963 ) ) ;
#13260=CARTESIAN_POINT ( 'NONE',  ( -3.469446951953614189E-15, -30.00000000000000355, 8.999999999999992895 ) ) ;
#13269=FACE_OUTER_BOUND ( 'NONE', #1980, .T. ) ;
#13274=CARTESIAN_POINT ( 'NONE',  ( -3.735045420075836212E-15, -28.96562499938548640, 4.662447845253954171 ) ) ;
#13278=CARTESIAN_POINT ( 'NONE',  ( -1.859271017917182139E-15, -26.18124999877096570, 12.99999999999999289 ) ) ;
#13283=DIRECTION ( 'NONE',  ( -0.000000000000000000, -1.000000000000000000, -0.000000000000000000 ) ) ;
#13285=CARTESIAN_POINT ( 'NONE',  ( 2.672651547586948120E-15, 27.27812499938548640, 13.33755215474603162 ) ) ;
#13286=CARTESIAN_POINT ( 'NONE',  ( -1.294650675951837693, -29.97301818707614984, 5.206367449752296039 ) ) ;
#13287=CARTESIAN_POINT ( 'NONE',  ( 23.27056975780394765, 17.95817500188513094, 11.16877607737301226 ) ) ;
#13288=CARTESIAN_POINT ( 'NONE',  ( 20.32269083260512588, 20.32269083260505838, 13.33755215474602984 ) ) ;
#13293=CARTESIAN_POINT ( 'NONE',  ( 18.78246010926947918, 21.43865748722877740, 5.746835883940462963 ) ) ;
#13294=CARTESIAN_POINT ( 'NONE',  ( 21.33252770405263732, 18.50410057930636754, 5.535898384862238508 ) ) ;
#13298=CARTESIAN_POINT ( 'NONE',  ( -3.999999999999997335, 29.25624999877096499, 11.30940107675849404 ) ) ;
#13299=CARTESIAN_POINT ( 'NONE',  ( -3.756430356250003655, -29.64062499938548356, 8.999999999999992895 ) ) ;
#13300=CARTESIAN_POINT ( 'NONE',  ( 1.859271017917182139E-15, 25.78750000000000142, 12.99999999999999289 ) ) ;
#13304=CARTESIAN_POINT ( 'NONE',  ( -22.56362157461194329, 13.02991752792602931, 20.00001200000000168 ) ) ;
#13305=CARTESIAN_POINT ( 'NONE',  ( 3.756430356249996994, -28.06562499938548427, 8.999999999999992895 ) ) ;
#13320=FACE_OUTER_BOUND ( 'NONE', #4818, .T. ) ;
#13325=CARTESIAN_POINT ( 'NONE',  ( -1.071796769724481901, 27.56740381056766864, 12.99999999999999645 ) ) ;
#13326=CARTESIAN_POINT ( 'NONE',  ( -3.756430356250003655, -28.85312499938548569, 8.999999999999992895 ) ) ;
#13330=CARTESIAN_POINT ( 'NONE',  ( 18.71181319714904490, 18.71181319714897739, 4.999999999999991118 ) ) ;
#13331=CARTESIAN_POINT ( 'NONE',  ( 20.30280345481879323, 20.30280345481869730, 4.999999999999992006 ) ) ;
#13340=AXIS2_PLACEMENT_3D ( 'NONE', #19845, #1690, #1945 ) ;
#13353=CARTESIAN_POINT ( 'NONE',  ( 0.000000000000000000, 0.000000000000000000, 0.000000000000000000 ) ) ;
#13355=CARTESIAN_POINT ( 'NONE',  ( -3.756430356249995661, 25.44062499938548427, 6.831223922626973533 ) ) ;
#13358=CARTESIAN_POINT ( 'NONE',  ( 25.99307600111999150, -0.5999999999999996447, 19.00000000000000000 ) ) ;
#13364=CARTESIAN_POINT ( 'NONE',  ( -2.000000000000000888, -28.01874999877096784, 12.46410161513774817 ) ) ;
#13366=CARTESIAN_POINT ( 'NONE',  ( 3.834746474454188013E-15, 27.75624999877096855, 4.999999999999992006 ) ) ;
#13376=CARTESIAN_POINT ( 'NONE',  ( -3.756430356250003655, -27.05312499938548498, 8.999999999999992895 ) ) ;
#13381=ORIENTED_EDGE ( 'NONE', *, *, #17409, .F. ) ;
#13387=CARTESIAN_POINT ( 'NONE',  ( 23.66831732222138740, 18.35592256630256003, 11.16877607737301226 ) ) ;
#13390=CARTESIAN_POINT ( 'NONE',  ( 4.000000000000003553, 26.35000000000000142, 8.999999999999992895 ) ) ;
#13394=CARTESIAN_POINT ( 'NONE',  ( 18.33167953626305646, 20.98787691422236179, 12.25316411605951927 ) ) ;
#13397=ORIENTED_EDGE ( 'NONE', *, *, #12571, .T. ) ;
#13399=CARTESIAN_POINT ( 'NONE',  ( -3.756430356250003211, -29.22812499938548569, 6.831223922626973533 ) ) ;
#13401=DIRECTION ( 'NONE',  ( 0.000000000000000000, 0.000000000000000000, 1.000000000000000000 ) ) ;
#13404=ORIENTED_EDGE ( 'NONE', *, *, #12222, .T. ) ;
#13405=ORIENTED_EDGE ( 'NONE', *, *, #1321, .T. ) ;
#13409=CARTESIAN_POINT ( 'NONE',  ( 23.68807716974937705, 18.03122292025692275, 8.999999999999992895 ) ) ;
#13412=CARTESIAN_POINT ( 'NONE',  ( -2.672651547586948120E-15, -28.29062499938548925, 13.33755215474603162 ) ) ;
#13413=EDGE_CURVE ( 'NONE', #16293, #11588, #952, .T. ) ;
#13422=CARTESIAN_POINT ( 'NONE',  ( -1.071796769724490117, 26.93259618943234202, 4.999999999999992895 ) ) ;
#13423=AXIS2_PLACEMENT_3D ( 'NONE', #17995, #84, #8056 ) ;
#13427=CARTESIAN_POINT ( 'NONE',  ( 3.756430356250003655, 26.49062499938548498, 8.999999999999992895 ) ) ;
#13429=CARTESIAN_POINT ( 'NONE',  ( 22.23415261606371374, 19.57795523810426630, 12.25316411605952283 ) ) ;
#13430=CARTESIAN_POINT ( 'NONE',  ( 23.40315227927642283, 18.09075752335759901, 6.831223922626973533 ) ) ;
#13432=( BOUNDED_CURVE ( )  B_SPLINE_CURVE ( 2, ( #150, #8121, #16096, #11640, #24060, #18189, #4049, #17920, #6143 ),
 .UNSPECIFIED., .F., .F. ) 
 B_SPLINE_CURVE_WITH_KNOTS ( ( 3, 2, 2, 2, 3 ),
 ( 0.02500000000000000139, 0.03333333333333333287, 0.05000000000000000278, 0.06666666666666666574, 0.07500000000000001110 ),
 .UNSPECIFIED. ) 
 CURVE ( )  GEOMETRIC_REPRESENTATION_ITEM ( )  RATIONAL_B_SPLINE_CURVE ( ( 0.9330127018922194093, 0.9330127018922194093, 1.000000000000000000, 0.8660254037844387076, 1.000000000000000000, 0.8660254037844387076, 1.000000000000000000, 0.9330127018922191873, 0.9330127018922192983 ) ) 
 REPRESENTATION_ITEM ( '' )  );
#13433=PLANE ( 'NONE',  #23993 ) ;
#13435=CARTESIAN_POINT ( 'NONE',  ( 1.859271017917182139E-15, 26.68750000000000000, 12.99999999999999289 ) ) ;
#13436=CARTESIAN_POINT ( 'NONE',  ( 21.67957950013421353, 16.36718474421539682, 11.16877607737301403 ) ) ;
#13440=CARTESIAN_POINT ( 'NONE',  ( 3.756430356250003655, 26.15312499938548640, 8.999999999999992895 ) ) ;
#13441=CARTESIAN_POINT ( 'NONE',  ( -4.000000000000003553, -25.90000000000000213, 8.999999999999992895 ) ) ;
#13448=CARTESIAN_POINT ( 'NONE',  ( -3.735045420075836212E-15, -28.85312499938548569, 4.662447845253954171 ) ) ;
#13451=CARTESIAN_POINT ( 'NONE',  ( 18.97562471959685126, 23.23703773337175349, 6.356496494711869616 ) ) ;
#13456=ADVANCED_FACE ( 'NONE', ( #21081 ), #3157, .F. ) ;
#13458=CARTESIAN_POINT ( 'NONE',  ( -2.000000000000000888, -27.17500000000000071, 12.46410161513774817 ) ) ;
#13463=CARTESIAN_POINT ( 'NONE',  ( 1.859271017917182139E-15, 28.48749999999999716, 12.99999999999999289 ) ) ;
#13464=CYLINDRICAL_SURFACE ( 'NONE', #9221, 4.000000000000000000 ) ;
#13466=CARTESIAN_POINT ( 'NONE',  ( 21.39439954740644723, 15.73754529791400181, 11.30940107675849760 ) ) ;
#13469=CARTESIAN_POINT ( 'NONE',  ( 3.756430356249996994, -28.17812499938548498, 8.999999999999992895 ) ) ;
#13470=VECTOR ( 'NONE', #1966, 1000.000000000000000 ) ;
#13473=DIRECTION ( 'NONE',  ( 0.000000000000000000, 0.000000000000000000, -1.000000000000000000 ) ) ;
#13474=CARTESIAN_POINT ( 'NONE',  ( 2.000000000000000888, 27.17500000000000071, 12.46410161513774817 ) ) ;
#13481=VERTEX_POINT ( 'NONE', #16910 ) ;
#13483=VERTEX_POINT ( 'NONE', #24876 ) ;
#13493=CARTESIAN_POINT ( 'NONE',  ( 3.756430356250003655, 27.50312499938548427, 8.999999999999992895 ) ) ;
#13494=CARTESIAN_POINT ( 'NONE',  ( 3.137519842735244810E-15, -26.85624999877096641, 4.999999999999991118 ) ) ;
#13500=CARTESIAN_POINT ( 'NONE',  ( -2.620986760973688460E-15, -27.08124999877096784, 13.61880215351699874 ) ) ;
#13511=CYLINDRICAL_SURFACE ( 'NONE', #17069, 4.000000000000000000 ) ;
#13512=VERTEX_POINT ( 'NONE', #25644 ) ;
#13513=CARTESIAN_POINT ( 'NONE',  ( 3.756430356249997882, -28.21562499938548285, 11.16877607737301226 ) ) ;
#13519=CARTESIAN_POINT ( 'NONE',  ( 3.063240906311874401, 29.84319947910909931, 11.57226653943513028 ) ) ;
#13521=CARTESIAN_POINT ( 'NONE',  ( 3.959305671612554781E-15, 30.00000000000000355, 12.99999999999999289 ) ) ;
#13522=CARTESIAN_POINT ( 'NONE',  ( 17.26874589022832751, 22.58114064614699856, 8.999999999999992895 ) ) ;
#13523=B_SPLINE_CURVE_WITH_KNOTS ( 'NONE', 3,
 ( #4446, #24458, #20387, #12418, #544, #4575, #6537, #12817, #4722, #12553, #280, #16224, #2243, #10198, #20533, #8248, #10587, #18581, #665, #6664, #12695, #1164, #25354, #16888, #3139, #18966, #10983, #19206, #5481, #2870, #9286, #9410, #21177, #9143 ),
 .UNSPECIFIED., .F., .F.,
 ( 4, 2, 2, 2, 2, 2, 2, 2, 2, 2, 2, 2, 2, 2, 2, 2, 4 ),
 ( 0.000000000000000000, 0.0007824850735655043557, 0.001564970147131008711, 0.002347455220696513176, 0.003129940294262017423, 0.003912425367827521670, 0.004694910441393026351, 0.005477395514958530165, 0.006259880588524034846, 0.007042365662089539527, 0.007824850735655043341, 0.008607335809220547154, 0.009389820882786052703, 0.01017230595635155652, 0.01095479102991706033, 0.01173727610348256588, 0.01251976117704806969 ),
 .UNSPECIFIED. ) ;
#13525=CARTESIAN_POINT ( 'NONE',  ( 3.752267015613588906E-15, 25.56250000000000000, 4.381197846482986158 ) ) ;
#13526=CARTESIAN_POINT ( 'NONE',  ( 23.03192121915348878, 17.71952646323466496, 11.16877607737301403 ) ) ;
#13528=ORIENTED_EDGE ( 'NONE', *, *, #24765, .T. ) ;
#13530=ORIENTED_EDGE ( 'NONE', *, *, #11449, .T. ) ;
#13537=CARTESIAN_POINT ( 'NONE',  ( -3.999999999999995559, 27.38124999877096855, 6.690598923241487306 ) ) ;
#13538=ORIENTED_EDGE ( 'NONE', *, *, #25028, .T. ) ;
#13540=EDGE_CURVE ( 'NONE', #130, #20899, #22829, .T. ) ;
#13546=( BOUNDED_CURVE ( )  B_SPLINE_CURVE ( 2, ( #7651, #15638, #24110, #9744, #10125, #13796, #71, #19674, #23862 ),
 .UNSPECIFIED., .F., .F. ) 
 B_SPLINE_CURVE_WITH_KNOTS ( ( 3, 2, 2, 2, 3 ),
 ( 0.3750000000000000000, 0.3833333333333333592, 0.4000000000000000222, 0.4166666666666666852, 0.4250000000000000444 ),
 .UNSPECIFIED. ) 
 CURVE ( )  GEOMETRIC_REPRESENTATION_ITEM ( )  RATIONAL_B_SPLINE_CURVE ( ( 0.9330127018922194093, 0.9330127018922194093, 1.000000000000000000, 0.8660254037844387076, 1.000000000000000000, 0.8660254037844387076, 1.000000000000000000, 0.9330127018922191873, 0.9330127018922194093 ) ) 
 REPRESENTATION_ITEM ( '' )  );
#13547=CARTESIAN_POINT ( 'NONE',  ( 21.21320343559646915, 21.21320343559638744, 4.999999999999992006 ) ) ;
#13549=CARTESIAN_POINT ( 'NONE',  ( -3.756430356249995661, 27.57812499938548356, 6.831223922626973533 ) ) ;
#13550=DIRECTION ( 'NONE',  ( 0.000000000000000000, -1.000000000000000000, 0.000000000000000000 ) ) ;
#13552=CARTESIAN_POINT ( 'NONE',  ( 3.756430356250003655, 27.84062499938548640, 8.999999999999992895 ) ) ;
#13553=CARTESIAN_POINT ( 'NONE',  ( 19.18911027444996975, 19.18911027444990225, 13.61880215351699874 ) ) ;
#13554=CARTESIAN_POINT ( 'NONE',  ( 16.60583328286593741, 21.91822803878461201, 6.831223922626973533 ) ) ;
#13556=CARTESIAN_POINT ( 'NONE',  ( 18.70297436238422506, 21.53140148713034208, 12.46410161513774639 ) ) ;
#13561=DIRECTION ( 'NONE',  ( 0.000000000000000000, 0.000000000000000000, -1.000000000000000000 ) ) ;
#13563=CARTESIAN_POINT ( 'NONE',  ( 21.43417430471724927, 15.77732005522480563, 11.30940107675849760 ) ) ;
#13564=CARTESIAN_POINT ( 'NONE',  ( -2.620986760973688460E-15, -26.68750000000000000, 13.61880215351699874 ) ) ;
#13565=CARTESIAN_POINT ( 'NONE',  ( 1.859271017917182139E-15, 29.33124999877096428, 12.99999999999999289 ) ) ;
#13569=CARTESIAN_POINT ( 'NONE',  ( -6.741346781237239405, 25.16843286583313954, 20.00001200000000168 ) ) ;
#13570=CARTESIAN_POINT ( 'NONE',  ( 1.878215178124998497, -29.49062499938548498, 12.25316411605951927 ) ) ;
#13571=ORIENTED_EDGE ( 'NONE', *, *, #17860, .F. ) ;
#13573=CARTESIAN_POINT ( 'NONE',  ( 1.878215178124995832, -25.40312499938548640, 5.746835883940462963 ) ) ;
#13578=CARTESIAN_POINT ( 'NONE',  ( 1.071796769724485454, -27.51115380933863719, 12.99999999999999467 ) ) ;
#13580=DIRECTION ( 'NONE',  ( 1.000000000000000000, 0.000000000000000000, 0.000000000000000000 ) ) ;
#13581=CARTESIAN_POINT ( 'NONE',  ( -2.875168806925156861, -29.86250404960532379, 11.79623638833883525 ) ) ;
#13584=CARTESIAN_POINT ( 'NONE',  ( 21.71259759894040187, 16.05574334944795112, 11.30940107675849760 ) ) ;
#13586=CARTESIAN_POINT ( 'NONE',  ( -4.000000000000003553, -27.64374999877096784, 8.999999999999992895 ) ) ;
#13587=CARTESIAN_POINT ( 'NONE',  ( 1.626862140677534194E-14, 27.58750000000000213, 12.99999999999999289 ) ) ;
#13588=( BOUNDED_CURVE ( )  B_SPLINE_CURVE ( 2, ( #22557, #8440, #6341, #20849, #20319, #2938, #16428, #14335, #14578 ),
 .UNSPECIFIED., .F., .F. ) 
 B_SPLINE_CURVE_WITH_KNOTS ( ( 3, 2, 2, 2, 3 ),
 ( 0.9250000000000000444, 0.9333333333333333481, 0.9499999999999999556, 0.9666666666666666741, 0.9749999999999999778 ),
 .UNSPECIFIED. ) 
 CURVE ( )  GEOMETRIC_REPRESENTATION_ITEM ( )  RATIONAL_B_SPLINE_CURVE ( ( 0.9330127018922194093, 0.9330127018922198534, 1.000000000000000000, 0.8660254037844387076, 1.000000000000000000, 0.8660254037844387076, 1.000000000000000000, 0.9330127018922194093, 0.9330127018922194093 ) ) 
 REPRESENTATION_ITEM ( '' )  );
#13591=CARTESIAN_POINT ( 'NONE',  ( -3.999999999999995559, 26.03124999877097068, 6.690598923241487306 ) ) ;
#13599=VECTOR ( 'NONE', #18310, 1000.000000000000000 ) ;
#13604=CARTESIAN_POINT ( 'NONE',  ( 3.959305671612554781E-15, 30.00000000000000355, 12.99999999999999289 ) ) ;
#13605=CARTESIAN_POINT ( 'NONE',  ( -2.000000000000000888, -28.01874999877096784, 12.46410161513774817 ) ) ;
#13611=CARTESIAN_POINT ( 'NONE',  ( 1.878215178125000939, 28.77812499938548640, 12.25316411605952283 ) ) ;
#13619=CARTESIAN_POINT ( 'NONE',  ( -4.000000000000001776, -26.25624999877096499, 11.30940107675849760 ) ) ;
#13620=CARTESIAN_POINT ( 'NONE',  ( 2.672651547586948120E-15, 27.39062499938548356, 13.33755215474602984 ) ) ;
#13621=DIRECTION ( 'NONE',  ( 0.000000000000000000, 0.000000000000000000, 1.000000000000000000 ) ) ;
#13629=ORIENTED_EDGE ( 'NONE', *, *, #3429, .F. ) ;
#13630=CARTESIAN_POINT ( 'NONE',  ( 1.878215178124995832, -27.65312499938548640, 5.746835883940462963 ) ) ;
#13633=EDGE_CURVE ( 'NONE', #11588, #6934, #18794, .T. ) ;
#13640=CARTESIAN_POINT ( 'NONE',  ( 17.85665593321704137, 17.85665593321697742, 4.662447845253954171 ) ) ;
#13643=CARTESIAN_POINT ( 'NONE',  ( 2.000000000000000888, 28.07500000000000284, 12.46410161513774817 ) ) ;
#13648=ORIENTED_EDGE ( 'NONE', *, *, #4012, .F. ) ;
#13651=DIRECTION ( 'NONE',  ( 0.000000000000000000, 1.000000000000000000, 0.000000000000000000 ) ) ;
#13658=DIRECTION ( 'NONE',  ( 0.000000000000000000, 1.000000000000000000, 0.000000000000000000 ) ) ;
#13661=DIRECTION ( 'NONE',  ( 0.000000000000000000, 0.000000000000000000, -1.000000000000000000 ) ) ;
#13663=ADVANCED_FACE ( 'NONE', ( #9309 ), #17294, .F. ) ;
#13665=CARTESIAN_POINT ( 'NONE',  ( -3.756430356249995661, 25.32812499938548356, 6.831223922626973533 ) ) ;
#13669=CARTESIAN_POINT ( 'NONE',  ( -1.042539689874651954, -29.98299368898127071, 5.129272290912049392 ) ) ;
#13670=CARTESIAN_POINT ( 'NONE',  ( 19.34820930021694352, 19.34820930021687246, 4.381197846482986158 ) ) ;
#13671=CARTESIAN_POINT ( 'NONE',  ( 21.99550407741325486, 19.33930669945380743, 12.25316411605952283 ) ) ;
#13679=CARTESIAN_POINT ( 'NONE',  ( -3.752267015613588906E-15, -26.46250000000000213, 4.381197846482986158 ) ) ;
#13692=ADVANCED_FACE ( 'NONE', ( #24326 ), #24059, .F. ) ;
#13700=CARTESIAN_POINT ( 'NONE',  ( -3.469446951953614189E-15, -30.00000000000000355, 8.999999999999992895 ) ) ;
#13702=CARTESIAN_POINT ( 'NONE',  ( 20.81103645292755289, 15.15418220343510392, 6.690598923241489970 ) ) ;
#13704=CARTESIAN_POINT ( 'NONE',  ( -3.999999999999997335, 27.51250000000000284, 11.30940107675849404 ) ) ;
#13705=CARTESIAN_POINT ( 'NONE',  ( 3.756430356249996994, -29.07812499938548356, 8.999999999999992895 ) ) ;
#13709=CARTESIAN_POINT ( 'NONE',  ( 4.000000000000003553, 29.03124999877096712, 6.690598923241489970 ) ) ;
#13713=DIRECTION ( 'NONE',  ( 1.000000000000000000, 0.000000000000000000, 0.000000000000000000 ) ) ;
#13727=( NAMED_UNIT ( * ) PLANE_ANGLE_UNIT ( ) SI_UNIT ( $, .RADIAN. ) );
#13729=( BOUNDED_CURVE ( )  B_SPLINE_CURVE ( 2, ( #16551, #6592, #12229, #6081, #14066, #22032, #210, #8180, #4254 ),
 .UNSPECIFIED., .F., .F. ) 
 B_SPLINE_CURVE_WITH_KNOTS ( ( 3, 2, 2, 2, 3 ),
 ( 0.6750000000000000444, 0.6833333333333333481, 0.6999999999999999556, 0.7166666666666666741, 0.7249999999999999778 ),
 .UNSPECIFIED. ) 
 CURVE ( )  GEOMETRIC_REPRESENTATION_ITEM ( )  RATIONAL_B_SPLINE_CURVE ( ( 0.9330127018922194093, 0.9330127018922198534, 1.000000000000000000, 0.8660254037844387076, 1.000000000000000000, 0.8660254037844387076, 1.000000000000000000, 0.9330127018922194093, 0.9330127018922194093 ) ) 
 REPRESENTATION_ITEM ( '' )  );
#13730=CARTESIAN_POINT ( 'NONE',  ( -1.878215178124995832, 28.55312499938548498, 5.746835883940462963 ) ) ;
#13736=VECTOR ( 'NONE', #1910, 999.9999999999998863 ) ;
#13740=CARTESIAN_POINT ( 'NONE',  ( -3.752267015613588906E-15, -27.30624999877097281, 4.381197846482986158 ) ) ;
#13741=CARTESIAN_POINT ( 'NONE',  ( -3.756430356249995661, 29.04062499938548569, 6.831223922626973533 ) ) ;
#13746=CARTESIAN_POINT ( 'NONE',  ( 1.999999999999995781, -25.99374999877096926, 5.535898384862237620 ) ) ;
#13750=DIRECTION ( 'NONE',  ( 0.000000000000000000, 0.000000000000000000, -1.000000000000000000 ) ) ;
#13752=CARTESIAN_POINT ( 'NONE',  ( 1.878215178124995832, -28.55312499938548498, 5.746835883940462963 ) ) ;
#13760=CIRCLE ( 'NONE', #12500, 0.7500000000000001110 ) ;
#13763=CARTESIAN_POINT ( 'NONE',  ( 17.58694394176227149, 22.89933869768094610, 8.999999999999992895 ) ) ;
#13769=CARTESIAN_POINT ( 'NONE',  ( 4.000000000000003553, 29.05000000000000071, 8.999999999999992895 ) ) ;
#13774=DIRECTION ( 'NONE',  ( -0.000000000000000000, -0.000000000000000000, 1.000000000000000000 ) ) ;
#13778=ADVANCED_FACE ( 'NONE', ( #23938 ), #21974, .F. ) ;
#13783=LINE ( 'NONE', #21760, #920 ) ;
#13796=CARTESIAN_POINT ( 'NONE',  ( -4.000000000000003553, -26.83749999999999503, 6.690598923241489970 ) ) ;
#13800=CARTESIAN_POINT ( 'NONE',  ( 20.46190248058575634, 20.46190248058568173, 12.99999999999999289 ) ) ;
#13802=CARTESIAN_POINT ( 'NONE',  ( 21.26623644418545211, 18.43780931943919299, 12.46410161513774817 ) ) ;
#13803=CARTESIAN_POINT ( 'NONE',  ( 20.16359180683815921, 20.16359180683807750, 4.662447845253954171 ) ) ;
#13808=DIRECTION ( 'NONE',  ( -0.7071067811865487940, -0.7071067811865463515, 0.000000000000000000 ) ) ;
#13810=CARTESIAN_POINT ( 'NONE',  ( 22.23415261606371374, 19.57795523810426630, 12.25316411605952283 ) ) ;
#13814=CARTESIAN_POINT ( 'NONE',  ( 1.999999999999998224, -27.10000000000000142, 12.46410161513774639 ) ) ;
#13821=CARTESIAN_POINT ( 'NONE',  ( 1.999999999999995781, -29.59374999877096712, 5.535898384862237620 ) ) ;
#13822=CARTESIAN_POINT ( 'NONE',  ( 20.67279826512042007, 15.85973458909327860, 20.00001200000000523 ) ) ;
#13823=LINE ( 'NONE', #5972, #25510 ) ;
#13824=EDGE_LOOP ( 'NONE', ( #6006, #7371, #16758, #24976 ) ) ;
#13825=ORIENTED_EDGE ( 'NONE', *, *, #24499, .T. ) ;
#13826=( NAMED_UNIT ( * ) SI_UNIT ( $, .STERADIAN. ) SOLID_ANGLE_UNIT ( ) );
#13838=CARTESIAN_POINT ( 'NONE',  ( 16.87327180006579752, 19.52946917802510285, 5.746835883940462963 ) ) ;
#13839=CARTESIAN_POINT ( 'NONE',  ( -3.469446951953614189E-15, -30.00000000000000355, 4.999999999999992006 ) ) ;
#13842=CARTESIAN_POINT ( 'NONE',  ( 2.007320019195686811, 29.93357098804190741, 5.530155478426868498 ) ) ;
#13869=CARTESIAN_POINT ( 'NONE',  ( 3.735045420075836212E-15, 29.41562499938548569, 4.662447845253954171 ) ) ;
#13878=CARTESIAN_POINT ( 'NONE',  ( -2.000000000000003997, -29.51874999877096784, 5.535898384862238508 ) ) ;
#13880=CARTESIAN_POINT ( 'NONE',  ( -1.878215178124998497, 27.35312499938548569, 12.25316411605951927 ) ) ;
#13882=DIRECTION ( 'NONE',  ( 0.7071067811865487940, 0.7071067811865463515, 0.000000000000000000 ) ) ;
#13886=CARTESIAN_POINT ( 'NONE',  ( 2.000000000000003997, 28.22500000000000142, 5.535898384862238508 ) ) ;
#13893=CARTESIAN_POINT ( 'NONE',  ( -1.878215178125000939, -26.41562499938548214, 12.25316411605952283 ) ) ;
#13900=CARTESIAN_POINT ( 'NONE',  ( -3.756430356249997438, 25.51562499938548356, 11.16877607737301048 ) ) ;
#13901=ADVANCED_FACE ( 'NONE', ( #16605 ), #12810, .F. ) ;
#13904=CARTESIAN_POINT ( 'NONE',  ( 23.35011927068743276, 18.03772451476861605, 11.16877607737301226 ) ) ;
#13909=CARTESIAN_POINT ( 'NONE',  ( -3.999999999999996447, 29.27500000000000213, 8.999999999999992895 ) ) ;
#13912=CARTESIAN_POINT ( 'NONE',  ( 20.64088888413907696, 20.64088888413900236, 13.33755215474603162 ) ) ;
#13915=VERTEX_POINT ( 'NONE', #11097 ) ;
#13920=CARTESIAN_POINT ( 'NONE',  ( 3.735045420075836212E-15, 26.71562499938548640, 4.662447845253954171 ) ) ;
#13921=CARTESIAN_POINT ( 'NONE',  ( -3.469446951953614189E-15, -30.00000000000000355, 4.999999999999992006 ) ) ;
#13924=EDGE_LOOP ( 'NONE', ( #20697, #5484, #24440, #3045 ) ) ;
#13925=AXIS2_PLACEMENT_3D ( 'NONE', #4235, #12214, #20183 ) ;
#13937=CARTESIAN_POINT ( 'NONE',  ( 3.756430356250003655, 26.49062499938548498, 8.999999999999992895 ) ) ;
#13940=LINE ( 'NONE', #7782, #13736 ) ;
#13941=CARTESIAN_POINT ( 'NONE',  ( 21.37230246136343581, 18.54387533661716958, 5.535898384862238508 ) ) ;
#13943=FACE_OUTER_BOUND ( 'NONE', #22039, .T. ) ;
#13949=CARTESIAN_POINT ( 'NONE',  ( 3.999999999999996447, -27.47499999999999787, 8.999999999999992895 ) ) ;
#13962=EDGE_CURVE ( 'NONE', #17313, #17328, #10702, .T. ) ;
#13972=CARTESIAN_POINT ( 'NONE',  ( 21.42091605170094937, 15.76406180220850040, 8.999999999999992895 ) ) ;
#13977=CARTESIAN_POINT ( 'NONE',  ( -1.289143957944685281, 29.97326948525437729, 12.79562863665509553 ) ) ;
#13978=CARTESIAN_POINT ( 'NONE',  ( -1.071796769724485454, 26.61115380933863150, 12.99999999999999467 ) ) ;
#13979=DIRECTION ( 'NONE',  ( -0.7071067811865487940, -0.7071067811865463515, 0.000000000000000000 ) ) ;
#13980=ORIENTED_EDGE ( 'NONE', *, *, #14998, .T. ) ;
#13983=CARTESIAN_POINT ( 'NONE',  ( -1.626862140677534194E-14, -27.98124999877096997, 12.99999999999999289 ) ) ;
#13988=VERTEX_POINT ( 'NONE', #22756 ) ;
#13997=CARTESIAN_POINT ( 'NONE',  ( 3.735045420075836212E-15, 28.06562499938548427, 4.662447845253954171 ) ) ;
#13998=EDGE_CURVE ( 'NONE', #20149, #8491, #3262, .T. ) ;
#14005=CARTESIAN_POINT ( 'NONE',  ( -4.000000000000003553, -29.44374999877096855, 8.999999999999992895 ) ) ;
#14007=CARTESIAN_POINT ( 'NONE',  ( 3.756430356250002323, 28.36562499938548854, 11.16877607737301226 ) ) ;
#14018=CARTESIAN_POINT ( 'NONE',  ( 0.000000000000000000, 0.000000000000000000, 19.59999999999999787 ) ) ;
#14025=AXIS2_PLACEMENT_3D ( 'NONE', #2152, #10119, #18119 ) ;
#14027=CARTESIAN_POINT ( 'NONE',  ( -3.756430356249996994, 25.47812499938548569, 8.999999999999992895 ) ) ;
#14031=CARTESIAN_POINT ( 'NONE',  ( 17.29753586877772520, 19.95373324673703408, 12.25316411605951927 ) ) ;
#14034=CARTESIAN_POINT ( 'NONE',  ( -3.999999999999996447, 27.92500000000000071, 8.999999999999992895 ) ) ;
#14035=CARTESIAN_POINT ( 'NONE',  ( 3.756430356250003655, 28.74062499938548498, 8.999999999999992895 ) ) ;
#14037=CARTESIAN_POINT ( 'NONE',  ( 20.79998790990604718, 20.79998790990596902, 4.662447845253954171 ) ) ;
#14046=CARTESIAN_POINT ( 'NONE',  ( 2.672651547586948120E-15, 25.59062499938548640, 13.33755215474602984 ) ) ;
#14047=CARTESIAN_POINT ( 'NONE',  ( 18.51293941407127974, 18.51293941407120869, 12.99999999999999112 ) ) ;
#14050=DIRECTION ( 'NONE',  ( 0.000000000000000000, 0.000000000000000000, -1.000000000000000000 ) ) ;
#14060=CARTESIAN_POINT ( 'NONE',  ( -3.834746474454188013E-15, -28.65624999877096712, 4.999999999999992006 ) ) ;
#14063=CARTESIAN_POINT ( 'NONE',  ( 21.80540536484019043, 16.14855111534773968, 6.690598923241489970 ) ) ;
#14066=CARTESIAN_POINT ( 'NONE',  ( 23.01190630937068349, 17.35505205987822919, 8.999999999999992895 ) ) ;
#14068=CARTESIAN_POINT ( 'NONE',  ( 18.11727402765218287, 23.42966878357085037, 6.831223922626973533 ) ) ;
#14076=CARTESIAN_POINT ( 'NONE',  ( -3.469446951953614189E-15, -30.00000000000000355, 8.999999999999992895 ) ) ;
#14077=DIRECTION ( 'NONE',  ( 0.000000000000000000, 0.000000000000000000, -1.000000000000000000 ) ) ;
#14080=CARTESIAN_POINT ( 'NONE',  ( 3.756430356249996994, -25.47812499938548569, 8.999999999999992895 ) ) ;
#14086=EDGE_CURVE ( 'NONE', #23081, #14590, #23971, .T. ) ;
#14087=DIRECTION ( 'NONE',  ( -1.000000000000000000, 0.000000000000000000, 0.000000000000000000 ) ) ;
#14090=CARTESIAN_POINT ( 'NONE',  ( 19.18911027444997686, 19.18911027444989870, 12.99999999999999112 ) ) ;
#14094=CARTESIAN_POINT ( 'NONE',  ( 16.90427148687188819, 22.56112573636419683, 11.30940107675849404 ) ) ;
#14096=CARTESIAN_POINT ( 'NONE',  ( 3.999999999999997335, -27.06250000000000000, 11.30940107675849404 ) ) ;
#14105=CARTESIAN_POINT ( 'NONE',  ( 2.620986760973688460E-15, 26.18124999877096926, 13.61880215351699874 ) ) ;
#14107=CARTESIAN_POINT ( 'NONE',  ( 3.756430356250003655, 29.64062499938548356, 8.999999999999992895 ) ) ;
#14108=ORIENTED_EDGE ( 'NONE', *, *, #11237, .T. ) ;
#14109=ADVANCED_FACE ( 'NONE', ( #1294 ), #13464, .F. ) ;
#14122=CARTESIAN_POINT ( 'NONE',  ( 1.878215178125000939, 26.41562499938548214, 12.25316411605952283 ) ) ;
#14127=CARTESIAN_POINT ( 'NONE',  ( -4.000000000000003553, -29.89374999877096784, 8.999999999999992895 ) ) ;
#14129=CARTESIAN_POINT ( 'NONE',  ( -3.735045420075836212E-15, -25.36562499938548498, 4.662447845253954171 ) ) ;
#14130=CARTESIAN_POINT ( 'NONE',  ( 3.756430356250003655, 27.95312499938548711, 8.999999999999992895 ) ) ;
#14134=ADVANCED_BREP_SHAPE_REPRESENTATION ( '', ( #4848, #21036 ), #8093 ) ;
#14137=EDGE_LOOP ( 'NONE', ( #25655, #16723, #24068, #673 ) ) ;
#14138=CARTESIAN_POINT ( 'NONE',  ( -3.756430356250003655, -29.75312499938548783, 8.999999999999992895 ) ) ;
#14141=AXIS2_PLACEMENT_3D ( 'NONE', #12972, #1072, #5372 ) ;
#14142=ORIENTED_EDGE ( 'NONE', *, *, #16568, .F. ) ;
#14150=CARTESIAN_POINT ( 'NONE',  ( -1.878215178124998497, 27.35312499938548569, 12.25316411605951927 ) ) ;
#14151=CIRCLE ( 'NONE', #22925, 4.000000000000000000 ) ;
#14154=CARTESIAN_POINT ( 'NONE',  ( 15.91640417120904871, 21.22879892712773042, 8.999999999999992895 ) ) ;
#14160=CARTESIAN_POINT ( 'NONE',  ( -3.999999999999997335, 27.51250000000000284, 11.30940107675849404 ) ) ;
#14161=CARTESIAN_POINT ( 'NONE',  ( 1.878215178125000939, 28.21562499938548640, 12.25316411605952283 ) ) ;
#14164=ORIENTED_EDGE ( 'NONE', *, *, #9183, .T. ) ;
#14170=EDGE_CURVE ( 'NONE', #18087, #3297, #21169, .T. ) ;
#14171=CARTESIAN_POINT ( 'NONE',  ( -1.999999999999998224, 29.74374999877096926, 12.46410161513774639 ) ) ;
#14173=CARTESIAN_POINT ( 'NONE',  ( -1.999999999999998224, 26.20000000000000284, 12.46410161513774639 ) ) ;
#14182=CARTESIAN_POINT ( 'NONE',  ( 2.000000000000003997, 29.12500000000000000, 5.535898384862238508 ) ) ;
#14185=CARTESIAN_POINT ( 'NONE',  ( -1.057460391440397258E-14, 29.55624999877096926, 4.999999999999992006 ) ) ;
#14191=CARTESIAN_POINT ( 'NONE',  ( 1.071796769724488563, -28.86115380933863506, 12.99999999999999289 ) ) ;
#14195=CARTESIAN_POINT ( 'NONE',  ( -4.000000000000003553, -28.54374999877096997, 8.999999999999992895 ) ) ;
#14196=DIRECTION ( 'NONE',  ( 0.000000000000000000, 0.000000000000000000, -1.000000000000000000 ) ) ;
#14198=DIRECTION ( 'NONE',  ( 0.000000000000000000, 1.000000000000000000, 0.000000000000000000 ) ) ;
#14200=ORIENTED_EDGE ( 'NONE', *, *, #24748, .T. ) ;
#14202=CARTESIAN_POINT ( 'NONE',  ( -2.000000000000003997, -28.22500000000000142, 5.535898384862238508 ) ) ;
#14205=EDGE_CURVE ( 'NONE', #18284, #22563, #6091, .T. ) ;
#14212=CARTESIAN_POINT ( 'NONE',  ( 3.756430356249996994, -27.72812499938548569, 8.999999999999992895 ) ) ;
#14215=VECTOR ( 'NONE', #22383, 1000.000000000000000 ) ;
#14216=ADVANCED_FACE ( 'NONE', ( #12380 ), #14227, .F. ) ;
#14223=AXIS2_PLACEMENT_3D ( 'NONE', #3182, #17322, #25285 ) ;
#14227=CYLINDRICAL_SURFACE ( 'NONE', #1620, 4.000000000000000000 ) ;
#14228=CARTESIAN_POINT ( 'NONE',  ( 18.14606400620158411, 20.80226138416088588, 5.746835883940462963 ) ) ;
#14229=CARTESIAN_POINT ( 'NONE',  ( 21.54465973840859760, 18.71623261366233848, 12.46410161513774817 ) ) ;
#14233=CARTESIAN_POINT ( 'NONE',  ( 1.294650675951837693, 29.97301818707614984, 5.206367449752296039 ) ) ;
#14236=CARTESIAN_POINT ( 'NONE',  ( -3.595408253811773758, 29.78394301743083261, 10.77252090037689136 ) ) ;
#14241=DIRECTION ( 'NONE',  ( 0.000000000000000000, 0.000000000000000000, -1.000000000000000000 ) ) ;
#14242=CARTESIAN_POINT ( 'NONE',  ( -3.999999999999996447, 26.51874999877097139, 8.999999999999992895 ) ) ;
#14243=CARTESIAN_POINT ( 'NONE',  ( -2.672651547586948120E-15, -27.27812499938548285, 13.33755215474602984 ) ) ;
#14248=ORIENTED_EDGE ( 'NONE', *, *, #9037, .T. ) ;
#14261=CARTESIAN_POINT ( 'NONE',  ( 1.878215178125000939, 26.86562499938548498, 12.25316411605952283 ) ) ;
#14270=CARTESIAN_POINT ( 'NONE',  ( 1.999999999999998224, -28.39374999877096784, 12.46410161513774639 ) ) ;
#14283=VERTEX_POINT ( 'NONE', #15933 ) ;
#14287=CARTESIAN_POINT ( 'NONE',  ( 20.72827001538724900, 19.21252048753512298, 4.999999999999992895 ) ) ;
#14292=CARTESIAN_POINT ( 'NONE',  ( -1.878215178124995832, 26.30312499938548498, 5.746835883940462963 ) ) ;
#14296=CARTESIAN_POINT ( 'NONE',  ( 19.12944813935283150, 19.12944813935275334, 4.662447845253954171 ) ) ;
#14298=VECTOR ( 'NONE', #8273, 1000.000000000000000 ) ;
#14299=CARTESIAN_POINT ( 'NONE',  ( 17.52740933866159168, 23.18426358815389676, 6.690598923241487306 ) ) ;
#14304=CARTESIAN_POINT ( 'NONE',  ( 1.878215178125004048, 28.36562499938548143, 5.746835883940462963 ) ) ;
#14305=EDGE_CURVE ( 'NONE', #1228, #22272, #15789, .T. ) ;
#14307=CARTESIAN_POINT ( 'NONE',  ( -3.999999999999995559, 27.43750000000000000, 6.690598923241487306 ) ) ;
#14308=CARTESIAN_POINT ( 'NONE',  ( 1.859271017917182139E-15, 29.38749999999999929, 12.99999999999999289 ) ) ;
#14314=AXIS2_PLACEMENT_3D ( 'NONE', #10834, #1296, #17265 ) ;
#14317=ORIENTED_EDGE ( 'NONE', *, *, #19887, .T. ) ;
#14321=ORIENTED_EDGE ( 'NONE', *, *, #17409, .T. ) ;
#14326=CARTESIAN_POINT ( 'NONE',  ( 4.000000000000003553, 26.83749999999999503, 6.690598923241489970 ) ) ;
#14328=CARTESIAN_POINT ( 'NONE',  ( 4.000000000000002665, 29.73213749463701205, 9.470295877454901756 ) ) ;
#14331=CARTESIAN_POINT ( 'NONE',  ( 3.756430356250004099, 27.42812499938548143, 6.831223922626973533 ) ) ;
#14335=CARTESIAN_POINT ( 'NONE',  ( -1.071796769724488563, 29.36740381056767291, 12.99999999999999289 ) ) ;
#14337=CARTESIAN_POINT ( 'NONE',  ( 1.071796769724487230, -27.77634618820330559, 4.999999999999992006 ) ) ;
#14342=CARTESIAN_POINT ( 'NONE',  ( 3.999999999999996003, -28.78750000000000142, 6.690598923241487306 ) ) ;
#14351=CARTESIAN_POINT ( 'NONE',  ( -3.756430356250002323, -26.56562499938548783, 11.16877607737301403 ) ) ;
#14358=EDGE_CURVE ( 'NONE', #9527, #14695, #19453, .T. ) ;
#14361=DIRECTION ( 'NONE',  ( -0.7071067811865487940, -0.7071067811865463515, 0.000000000000000000 ) ) ;
#14362=DIRECTION ( 'NONE',  ( -0.000000000000000000, -0.000000000000000000, 1.000000000000000000 ) ) ;
#14363=CARTESIAN_POINT ( 'NONE',  ( 20.78010053211970032, 20.78010053211962926, 12.99999999999999289 ) ) ;
#14364=CARTESIAN_POINT ( 'NONE',  ( 19.68856820379214057, 17.03237082583270023, 12.25316411605952283 ) ) ;
#14365=CARTESIAN_POINT ( 'NONE',  ( 20.10392967174101031, 20.10392967174093926, 13.61880215351699874 ) ) ;
#14370=CARTESIAN_POINT ( 'NONE',  ( 21.21320343559646915, 21.21320343559638744, 4.999999999999992006 ) ) ;
#14373=CARTESIAN_POINT ( 'NONE',  ( 16.55507374853184999, 19.21127112649115531, 5.746835883940462963 ) ) ;
#14374=CARTESIAN_POINT ( 'NONE',  ( 1.999999999999998224, -28.00000000000000000, 12.46410161513774639 ) ) ;
#14376=CARTESIAN_POINT ( 'NONE',  ( 4.000000000000001776, 27.15624999877097423, 11.30940107675849760 ) ) ;
#14377=CARTESIAN_POINT ( 'NONE',  ( 4.000000000000003553, 26.74374999877096926, 8.999999999999992895 ) ) ;
#14378=CARTESIAN_POINT ( 'NONE',  ( -3.756430356250004099, -27.42812499938548143, 6.831223922626973533 ) ) ;
#14379=CARTESIAN_POINT ( 'NONE',  ( 3.369928719974892281E-15, 25.11250000000000426, 4.999999999999992006 ) ) ;
#14381=EDGE_CURVE ( 'NONE', #7537, #7733, #18628, .T. ) ;
#14382=ORIENTED_EDGE ( 'NONE', *, *, #3335, .T. ) ;
#14383=CARTESIAN_POINT ( 'NONE',  ( -3.756430356250003655, -25.14062499938548356, 8.999999999999992895 ) ) ;
#14388=CARTESIAN_POINT ( 'NONE',  ( 3.469446951953614189E-15, 25.00000000000000000, 8.999999999999992895 ) ) ;
#14389=( BOUNDED_CURVE ( )  B_SPLINE_CURVE ( 2, ( #17784, #25499, #13605, #21571, #1956, #15573, #8544, #23541, #9804 ),
 .UNSPECIFIED., .F., .F. ) 
 B_SPLINE_CURVE_WITH_KNOTS ( ( 3, 2, 2, 2, 3 ),
 ( 0.5750000000000000666, 0.5833333333333333703, 0.5999999999999999778, 0.6166666666666666963, 0.6250000000000000000 ),
 .UNSPECIFIED. ) 
 CURVE ( )  GEOMETRIC_REPRESENTATION_ITEM ( )  RATIONAL_B_SPLINE_CURVE ( ( 0.9330127018922194093, 0.9330127018922198534, 1.000000000000000000, 0.8660254037844387076, 1.000000000000000000, 0.8660254037844387076, 1.000000000000000000, 0.9330127018922194093, 0.9330127018922194093 ) ) 
 REPRESENTATION_ITEM ( '' )  );
#14392=CARTESIAN_POINT ( 'NONE',  ( 2.672651547586948120E-15, 25.47812499938548569, 13.33755215474602984 ) ) ;
#14399=CARTESIAN_POINT ( 'NONE',  ( 3.999999999999997335, -28.35624999877096997, 11.30940107675849404 ) ) ;
#14405=CARTESIAN_POINT ( 'NONE',  ( 0.7500000000000001110, 0.000000000000000000, 15.00000000000000178 ) ) ;
#14406=DIRECTION ( 'NONE',  ( 0.000000000000000000, 1.000000000000000000, 0.000000000000000000 ) ) ;
#14412=ORIENTED_EDGE ( 'NONE', *, *, #9364, .T. ) ;
#14415=ORIENTED_EDGE ( 'NONE', *, *, #13233, .F. ) ;
#14417=CARTESIAN_POINT ( 'NONE',  ( -1.878215178124998497, 26.00312499938548783, 12.25316411605951927 ) ) ;
#14418=AXIS2_PLACEMENT_3D ( 'NONE', #7382, #19410, #25183 ) ;
#14421=CARTESIAN_POINT ( 'NONE',  ( 21.09621640565530853, 15.78382164973649537, 6.831223922626973533 ) ) ;
#14426=CARTESIAN_POINT ( 'NONE',  ( 1.878215178125000939, 29.11562499938548498, 12.25316411605952283 ) ) ;
#14429=DIRECTION ( 'NONE',  ( 0.000000000000000000, 0.000000000000000000, -1.000000000000000000 ) ) ;
#14433=( BOUNDED_CURVE ( )  B_SPLINE_CURVE ( 2, ( #24453, #10704, #400, #4183, #6531, #660, #8369, #14647, #778 ),
 .UNSPECIFIED., .F., .F. ) 
 B_SPLINE_CURVE_WITH_KNOTS ( ( 3, 2, 2, 2, 3 ),
 ( 0.7249999999999999778, 0.7333333333333332815, 0.7500000000000000000, 0.7666666666666667185, 0.7750000000000000222 ),
 .UNSPECIFIED. ) 
 CURVE ( )  GEOMETRIC_REPRESENTATION_ITEM ( )  RATIONAL_B_SPLINE_CURVE ( ( 0.9330127018922194093, 0.9330127018922194093, 1.000000000000000000, 0.8660254037844387076, 1.000000000000000000, 0.8660254037844387076, 1.000000000000000000, 0.9330127018922194093, 0.9330127018922194093 ) ) 
 REPRESENTATION_ITEM ( '' )  );
#14438=CARTESIAN_POINT ( 'NONE',  ( -1.071796769724487230, 26.03259618943233278, 4.999999999999992006 ) ) ;
#14444=ADVANCED_FACE ( 'NONE', ( #25202, #11705 ), #7661, .T. ) ;
#14449=CARTESIAN_POINT ( 'NONE',  ( 2.000000000000000888, 26.72500000000000142, 12.46410161513774817 ) ) ;
#14453=CARTESIAN_POINT ( 'NONE',  ( 1.878215178125000939, 26.86562499938548498, 12.25316411605952283 ) ) ;
#14455=CARTESIAN_POINT ( 'NONE',  ( 21.58443449571939965, 18.75600737097314052, 12.46410161513774817 ) ) ;
#14457=CARTESIAN_POINT ( 'NONE',  ( -1.057460391440397258E-14, 29.10624999877096641, 4.999999999999992006 ) ) ;
#14458=CARTESIAN_POINT ( 'NONE',  ( -3.756430356250003211, -26.07812499938548356, 6.831223922626973533 ) ) ;
#14462=CARTESIAN_POINT ( 'NONE',  ( 3.999999999999997335, -27.96250000000000213, 11.30940107675849404 ) ) ;
#14465=ORIENTED_EDGE ( 'NONE', *, *, #12347, .F. ) ;
#14468=EDGE_LOOP ( 'NONE', ( #1599, #24548, #25720, #20894, #4786, #4118 ) ) ;
#14471=CARTESIAN_POINT ( 'NONE',  ( -1.878215178125004048, -26.67812499938548498, 5.746835883940462963 ) ) ;
#14473=CARTESIAN_POINT ( 'NONE',  ( 19.30843454290614147, 19.30843454290607752, 4.999999999999991118 ) ) ;
#14474=EDGE_CURVE ( 'NONE', #8943, #3881, #17230, .T. ) ;
#14481=CARTESIAN_POINT ( 'NONE',  ( 19.28854716511979461, 19.28854716511973066, 13.33755215474602984 ) ) ;
#14482=CARTESIAN_POINT ( 'NONE',  ( 19.14933551713916771, 19.14933551713910020, 13.61880215351699874 ) ) ;
#14484=CARTESIAN_POINT ( 'NONE',  ( 22.22083059878729117, 19.39240347404102849, 12.46410161513774817 ) ) ;
#14486=LINE ( 'NONE', #14370, #7457 ) ;
#14487=VERTEX_POINT ( 'NONE', #1516 ) ;
#14488=CARTESIAN_POINT ( 'NONE',  ( 20.45982030258741702, 15.14742554666860563, 6.831223922626973533 ) ) ;
#14489=DIRECTION ( 'NONE',  ( 0.000000000000000000, 0.000000000000000000, 1.000000000000000000 ) ) ;
#14493=CARTESIAN_POINT ( 'NONE',  ( -3.735045420075836212E-15, -26.60312499938547859, 4.662447845253954171 ) ) ;
#14499=CARTESIAN_POINT ( 'NONE',  ( -3.756430356250003655, -29.75312499938548783, 8.999999999999992895 ) ) ;
#14503=EDGE_CURVE ( 'NONE', #990, #6938, #4702, .T. ) ;
#14504=DIRECTION ( 'NONE',  ( 0.000000000000000000, 1.000000000000000000, 0.000000000000000000 ) ) ;
#14507=CARTESIAN_POINT ( 'NONE',  ( 3.756430356250004099, 25.17812499938548498, 6.831223922626973533 ) ) ;
#14515=CARTESIAN_POINT ( 'NONE',  ( 1.878215178124998497, -26.90312499938548285, 12.25316411605951927 ) ) ;
#14519=DIRECTION ( 'NONE',  ( 0.000000000000000000, 1.000000000000000000, 0.000000000000000000 ) ) ;
#14522=FACE_OUTER_BOUND ( 'NONE', #14137, .T. ) ;
#14525=EDGE_LOOP ( 'NONE', ( #6359, #4457, #6424, #994 ) ) ;
#14528=VERTEX_POINT ( 'NONE', #23348 ) ;
#14532=CARTESIAN_POINT ( 'NONE',  ( 3.735045420075836212E-15, 28.51562499938548356, 4.662447845253954171 ) ) ;
#14536=CARTESIAN_POINT ( 'NONE',  ( 16.57931677857143882, 21.89171153449011697, 11.16877607737301226 ) ) ;
#14544=CARTESIAN_POINT ( 'NONE',  ( 1.878215178125004048, 28.81562499938548427, 5.746835883940462963 ) ) ;
#14546=CARTESIAN_POINT ( 'NONE',  ( -2.000000000000003997, -28.22500000000000142, 5.535898384862238508 ) ) ;
#14548=ORIENTED_EDGE ( 'NONE', *, *, #12980, .F. ) ;
#14549=ORIENTED_EDGE ( 'NONE', *, *, #5541, .T. ) ;
#14556=CARTESIAN_POINT ( 'NONE',  ( -3.469446951953614189E-15, -30.00000000000000355, 4.999999999999992006 ) ) ;
#14561=DIRECTION ( 'NONE',  ( 1.000000000000000000, 0.000000000000000000, 0.000000000000000000 ) ) ;
#14565=VECTOR ( 'NONE', #5604, 1000.000000000000000 ) ;
#14569=EDGE_CURVE ( 'NONE', #11941, #16614, #7149, .T. ) ;
#14570=CARTESIAN_POINT ( 'NONE',  ( 1.878215178125004048, 27.01562499938548711, 5.746835883940462963 ) ) ;
#14573=CARTESIAN_POINT ( 'NONE',  ( 20.83105136271035462, 15.51865660679153969, 8.999999999999992895 ) ) ;
#14576=CARTESIAN_POINT ( 'NONE',  ( 20.46190248058575634, 20.46190248058568528, 13.61880215351699874 ) ) ;
#14578=CARTESIAN_POINT ( 'NONE',  ( 1.859271017917182139E-15, 29.38749999999999929, 12.99999999999999289 ) ) ;
#14579=CARTESIAN_POINT ( 'NONE',  ( 3.999999999999995559, -27.83124999877096784, 6.690598923241487306 ) ) ;
#14580=CARTESIAN_POINT ( 'NONE',  ( 3.756430356249996994, -26.26562499938548711, 8.999999999999992895 ) ) ;
#14584=CARTESIAN_POINT ( 'NONE',  ( 3.999999999999996003, -28.33750000000000213, 6.690598923241487306 ) ) ;
#14586=ORIENTED_EDGE ( 'NONE', *, *, #9092, .T. ) ;
#14587=ORIENTED_EDGE ( 'NONE', *, *, #12188, .T. ) ;
#14590=VERTEX_POINT ( 'NONE', #9870 ) ;
#14591=CARTESIAN_POINT ( 'NONE',  ( 3.756430356249997438, -25.96562499938548640, 11.16877607737301048 ) ) ;
#14594=AXIS2_PLACEMENT_3D ( 'NONE', #24024, #11734, #14087 ) ;
#14605=LINE ( 'NONE', #18401, #14677 ) ;
#14608=CARTESIAN_POINT ( 'NONE',  ( 22.31597560320210505, 17.00358084728328478, 11.16877607737301226 ) ) ;
#14609=CARTESIAN_POINT ( 'NONE',  ( 23.33010436090463102, 17.67325011141217317, 8.999999999999992895 ) ) ;
#14611=CARTESIAN_POINT ( 'NONE',  ( -3.999999999999997335, 28.41250000000000142, 11.30940107675849404 ) ) ;
#14622=CARTESIAN_POINT ( 'NONE',  ( 2.000000000000003997, 28.16874999877096997, 5.535898384862238508 ) ) ;
#14623=CARTESIAN_POINT ( 'NONE',  ( 3.756430356249995661, -27.57812499938548356, 6.831223922626973533 ) ) ;
#14625=ORIENTED_EDGE ( 'NONE', *, *, #12468, .T. ) ;
#14627=VECTOR ( 'NONE', #15858, 1000.000000000000000 ) ;
#14629=CARTESIAN_POINT ( 'NONE',  ( 1.878215178124995832, -25.74062499938548498, 5.746835883940462963 ) ) ;
#14630=ORIENTED_EDGE ( 'NONE', *, *, #25697, .T. ) ;
#14641=CARTESIAN_POINT ( 'NONE',  ( -3.756430356249997882, 29.56562499938549138, 11.16877607737301226 ) ) ;
#14647=CARTESIAN_POINT ( 'NONE',  ( -1.071796769724488563, 28.86115380933863506, 12.99999999999999289 ) ) ;
#14648=CARTESIAN_POINT ( 'NONE',  ( -2.672651547586948120E-15, -26.49062499938548143, 13.33755215474602984 ) ) ;
#14650=EDGE_CURVE ( 'NONE', #19628, #9493, #13940, .T. ) ;
#14653=CARTESIAN_POINT ( 'NONE',  ( 3.999999999999996447, -25.22500000000000142, 8.999999999999992895 ) ) ;
#14654=CARTESIAN_POINT ( 'NONE',  ( -3.999999999999995559, 27.88750000000000284, 6.690598923241487306 ) ) ;
#14669=CARTESIAN_POINT ( 'NONE',  ( 1.878215178125004048, 29.37812499938548783, 5.746835883940462963 ) ) ;
#14677=VECTOR ( 'NONE', #14362, 1000.000000000000000 ) ;
#14678=CARTESIAN_POINT ( 'NONE',  ( 11.52193136556785369, -23.36965697125208052, 20.00001199999999457 ) ) ;
#14683=EDGE_CURVE ( 'NONE', #18554, #12515, #2028, .T. ) ;
#14695=VERTEX_POINT ( 'NONE', #23997 ) ;
#14697=ORIENTED_EDGE ( 'NONE', *, *, #8703, .F. ) ;
#14698=CARTESIAN_POINT ( 'NONE',  ( -1.878215178125000939, -25.62812499938548783, 12.25316411605952283 ) ) ;
#14700=FACE_OUTER_BOUND ( 'NONE', #9358, .T. ) ;
#14707=AXIS2_PLACEMENT_3D ( 'NONE', #15762, #4248, #17596 ) ;
#14710=CARTESIAN_POINT ( 'NONE',  ( 15.70427213685309020, 21.01666689277176658, 11.16877607737301226 ) ) ;
#14711=CARTESIAN_POINT ( 'NONE',  ( -3.756430356249997882, 29.00312499938548072, 11.16877607737301226 ) ) ;
#14712=VECTOR ( 'NONE', #8889, 1000.000000000000000 ) ;
#14716=CARTESIAN_POINT ( 'NONE',  ( 23.68807716974937705, 18.03122292025692275, 8.999999999999992895 ) ) ;
#14717=VECTOR ( 'NONE', #863, 1000.000000000000000 ) ;
#14720=AXIS2_PLACEMENT_3D ( 'NONE', #11873, #21943, #8088 ) ;
#14721=CARTESIAN_POINT ( 'NONE',  ( -3.756430356250003211, -27.87812499938548427, 6.831223922626973533 ) ) ;
#14732=ORIENTED_EDGE ( 'NONE', *, *, #20906, .T. ) ;
#14733=CARTESIAN_POINT ( 'NONE',  ( -3.756430356250002323, -25.66562499938548569, 11.16877607737301403 ) ) ;
#14739=CARTESIAN_POINT ( 'NONE',  ( 21.32489136114433848, 19.80914183329221956, 4.999999999999988454 ) ) ;
#14741=DIRECTION ( 'NONE',  ( 0.000000000000000000, -1.000000000000000000, 0.000000000000000000 ) ) ;
#14745=CARTESIAN_POINT ( 'NONE',  ( 19.12944813935283150, 19.12944813935275334, 4.662447845253954171 ) ) ;
#14747=CARTESIAN_POINT ( 'NONE',  ( 20.83105136271035462, 15.51865660679153969, 8.999999999999992895 ) ) ;
#14749=CARTESIAN_POINT ( 'NONE',  ( 20.46970022635141362, 14.98507572364578699, 8.999999999999992895 ) ) ;
#14752=DIRECTION ( 'NONE',  ( 0.000000000000000000, 0.000000000000000000, 1.000000000000000000 ) ) ;
#14753=CARTESIAN_POINT ( 'NONE',  ( 21.04318339706631846, 15.73078864114750530, 11.16877607737301403 ) ) ;
#14754=CARTESIAN_POINT ( 'NONE',  ( -27.10000000000000497, 0.6000000000000000888, 19.59999999999999787 ) ) ;
#14757=CARTESIAN_POINT ( 'NONE',  ( 4.000000000000001776, 28.95624999877097494, 11.30940107675849760 ) ) ;
#14758=CARTESIAN_POINT ( 'NONE',  ( -3.756430356250003655, -26.04062499938548569, 8.999999999999992895 ) ) ;
#14761=DIRECTION ( 'NONE',  ( -1.000000000000000000, 0.000000000000000000, -0.000000000000000000 ) ) ;
#14762=ADVANCED_FACE ( 'NONE', ( #9014 ), #10972, .F. ) ;
#14765=CARTESIAN_POINT ( 'NONE',  ( -3.735045420075836212E-15, -25.25312499938548783, 4.662447845253954171 ) ) ;
#14772=EDGE_CURVE ( 'NONE', #21476, #16682, #8773, .T. ) ;
#14775=CARTESIAN_POINT ( 'NONE',  ( -26.00000000000000355, 0.000000000000000000, 20.00001200000000168 ) ) ;
#14776=CARTESIAN_POINT ( 'NONE',  ( -3.756430356249996994, 28.06562499938548427, 8.999999999999992895 ) ) ;
#14777=EDGE_CURVE ( 'NONE', #23711, #5606, #24644, .T. ) ;
#14780=DIRECTION ( 'NONE',  ( -0.7071067811865487940, -0.7071067811865463515, 0.000000000000000000 ) ) ;
#14781=CARTESIAN_POINT ( 'NONE',  ( 18.23893553636149534, 21.06736266110760880, 5.535898384862237620 ) ) ;
#14783=CARTESIAN_POINT ( 'NONE',  ( 1.057460391440397258E-14, -29.10624999877096641, 4.999999999999992006 ) ) ;
#14784=CARTESIAN_POINT ( 'NONE',  ( -3.756430356250004099, -26.64062499938549067, 6.831223922626973533 ) ) ;
#14803=CARTESIAN_POINT ( 'NONE',  ( 3.735045420075836212E-15, 28.96562499938548640, 4.662447845253954171 ) ) ;
#14807=CARTESIAN_POINT ( 'NONE',  ( 20.87953742278953229, 20.87953742278945768, 13.33755215474602984 ) ) ;
#14808=EDGE_CURVE ( 'NONE', #5938, #23065, #14816, .T. ) ;
#14809=CARTESIAN_POINT ( 'NONE',  ( -3.756430356249995661, 26.34062499938548285, 6.831223922626973533 ) ) ;
#14810=CARTESIAN_POINT ( 'NONE',  ( 20.30280345481879323, 20.30280345481869730, 4.999999999999992006 ) ) ;
#14816=( BOUNDED_CURVE ( )  B_SPLINE_CURVE ( 2, ( #13463, #3897, #21430, #25730, #15411, #3511, #19196, #11482, #17637 ),
 .UNSPECIFIED., .F., .F. ) 
 B_SPLINE_CURVE_WITH_KNOTS ( ( 3, 2, 2, 2, 3 ),
 ( 0.7750000000000000222, 0.7833333333333333259, 0.8000000000000000444, 0.8166666666666666519, 0.8250000000000000666 ),
 .UNSPECIFIED. ) 
 CURVE ( )  GEOMETRIC_REPRESENTATION_ITEM ( )  RATIONAL_B_SPLINE_CURVE ( ( 0.9330127018922194093, 0.9330127018922194093, 1.000000000000000000, 0.8660254037844387076, 1.000000000000000000, 0.8660254037844387076, 1.000000000000000000, 0.9330127018922189652, 0.9330127018922194093 ) ) 
 REPRESENTATION_ITEM ( '' )  );
#14818=CARTESIAN_POINT ( 'NONE',  ( 1.071796769724490117, -26.48259618943233562, 4.999999999999992895 ) ) ;
#14822=VERTEX_POINT ( 'NONE', #23763 ) ;
#14824=EDGE_LOOP ( 'NONE', ( #11994, #10649, #18843, #12950 ) ) ;
#14831=ORIENTED_EDGE ( 'NONE', *, *, #14650, .F. ) ;
#14834=CARTESIAN_POINT ( 'NONE',  ( 1.999999999999998224, -27.55000000000000071, 12.46410161513774639 ) ) ;
#14838=CARTESIAN_POINT ( 'NONE',  ( 21.78564551731219723, 16.47325076139337696, 8.999999999999992895 ) ) ;
#14840=CARTESIAN_POINT ( 'NONE',  ( -1.878215178124998497, 28.14062499938548356, 12.25316411605951927 ) ) ;
#14847=CARTESIAN_POINT ( 'NONE',  ( 3.756430356249997438, -26.75312499938548427, 11.16877607737301048 ) ) ;
#14857=ORIENTED_EDGE ( 'NONE', *, *, #16431, .T. ) ;
#14858=CARTESIAN_POINT ( 'NONE',  ( 3.756430356249996105, -29.49062499938548498, 6.831223922626973533 ) ) ;
#14859=CARTESIAN_POINT ( 'NONE',  ( 4.000000000000003553, 25.90000000000000213, 8.999999999999992895 ) ) ;
#14867=CARTESIAN_POINT ( 'NONE',  ( 18.06657825931632999, 20.89500538406245056, 12.46410161513774639 ) ) ;
#14871=CARTESIAN_POINT ( 'NONE',  ( 17.50739442887878639, 22.81978918479745744, 8.999999999999992895 ) ) ;
#14872=CARTESIAN_POINT ( 'NONE',  ( 16.28763523133199342, 21.60002998725066448, 6.831223922626973533 ) ) ;
#14877=CARTESIAN_POINT ( 'NONE',  ( 16.66113976570983368, 19.31733714366914256, 12.25316411605951927 ) ) ;
#14881=CARTESIAN_POINT ( 'NONE',  ( -3.999999999999996003, 28.73124999877096641, 6.690598923241487306 ) ) ;
#14882=CARTESIAN_POINT ( 'NONE',  ( 3.999999999999996003, -25.18750000000000000, 6.690598923241487306 ) ) ;
#14887=CARTESIAN_POINT ( 'NONE',  ( 3.756430356249997882, -29.00312499938548072, 11.16877607737301226 ) ) ;
#14889=ORIENTED_EDGE ( 'NONE', *, *, #15570, .F. ) ;
#14892=CARTESIAN_POINT ( 'NONE',  ( -8.000000000000000000, 10.00000000000000178, 15.00000000000000178 ) ) ;
#14896=CARTESIAN_POINT ( 'NONE',  ( -2.000000000000000888, -27.11874999877096926, 12.46410161513774817 ) ) ;
#14897=CARTESIAN_POINT ( 'NONE',  ( -3.756430356249997882, 28.55312499938548498, 11.16877607737301226 ) ) ;
#14908=CARTESIAN_POINT ( 'NONE',  ( 18.03564233677035489, 18.03564233677029094, 4.999999999999992006 ) ) ;
#14909=CARTESIAN_POINT ( 'NONE',  ( 1.878215178124998497, -27.35312499938548569, 12.25316411605951927 ) ) ;
#14910=CARTESIAN_POINT ( 'NONE',  ( 19.94483064597403654, 19.94483064597395838, 4.999999999999992006 ) ) ;
#14925=CARTESIAN_POINT ( 'NONE',  ( 0.000000000000000000, 0.000000000000000000, 19.00000000000000000 ) ) ;
#14928=CARTESIAN_POINT ( 'NONE',  ( 17.79907597611823533, 23.11147073203690283, 6.831223922626973533 ) ) ;
#14929=CARTESIAN_POINT ( 'NONE',  ( -1.878215178124995832, 25.85312499938548569, 5.746835883940462963 ) ) ;
#14930=EDGE_CURVE ( 'NONE', #939, #8636, #4265, .T. ) ;
#14936=CARTESIAN_POINT ( 'NONE',  ( 19.65004280752532395, 21.16579233537729721, 12.99999999999999289 ) ) ;
#14939=CARTESIAN_POINT ( 'NONE',  ( -4.000000000000001776, -25.41250000000000142, 11.30940107675849760 ) ) ;
#14940=ORIENTED_EDGE ( 'NONE', *, *, #9124, .T. ) ;
#14946=ORIENTED_EDGE ( 'NONE', *, *, #2288, .F. ) ;
#14952=( BOUNDED_CURVE ( )  B_SPLINE_CURVE ( 2, ( #14908, #23015, #2517, #18829, #5099, #2269, #22133, #24847, #440 ),
 .UNSPECIFIED., .F., .F. ) 
 B_SPLINE_CURVE_WITH_KNOTS ( ( 3, 2, 2, 2, 3 ),
 ( 0.02500000000000001180, 0.03333333333333333287, 0.05000000000000000278, 0.06666666666666666574, 0.07500000000000002498 ),
 .UNSPECIFIED. ) 
 CURVE ( )  GEOMETRIC_REPRESENTATION_ITEM ( )  RATIONAL_B_SPLINE_CURVE ( ( 0.9330127018922192983, 0.9330127018922194093, 1.000000000000000000, 0.8660254037844387076, 1.000000000000000000, 0.8660254037844387076, 1.000000000000000000, 0.9330127018922191873, 0.9330127018922192983 ) ) 
 REPRESENTATION_ITEM ( '' )  );
#14958=CARTESIAN_POINT ( 'NONE',  ( 20.80453485841585959, 15.49214010249704643, 11.16877607737301226 ) ) ;
#14959=( BOUNDED_CURVE ( )  B_SPLINE_CURVE ( 2, ( #20893, #2980, #25075, #12791, #18802, #23237, #6774, #20763, #10949 ),
 .UNSPECIFIED., .F., .F. ) 
 B_SPLINE_CURVE_WITH_KNOTS ( ( 3, 2, 2, 2, 3 ),
 ( 0.02500000000000000139, 0.03333333333333333287, 0.05000000000000000278, 0.06666666666666666574, 0.07500000000000001110 ),
 .UNSPECIFIED. ) 
 CURVE ( )  GEOMETRIC_REPRESENTATION_ITEM ( )  RATIONAL_B_SPLINE_CURVE ( ( 0.9330127018922194093, 0.9330127018922194093, 1.000000000000000000, 0.8660254037844387076, 1.000000000000000000, 0.8660254037844387076, 1.000000000000000000, 0.9330127018922191873, 0.9330127018922192983 ) ) 
 REPRESENTATION_ITEM ( '' )  );
#14961=CARTESIAN_POINT ( 'NONE',  ( -1.999999999999998224, 25.75000000000000355, 12.46410161513774639 ) ) ;
#14962=CARTESIAN_POINT ( 'NONE',  ( 21.14697593998939595, 18.49077856202994852, 5.746835883940462963 ) ) ;
#14963=DIRECTION ( 'NONE',  ( 0.000000000000000000, 0.000000000000000000, -1.000000000000000000 ) ) ;
#14965=EDGE_LOOP ( 'NONE', ( #3172, #7679, #13397, #11258, #13126, #1057, #13184, #3218 ) ) ;
#14967=CARTESIAN_POINT ( 'NONE',  ( 3.756430356249997438, -26.30312499938548854, 11.16877607737301048 ) ) ;
#14972=LINE ( 'NONE', #22950, #15049 ) ;
#14977=AXIS2_PLACEMENT_3D ( 'NONE', #5386, #15466, #7739 ) ;
#14982=CARTESIAN_POINT ( 'NONE',  ( 2.000000000000003997, 25.97500000000000142, 5.535898384862238508 ) ) ;
#14993=CARTESIAN_POINT ( 'NONE',  ( 3.756430356250003211, 26.52812499938548285, 6.831223922626973533 ) ) ;
#14996=CARTESIAN_POINT ( 'NONE',  ( 23.29708626209844269, 17.98469150617961887, 8.999999999999992895 ) ) ;
#14997=CARTESIAN_POINT ( 'NONE',  ( 16.95282131294928263, 19.60901869090858796, 5.746835883940462963 ) ) ;
#14998=EDGE_CURVE ( 'NONE', #21622, #21212, #7627, .T. ) ;
#14999=CARTESIAN_POINT ( 'NONE',  ( 23.68807716974937705, 18.03122292025692275, 8.999999999999992895 ) ) ;
#15001=CARTESIAN_POINT ( 'NONE',  ( 23.72661691079926527, 18.35913567140812575, 7.710170883190207824 ) ) ;
#15002=CARTESIAN_POINT ( 'NONE',  ( 22.63417365473605614, 17.32177889881723587, 11.16877607737301403 ) ) ;
#15003=CARTESIAN_POINT ( 'NONE',  ( 22.18105584147648912, 19.35262871673023000, 12.46410161513774817 ) ) ;
#15004=EDGE_LOOP ( 'NONE', ( #16982, #17310, #5000, #10110 ) ) ;
#15006=CARTESIAN_POINT ( 'NONE',  ( 4.000000000000003553, 29.03124999877096712, 6.690598923241489970 ) ) ;
#15007=CARTESIAN_POINT ( 'NONE',  ( -3.756430356250002323, -29.60312499938548569, 11.16877607737301226 ) ) ;
#15014=CARTESIAN_POINT ( 'NONE',  ( -3.756430356250004099, -28.32812499938548356, 6.831223922626973533 ) ) ;
#15017=CARTESIAN_POINT ( 'NONE',  ( 19.26088974974303625, 23.00113871462370341, 5.987824696368042154 ) ) ;
#15019=EDGE_CURVE ( 'NONE', #16342, #23081, #15961, .T. ) ;
#15027=CARTESIAN_POINT ( 'NONE',  ( -3.756430356249997882, 29.00312499938548072, 11.16877607737301226 ) ) ;
#15028=CARTESIAN_POINT ( 'NONE',  ( 20.53261315870440384, 14.87575890921195665, 6.690598923241489970 ) ) ;
#15030=CARTESIAN_POINT ( 'NONE',  ( 3.469446951953614189E-15, 30.00000000000000355, 8.999999999999992895 ) ) ;
#15035=LINE ( 'NONE', #12447, #14298 ) ;
#15036=CARTESIAN_POINT ( 'NONE',  ( 1.878215178124995832, -26.30312499938548498, 5.746835883940462963 ) ) ;
#15041=CARTESIAN_POINT ( 'NONE',  ( -3.999999999999997335, 26.10624999877096997, 11.30940107675849404 ) ) ;
#15048=ORIENTED_EDGE ( 'NONE', *, *, #3089, .F. ) ;
#15049=VECTOR ( 'NONE', #5288, 1000.000000000000000 ) ;
#15054=AXIS2_PLACEMENT_3D ( 'NONE', #7844, #15829, #3542 ) ;
#15056=EDGE_CURVE ( 'NONE', #11588, #19628, #15103, .T. ) ;
#15058=EDGE_LOOP ( 'NONE', ( #19945, #9910, #8352, #1885, #1564 ) ) ;
#15059=EDGE_CURVE ( 'NONE', #11742, #7537, #5027, .T. ) ;
#15060=CARTESIAN_POINT ( 'NONE',  ( 3.735045420075836212E-15, 29.41562499938548569, 4.662447845253954171 ) ) ;
#15064=CARTESIAN_POINT ( 'NONE',  ( 22.66069015903055117, 17.34829540311172735, 8.999999999999992895 ) ) ;
#15065=EDGE_CURVE ( 'NONE', #16682, #16342, #3067, .T. ) ;
#15066=CARTESIAN_POINT ( 'NONE',  ( 3.756430356250004099, 25.29062499938548569, 6.831223922626973533 ) ) ;
#15067=CARTESIAN_POINT ( 'NONE',  ( -19.58805710660146104, -17.18149551509901940, 20.00001200000000168 ) ) ;
#15071=LINE ( 'NONE', #7342, #23314 ) ;
#15083=CARTESIAN_POINT ( 'NONE',  ( 3.756430356249997882, -26.41562499938548569, 11.16877607737301226 ) ) ;
#15084=ORIENTED_EDGE ( 'NONE', *, *, #11177, .T. ) ;
#15085=DIRECTION ( 'NONE',  ( 0.000000000000000000, -1.000000000000000000, 0.000000000000000000 ) ) ;
#15091=CARTESIAN_POINT ( 'NONE',  ( -1.626862140677534194E-14, -27.58750000000000213, 12.99999999999999289 ) ) ;
#15096=CARTESIAN_POINT ( 'NONE',  ( 21.75912901301770219, 16.44673425709888548, 11.16877607737301226 ) ) ;
#15101=CARTESIAN_POINT ( 'NONE',  ( 2.000000000000000888, 26.27499999999999858, 12.46410161513774817 ) ) ;
#15102=CARTESIAN_POINT ( 'NONE',  ( 18.01348148472910893, 20.66967886268841426, 12.25316411605951927 ) ) ;
#15103=LINE ( 'NONE', #7370, #24122 ) ;
#15108=VECTOR ( 'NONE', #17772, 1000.000000000000000 ) ;
#15109=CARTESIAN_POINT ( 'NONE',  ( 3.756430356249996994, -28.51562499938548356, 8.999999999999992895 ) ) ;
#15115=ORIENTED_EDGE ( 'NONE', *, *, #7428, .T. ) ;
#15117=( BOUNDED_CURVE ( )  B_SPLINE_CURVE ( 2, ( #1163, #5480, #13474, #21440, #24969, #3520, #23527, #19465, #1556 ),
 .UNSPECIFIED., .F., .F. ) 
 B_SPLINE_CURVE_WITH_KNOTS ( ( 3, 2, 2, 2, 3 ),
 ( 0.4750000000000000333, 0.4833333333333333370, 0.5000000000000000000, 0.5166666666666667185, 0.5250000000000000222 ),
 .UNSPECIFIED. ) 
 CURVE ( )  GEOMETRIC_REPRESENTATION_ITEM ( )  RATIONAL_B_SPLINE_CURVE ( ( 0.9330127018922194093, 0.9330127018922196314, 1.000000000000000000, 0.8660254037844387076, 1.000000000000000000, 0.8660254037844387076, 1.000000000000000000, 0.9330127018922194093, 0.9330127018922194093 ) ) 
 REPRESENTATION_ITEM ( '' )  );
#15122=CARTESIAN_POINT ( 'NONE',  ( -3.756430356250002323, -28.36562499938548854, 11.16877607737301403 ) ) ;
#15137=DIRECTION ( 'NONE',  ( -1.000000000000000000, -0.000000000000000000, -0.000000000000000000 ) ) ;
#15138=CARTESIAN_POINT ( 'NONE',  ( -3.756430356249996105, 27.12812499938548427, 6.831223922626973533 ) ) ;
#15139=CARTESIAN_POINT ( 'NONE',  ( 3.469446951953614189E-15, 30.00000000000000355, 4.999999999999992006 ) ) ;
#15140=CARTESIAN_POINT ( 'NONE',  ( 15.32653948221845575, 20.98339373171076971, 8.999999999999992895 ) ) ;
#15141=CARTESIAN_POINT ( 'NONE',  ( 21.49396397007274473, 16.18156921415393157, 6.831223922626973533 ) ) ;
#15142=DIRECTION ( 'NONE',  ( -0.7071067811865487940, -0.7071067811865463515, 0.000000000000000000 ) ) ;
#15145=VECTOR ( 'NONE', #7328, 1000.000000000000000 ) ;
#15146=CARTESIAN_POINT ( 'NONE',  ( 16.89751483010538990, 22.20990958602406096, 11.16877607737301048 ) ) ;
#15150=CARTESIAN_POINT ( 'NONE',  ( 4.000000000000003553, 28.99374999877096926, 8.999999999999992895 ) ) ;
#15151=CARTESIAN_POINT ( 'NONE',  ( -3.756430356250004099, -29.22812499938548925, 6.831223922626973533 ) ) ;
#15152=CARTESIAN_POINT ( 'NONE',  ( -1.859271017917182139E-15, -29.38749999999999929, 12.99999999999999289 ) ) ;
#15157=CARTESIAN_POINT ( 'NONE',  ( 1.878215178124995832, -29.34062499938548285, 5.746835883940462963 ) ) ;
#15160=CARTESIAN_POINT ( 'NONE',  ( 21.02850174869167788, 21.39790512250117871, 12.99999999999999467 ) ) ;
#15163=ADVANCED_FACE ( 'NONE', ( #1225 ), #20990, .F. ) ;
#15175=CARTESIAN_POINT ( 'NONE',  ( -1.878215178125000939, -29.22812499938548569, 12.25316411605952283 ) ) ;
#15176=CARTESIAN_POINT ( 'NONE',  ( 19.20116603387162613, 20.71691556172359938, 4.999999999999992006 ) ) ;
#15179=DIRECTION ( 'NONE',  ( 1.000000000000000000, -0.000000000000000000, 0.000000000000000000 ) ) ;
#15180=CARTESIAN_POINT ( 'NONE',  ( 20.14370442905180525, 20.14370442905174130, 12.99999999999999289 ) ) ;
#15184=VERTEX_POINT ( 'NONE', #7119 ) ;
#15189=FACE_OUTER_BOUND ( 'NONE', #14468, .T. ) ;
#15190=DIRECTION ( 'NONE',  ( 0.000000000000000000, 0.000000000000000000, -1.000000000000000000 ) ) ;
#15194=CARTESIAN_POINT ( 'NONE',  ( 18.14379053194667790, 23.45618528786534895, 8.999999999999992895 ) ) ;
#15195=CARTESIAN_POINT ( 'NONE',  ( 1.878215178125004048, 26.67812499938548498, 5.746835883940462963 ) ) ;
#15198=CARTESIAN_POINT ( 'NONE',  ( 18.17706369300767832, 23.83391794249997631, 11.30940107675849404 ) ) ;
#15204=CARTESIAN_POINT ( 'NONE',  ( -4.000000000000003553, -25.43124999877096926, 6.690598923241489970 ) ) ;
#15213=FACE_OUTER_BOUND ( 'NONE', #23178, .T. ) ;
#15215=CARTESIAN_POINT ( 'NONE',  ( -3.756430356250004099, -26.19062499938548783, 6.831223922626973533 ) ) ;
#15223=EDGE_CURVE ( 'NONE', #15567, #13481, #7834, .T. ) ;
#15224=CARTESIAN_POINT ( 'NONE',  ( 16.34066823992098350, 21.65306299583965455, 11.16877607737301226 ) ) ;
#15227=CARTESIAN_POINT ( 'NONE',  ( -3.999999999999996447, 26.57500000000000284, 8.999999999999992895 ) ) ;
#15229=CARTESIAN_POINT ( 'NONE',  ( 20.51057983692150444, 17.85438245896205700, 5.746835883940462963 ) ) ;
#15235=CARTESIAN_POINT ( 'NONE',  ( 1.878215178124998497, -29.04062499938548569, 12.25316411605951927 ) ) ;
#15246=CARTESIAN_POINT ( 'NONE',  ( -1.878215178125004048, -28.47812499938548569, 5.746835883940462963 ) ) ;
#15247=CARTESIAN_POINT ( 'NONE',  ( 3.834746474454188013E-15, 26.01249999999999574, 4.999999999999992006 ) ) ;
#15249=LINE ( 'NONE', #13547, #22298 ) ;
#15254=DIRECTION ( 'NONE',  ( 0.000000000000000000, -1.000000000000000000, 0.000000000000000000 ) ) ;
#15255=CARTESIAN_POINT ( 'NONE',  ( 3.756430356250002323, 26.90312499938548285, 11.16877607737301403 ) ) ;
#15258=CARTESIAN_POINT ( 'NONE',  ( 21.16900926177230247, 15.51215501227985172, 6.690598923241489970 ) ) ;
#15259=CARTESIAN_POINT ( 'NONE',  ( 18.57260154916842154, 18.57260154916834693, 4.662447845253954171 ) ) ;
#15262=CARTESIAN_POINT ( 'NONE',  ( 21.40018120162940818, 21.02622566956345196, 4.999999999999992006 ) ) ;
#15263=CARTESIAN_POINT ( 'NONE',  ( 20.08404229395467055, 20.08404229395459240, 4.662447845253954171 ) ) ;
#15264=CARTESIAN_POINT ( 'NONE',  ( 22.69370825783673951, 17.03685400834428521, 8.999999999999992895 ) ) ;
#15266=CARTESIAN_POINT ( 'NONE',  ( 20.09951025522764922, 17.27108313048138655, 5.535898384862238508 ) ) ;
#15267=CARTESIAN_POINT ( 'NONE',  ( 1.878215178125000939, 26.52812499938548285, 12.25316411605952283 ) ) ;
#15268=CARTESIAN_POINT ( 'NONE',  ( -2.672651547586948120E-15, -28.62812499938548783, 13.33755215474602984 ) ) ;
#15276=CARTESIAN_POINT ( 'NONE',  ( -1.878215178125004048, -27.91562499938548569, 5.746835883940462963 ) ) ;
#15278=EDGE_LOOP ( 'NONE', ( #19851, #25781, #12307, #22215 ) ) ;
#15279=CARTESIAN_POINT ( 'NONE',  ( 18.97414603143021594, 23.23826331710101556, 11.64163568064553544 ) ) ;
#15286=CARTESIAN_POINT ( 'NONE',  ( -0.2902671272941750868, -30.00000000000000355, 12.99999999999999112 ) ) ;
#15287=CARTESIAN_POINT ( 'NONE',  ( -1.071796769724490117, 26.87634618820330701, 4.999999999999992895 ) ) ;
#15290=CARTESIAN_POINT ( 'NONE',  ( -1.071796769724494558, -27.73615380933863861, 4.999999999999992895 ) ) ;
#15291=CARTESIAN_POINT ( 'NONE',  ( 1.878215178124998497, -28.25312499938548427, 12.25316411605951927 ) ) ;
#15295=EDGE_CURVE ( 'NONE', #14528, #25775, #23454, .T. ) ;
#15303=EDGE_CURVE ( 'NONE', #6479, #10501, #4099, .T. ) ;
#15307=ORIENTED_EDGE ( 'NONE', *, *, #16907, .T. ) ;
#15310=CARTESIAN_POINT ( 'NONE',  ( 23.44808782266543901, 18.71365202105081949, 11.20140010723572566 ) ) ;
#15314=CARTESIAN_POINT ( 'NONE',  ( -3.756430356249996994, 25.92812499938548498, 8.999999999999992895 ) ) ;
#15321=CARTESIAN_POINT ( 'NONE',  ( -2.000000000000003997, -26.81874999877096855, 5.535898384862238508 ) ) ;
#15322=CARTESIAN_POINT ( 'NONE',  ( 21.21320343559646915, 21.21320343559638744, 8.999999999999992895 ) ) ;
#15330=ORIENTED_EDGE ( 'NONE', *, *, #21604, .F. ) ;
#15332=ORIENTED_EDGE ( 'NONE', *, *, #6840, .T. ) ;
#15333=CARTESIAN_POINT ( 'NONE',  ( -2.672651547586948120E-15, -27.84062499938548640, 13.33755215474602984 ) ) ;
#15338=( BOUNDED_CURVE ( )  B_SPLINE_CURVE ( 2, ( #24625, #1216, #6851, #833, #5154, #23069, #14834, #17047, #15091 ),
 .UNSPECIFIED., .F., .F. ) 
 B_SPLINE_CURVE_WITH_KNOTS ( ( 3, 2, 2, 2, 3 ),
 ( 0.5250000000000000222, 0.5333333333333333259, 0.5500000000000000444, 0.5666666666666666519, 0.5750000000000000666 ),
 .UNSPECIFIED. ) 
 CURVE ( )  GEOMETRIC_REPRESENTATION_ITEM ( )  RATIONAL_B_SPLINE_CURVE ( ( 0.9330127018922194093, 0.9330127018922194093, 1.000000000000000000, 0.8660254037844387076, 1.000000000000000000, 0.8660254037844387076, 1.000000000000000000, 0.9330127018922189652, 0.9330127018922194093 ) ) 
 REPRESENTATION_ITEM ( '' )  );
#15343=CARTESIAN_POINT ( 'NONE',  ( 20.72498534553237093, 15.41259058961355954, 11.16877607737301226 ) ) ;
#15345=CARTESIAN_POINT ( 'NONE',  ( -1.999999999999995781, 26.05000000000000071, 5.535898384862237620 ) ) ;
#15346=CARTESIAN_POINT ( 'NONE',  ( 16.97706434298888212, 22.28945909890755317, 11.16877607737301048 ) ) ;
#15349=VERTEX_POINT ( 'NONE', #19900 ) ;
#15360=VECTOR ( 'NONE', #9342, 1000.000000000000000 ) ;
#15363=CARTESIAN_POINT ( 'NONE',  ( 1.878215178124998497, -28.70312499938548356, 12.25316411605951927 ) ) ;
#15372=CARTESIAN_POINT ( 'NONE',  ( -3.137519842735244810E-15, 26.91249999999999787, 4.999999999999991118 ) ) ;
#15375=CARTESIAN_POINT ( 'NONE',  ( -1.878215178124998497, 27.24062499938548498, 12.25316411605951927 ) ) ;
#15376=CARTESIAN_POINT ( 'NONE',  ( -2.645323980344223447, -29.88371542788442881, 5.988343842124890237 ) ) ;
#15377=CARTESIAN_POINT ( 'NONE',  ( 20.72043839702256207, 20.72043839702248036, 4.662447845253954171 ) ) ;
#15378=CARTESIAN_POINT ( 'NONE',  ( 23.08495422774248240, 17.77255947182365503, 6.831223922626973533 ) ) ;
#15379=CARTESIAN_POINT ( 'NONE',  ( 17.70860545047158396, 20.53703257521770453, 12.46410161513774639 ) ) ;
#15380=DIRECTION ( 'NONE',  ( 1.000000000000000000, 0.000000000000000000, -0.000000000000000000 ) ) ;
#15382=CARTESIAN_POINT ( 'NONE',  ( 20.00676625532608455, 17.35056887736664422, 12.25316411605952283 ) ) ;
#15386=CARTESIAN_POINT ( 'NONE',  ( -3.999999999999997335, 29.70624999877097139, 11.30940107675849404 ) ) ;
#15388=CARTESIAN_POINT ( 'NONE',  ( -3.735045420075836212E-15, -29.30312499938548498, 4.662447845253954171 ) ) ;
#15390=ORIENTED_EDGE ( 'NONE', *, *, #7117, .F. ) ;
#15393=CARTESIAN_POINT ( 'NONE',  ( -2.672651547586948120E-15, -28.17812499938548143, 13.33755215474602984 ) ) ;
#15394=VERTEX_POINT ( 'NONE', #14308 ) ;
#15398=AXIS2_PLACEMENT_3D ( 'NONE', #2745, #10707, #9140 ) ;
#15401=ADVANCED_FACE ( 'NONE', ( #22271 ), #815, .F. ) ;
#15411=CARTESIAN_POINT ( 'NONE',  ( 4.000000000000003553, 28.60000000000000142, 8.999999999999992895 ) ) ;
#15412=B_SPLINE_CURVE_WITH_KNOTS ( 'NONE', 3,
 ( #20853, #10908, #1105, #18904, #22703, #16821, #17064, #4783, #12757, #9353 ),
 .UNSPECIFIED., .F., .F.,
 ( 4, 2, 2, 2, 4 ),
 ( 0.01251976117704806969, 0.01338929815772730951, 0.01425883513840654759, 0.01512837211908578741, 0.01599790909976502723 ),
 .UNSPECIFIED. ) ;
#15415=CARTESIAN_POINT ( 'NONE',  ( 15.63147928073609982, 21.28833353022841379, 11.30940107675849404 ) ) ;
#15417=CARTESIAN_POINT ( 'NONE',  ( 1.626862140677534194E-14, 27.58750000000000213, 12.99999999999999289 ) ) ;
#15419=( BOUNDED_CURVE ( )  B_SPLINE_CURVE ( 2, ( #16573, #24532, #2704, #10933, #16317, #10794, #22844, #8712, #10665, #18786, #874, #18656, #16844, #20877, #21018, #15517, #9484, #11318, #11062, #25315, #22972, #5307, #3341, #5434, #23223, #7279, #19163, #23346, #7395, #17086, #19422, #18924, #19040, #25058, #3095, #13039, #13427, #14993, #1515, #25201, #1123, #21399, #19298, #17465, #9098, #23486, #1255, #15255, #25436, #17229, #7520, #1397, #7148, #15138, #9370, #5189, #15375, #13285, #1008, #23107, #5060, #21517, #17351, #3478, #11451, #13167, #21136, #3209, #21261, #11179, #9240, #5572, #13552, #3599, #8985, #16962, #24929, #7008, #6441, #10100, #1641, #18483, #14161, #8407, #2137, #6309, #14304, #22129, #24483, #22268, #20166, #18219, #16523, #7660, #2266, #25574, #14035, #178, #14544, #19539, #437, #12445, #17597, #24090, #572, #16395, #14426, #22387, #4217, #12323, #15643, #4347, #12052, #20032, #6563, #10340, #24222, #20291, #24364, #16253, #301 ),
 .UNSPECIFIED., .F., .F. ) 
 B_SPLINE_CURVE_WITH_KNOTS ( ( 3, 2, 2, 2, 2, 2, 2, 2, 2, 2, 2, 2, 2, 2, 2, 2, 2, 2, 2, 2, 2, 2, 2, 2, 2, 2, 2, 2, 2, 2, 2, 2, 2, 2, 2, 2, 2, 2, 2, 2, 2, 2, 2, 2, 2, 2, 2, 2, 2, 2, 2, 2, 2, 2, 2, 2, 2, 2, 2, 2, 3 ),
 ( 0.000000000000000000, 0.01666666666666666644, 0.03333333333333333287, 0.05000000000000000278, 0.06666666666666666574, 0.08333333333333332871, 0.1000000000000000056, 0.1166666666666666685, 0.1333333333333333315, 0.1499999999999999944, 0.1666666666666666574, 0.1833333333333333204, 0.2000000000000000111, 0.2166666666666666741, 0.2333333333333333370, 0.2500000000000000000, 0.2666666666666666630, 0.2833333333333333259, 0.2999999999999999889, 0.3166666666666666519, 0.3333333333333333148, 0.3499999999999999778, 0.3666666666666666408, 0.3833333333333333592, 0.4000000000000000222, 0.4166666666666666852, 0.4333333333333333481, 0.4500000000000000111, 0.4666666666666666741, 0.4833333333333333370, 0.5000000000000000000, 0.5166666666666667185, 0.5333333333333333259, 0.5500000000000000444, 0.5666666666666666519, 0.5833333333333333703, 0.5999999999999999778, 0.6166666666666666963, 0.6333333333333333037, 0.6500000000000000222, 0.6666666666666666297, 0.6833333333333333481, 0.6999999999999999556, 0.7166666666666666741, 0.7333333333333332815, 0.7500000000000000000, 0.7666666666666667185, 0.7833333333333333259, 0.8000000000000000444, 0.8166666666666666519, 0.8333333333333333703, 0.8499999999999999778, 0.8666666666666666963, 0.8833333333333333037, 0.9000000000000000222, 0.9166666666666666297, 0.9333333333333333481, 0.9499999999999999556, 0.9666666666666666741, 0.9833333333333332815, 1.000000000000000000 ),
 .UNSPECIFIED. ) 
 CURVE ( )  GEOMETRIC_REPRESENTATION_ITEM ( )  RATIONAL_B_SPLINE_CURVE ( ( 1.000000000000000000, 0.8660254037844387076, 1.000000000000000000, 0.8660254037844387076, 1.000000000000000000, 0.8660254037844387076, 1.000000000000000000, 0.8660254037844387076, 1.000000000000000000, 0.8660254037844387076, 1.000000000000000000, 0.8660254037844387076, 1.000000000000000000, 0.8660254037844387076, 1.000000000000000000, 0.8660254037844387076, 1.000000000000000000, 0.8660254037844387076, 1.000000000000000000, 0.8660254037844387076, 1.000000000000000000, 0.8660254037844387076, 1.000000000000000000, 0.8660254037844387076, 1.000000000000000000, 0.8660254037844387076, 1.000000000000000000, 0.8660254037844387076, 1.000000000000000000, 0.8660254037844387076, 1.000000000000000000, 0.8660254037844387076, 1.000000000000000000, 0.8660254037844387076, 1.000000000000000000, 0.8660254037844387076, 1.000000000000000000, 0.8660254037844387076, 1.000000000000000000, 0.8660254037844387076, 1.000000000000000000, 0.8660254037844387076, 1.000000000000000000, 0.8660254037844387076, 1.000000000000000000, 0.8660254037844387076, 1.000000000000000000, 0.8660254037844387076, 1.000000000000000000, 0.8660254037844387076, 1.000000000000000000, 0.8660254037844387076, 1.000000000000000000, 0.8660254037844387076, 1.000000000000000000, 0.8660254037844387076, 1.000000000000000000, 0.8660254037844387076, 1.000000000000000000, 0.8660254037844387076, 1.000000000000000000, 0.8660254037844387076, 1.000000000000000000, 0.8660254037844387076, 1.000000000000000000, 0.8660254037844387076, 1.000000000000000000, 0.8660254037844387076, 1.000000000000000000, 0.8660254037844387076, 1.000000000000000000, 0.8660254037844387076, 1.000000000000000000, 0.8660254037844387076, 1.000000000000000000, 0.8660254037844387076, 1.000000000000000000, 0.8660254037844387076, 1.000000000000000000, 0.8660254037844387076, 1.000000000000000000, 0.8660254037844387076, 1.000000000000000000, 0.8660254037844387076, 1.000000000000000000, 0.8660254037844387076, 1.000000000000000000, 0.8660254037844387076, 1.000000000000000000, 0.8660254037844387076, 1.000000000000000000, 0.8660254037844387076, 1.000000000000000000, 0.8660254037844387076, 1.000000000000000000, 0.8660254037844387076, 1.000000000000000000, 0.8660254037844387076, 1.000000000000000000, 0.8660254037844387076, 1.000000000000000000, 0.8660254037844387076, 1.000000000000000000, 0.8660254037844387076, 1.000000000000000000, 0.8660254037844387076, 1.000000000000000000, 0.8660254037844387076, 1.000000000000000000, 0.8660254037844387076, 1.000000000000000000, 0.8660254037844387076, 1.000000000000000000, 0.8660254037844387076, 1.000000000000000000, 0.8660254037844387076, 1.000000000000000000, 0.8660254037844387076, 1.000000000000000000, 0.8660254037844387076, 1.000000000000000000 ) ) 
 REPRESENTATION_ITEM ( '' )  );
#15421=CARTESIAN_POINT ( 'NONE',  ( 21.16900926177230247, 15.51215501227985172, 6.690598923241489970 ) ) ;
#15423=CARTESIAN_POINT ( 'NONE',  ( -2.000000000000000888, -28.52500000000000213, 12.46410161513774817 ) ) ;
#15430=ORIENTED_EDGE ( 'NONE', *, *, #13633, .F. ) ;
#15434=ORIENTED_EDGE ( 'NONE', *, *, #22318, .T. ) ;
#15443=CARTESIAN_POINT ( 'NONE',  ( 3.756430356250004099, 27.54062499938548569, 6.831223922626973533 ) ) ;
#15454=CARTESIAN_POINT ( 'NONE',  ( 3.999999999999997335, -27.45624999877096784, 11.30940107675849404 ) ) ;
#15460=CARTESIAN_POINT ( 'NONE',  ( -4.000000000000003553, -25.90000000000000213, 8.999999999999992895 ) ) ;
#15466=DIRECTION ( 'NONE',  ( -0.000000000000000000, -0.000000000000000000, 1.000000000000000000 ) ) ;
#15468=CARTESIAN_POINT ( 'NONE',  ( -2.672651547586948120E-15, -26.94062499938548783, 13.33755215474602984 ) ) ;
#15470=CARTESIAN_POINT ( 'NONE',  ( -3.999999999999995559, 28.78750000000000142, 6.690598923241487306 ) ) ;
#15472=EDGE_LOOP ( 'NONE', ( #10265, #18196, #7711, #4064, #2414, #3764, #24199, #22895 ) ) ;
#15477=DIRECTION ( 'NONE',  ( 1.000000000000000000, 0.000000000000000000, 0.000000000000000000 ) ) ;
#15478=CARTESIAN_POINT ( 'NONE',  ( 19.18020767368691182, 21.83640505164621004, 5.746835883940462963 ) ) ;
#15479=EDGE_CURVE ( 'NONE', #25112, #11742, #19304, .T. ) ;
#15483=CARTESIAN_POINT ( 'NONE',  ( -1.999999999999998224, 25.30000000000000426, 12.46410161513774639 ) ) ;
#15486=CARTESIAN_POINT ( 'NONE',  ( 16.60583328286593741, 21.91822803878461912, 6.831223922626973533 ) ) ;
#15491=CARTESIAN_POINT ( 'NONE',  ( -1.878215178125000939, -28.66562499938548569, 12.25316411605952283 ) ) ;
#15492=EDGE_CURVE ( 'NONE', #8456, #16614, #11279, .T. ) ;
#15493=ORIENTED_EDGE ( 'NONE', *, *, #7069, .F. ) ;
#15499=VERTEX_POINT ( 'NONE', #2902 ) ;
#15505=CYLINDRICAL_SURFACE ( 'NONE', #24358, 4.000000000000000000 ) ;
#15512=CARTESIAN_POINT ( 'NONE',  ( -3.756430356249997882, 27.65312499938548640, 11.16877607737301226 ) ) ;
#15517=CARTESIAN_POINT ( 'NONE',  ( 3.735045420075836212E-15, 25.70312499938548001, 4.662447845253954171 ) ) ;
#15520=CARTESIAN_POINT ( 'NONE',  ( 16.91752973988819164, 22.57438398938050028, 8.999999999999992895 ) ) ;
#15521=CARTESIAN_POINT ( 'NONE',  ( 21.67730602587931088, 19.02110864791986344, 12.25316411605952283 ) ) ;
#15526=CARTESIAN_POINT ( 'NONE',  ( 21.06742642710591440, 18.41122904914646341, 5.746835883940462963 ) ) ;
#15527=LINE ( 'NONE', #17607, #3350 ) ;
#15530=CARTESIAN_POINT ( 'NONE',  ( -4.000000000000003553, -26.35000000000000142, 8.999999999999992895 ) ) ;
#15535=CARTESIAN_POINT ( 'NONE',  ( -25.16843286583315731, 6.741346781237202102, 20.00001200000000168 ) ) ;
#15536=CARTESIAN_POINT ( 'NONE',  ( 4.000000000000003553, 26.29374999877096997, 8.999999999999992895 ) ) ;
#15546=CARTESIAN_POINT ( 'NONE',  ( 3.834746474454188013E-15, 26.01249999999999574, 4.999999999999992006 ) ) ;
#15549=CARTESIAN_POINT ( 'NONE',  ( -1.999999999999995781, 26.50000000000000355, 5.535898384862237620 ) ) ;
#15554=CARTESIAN_POINT ( 'NONE',  ( -4.000000000000001776, -27.60624999877096641, 11.30940107675849760 ) ) ;
#15564=CARTESIAN_POINT ( 'NONE',  ( -8.831537335106614961E-15, -26.23749999999999716, 12.99999999999999112 ) ) ;
#15567=VERTEX_POINT ( 'NONE', #24999 ) ;
#15570=EDGE_CURVE ( 'NONE', #24947, #18727, #11012, .T. ) ;
#15571=ORIENTED_EDGE ( 'NONE', *, *, #18920, .F. ) ;
#15573=CARTESIAN_POINT ( 'NONE',  ( -4.000000000000003553, -28.13124999877096855, 6.690598923241489970 ) ) ;
#15575=CARTESIAN_POINT ( 'NONE',  ( 23.85222316637486628, 18.19536891688240487, 9.470295877454905309 ) ) ;
#15579=CARTESIAN_POINT ( 'NONE',  ( -3.369928719974892281E-15, -25.50624999877096855, 4.999999999999992006 ) ) ;
#15581=CARTESIAN_POINT ( 'NONE',  ( 2.672651547586948120E-15, 27.84062499938548640, 13.33755215474602984 ) ) ;
#15588=CARTESIAN_POINT ( 'NONE',  ( 1.999999999999995781, -27.34374999877097068, 5.535898384862237620 ) ) ;
#15589=CARTESIAN_POINT ( 'NONE',  ( 3.756430356250002323, 27.01562499938548356, 11.16877607737301226 ) ) ;
#15598=ORIENTED_EDGE ( 'NONE', *, *, #9244, .F. ) ;
#15599=CARTESIAN_POINT ( 'NONE',  ( 1.878215178124995832, -28.10312499938548569, 5.746835883940462963 ) ) ;
#15602=VERTEX_POINT ( 'NONE', #20818 ) ;
#15603=LINE ( 'NONE', #5652, #1764 ) ;
#15609=FACE_OUTER_BOUND ( 'NONE', #8457, .T. ) ;
#15613=CARTESIAN_POINT ( 'NONE',  ( 22.74023967191403628, 17.42784491599521601, 8.999999999999992895 ) ) ;
#15615=CARTESIAN_POINT ( 'NONE',  ( 2.000000000000003997, 27.77500000000000213, 5.535898384862238508 ) ) ;
#15617=CARTESIAN_POINT ( 'NONE',  ( 21.35910797434536335, 18.70291059638591946, 12.25316411605952283 ) ) ;
#15618=CARTESIAN_POINT ( 'NONE',  ( -4.000000000000003553, -29.48124999877097352, 6.690598923241489970 ) ) ;
#15620=ORIENTED_EDGE ( 'NONE', *, *, #11672, .F. ) ;
#15626=EDGE_CURVE ( 'NONE', #13988, #7895, #6787, .T. ) ;
#15628=CARTESIAN_POINT ( 'NONE',  ( -3.999999999999997335, 27.45624999877096784, 11.30940107675849404 ) ) ;
#15638=CARTESIAN_POINT ( 'NONE',  ( -1.071796769724492338, -26.70759618943233704, 12.99999999999999467 ) ) ;
#15641=CARTESIAN_POINT ( 'NONE',  ( 2.672651547586948120E-15, 26.82812499938548356, 13.33755215474602984 ) ) ;
#15643=CARTESIAN_POINT ( 'NONE',  ( 1.878215178125004048, 29.26562499938548356, 5.746835883940462963 ) ) ;
#15645=CARTESIAN_POINT ( 'NONE',  ( 19.03001124868300309, 19.03001124868292848, 4.381197846482986158 ) ) ;
#15646=CARTESIAN_POINT ( 'NONE',  ( 18.86200962215296784, 21.51820700011226606, 5.746835883940462963 ) ) ;
#15647=CARTESIAN_POINT ( 'NONE',  ( 19.14933551713917126, 19.14933551713910376, 12.99999999999999289 ) ) ;
#15649=DIRECTION ( 'NONE',  ( 0.000000000000000000, 0.000000000000000000, 1.000000000000000000 ) ) ;
#15652=CARTESIAN_POINT ( 'NONE',  ( 17.85210898470722896, 23.16450374062589646, 11.16877607737301048 ) ) ;
#15654=ORIENTED_EDGE ( 'NONE', *, *, #1933, .F. ) ;
#15656=CARTESIAN_POINT ( 'NONE',  ( -4.000000000000001776, -25.86250000000000071, 11.30940107675849760 ) ) ;
#15658=ORIENTED_EDGE ( 'NONE', *, *, #24165, .T. ) ;
#15660=LINE ( 'NONE', #25455, #12594 ) ;
#15661=CARTESIAN_POINT ( 'NONE',  ( 19.58805710660146815, 17.18149551509899453, 20.00001200000000168 ) ) ;
#15663=ORIENTED_EDGE ( 'NONE', *, *, #17656, .T. ) ;
#15670=CARTESIAN_POINT ( 'NONE',  ( -4.000000000000001776, -27.21250000000000213, 11.30940107675849760 ) ) ;
#15673=CARTESIAN_POINT ( 'NONE',  ( -2.205873879792267900, -29.91968208057595646, 12.34935938736416894 ) ) ;
#15675=CARTESIAN_POINT ( 'NONE',  ( 23.85222316637486273, 18.19536891688240843, 8.999999999999992895 ) ) ;
#15676=CARTESIAN_POINT ( 'NONE',  ( 16.24135887950949808, 21.89821312900181027, 8.999999999999992895 ) ) ;
#15678=DIRECTION ( 'NONE',  ( -0.000000000000000000, -0.000000000000000000, 1.000000000000000000 ) ) ;
#15679=CARTESIAN_POINT ( 'NONE',  ( 1.878215178124998497, -28.70312499938548356, 12.25316411605951927 ) ) ;
#15681=CARTESIAN_POINT ( 'NONE',  ( 19.78131220369370169, 16.95288507894744257, 5.535898384862238508 ) ) ;
#15688=ORIENTED_EDGE ( 'NONE', *, *, #17010, .F. ) ;
#15691=ORIENTED_EDGE ( 'NONE', *, *, #7872, .T. ) ;
#15693=ORIENTED_EDGE ( 'NONE', *, *, #15492, .F. ) ;
#15697=CARTESIAN_POINT ( 'NONE',  ( -1.859271017917182139E-15, -29.38749999999999929, 12.99999999999999289 ) ) ;
#15703=DIRECTION ( 'NONE',  ( 0.000000000000000000, 0.000000000000000000, 1.000000000000000000 ) ) ;
#15705=CARTESIAN_POINT ( 'NONE',  ( 1.878215178125000939, 28.32812499938548711, 12.25316411605952283 ) ) ;
#15713=CARTESIAN_POINT ( 'NONE',  ( -4.000000000000001776, -27.15624999877097423, 11.30940107675849760 ) ) ;
#15714=CARTESIAN_POINT ( 'NONE',  ( -3.756430356249997882, 27.31562499938548427, 11.16877607737301226 ) ) ;
#15718=ORIENTED_EDGE ( 'NONE', *, *, #23851, .T. ) ;
#15720=ORIENTED_EDGE ( 'NONE', *, *, #21818, .T. ) ;
#15721=ORIENTED_EDGE ( 'NONE', *, *, #9329, .F. ) ;
#15722=CARTESIAN_POINT ( 'NONE',  ( 0.000000000000000000, 10.00000000000000000, 15.00000000000000178 ) ) ;
#15724=CARTESIAN_POINT ( 'NONE',  ( 3.756430356249995661, -27.69062499938548427, 6.831223922626973533 ) ) ;
#15730=EDGE_CURVE ( 'NONE', #25775, #13483, #2013, .T. ) ;
#15734=CARTESIAN_POINT ( 'NONE',  ( 15.28000806814115720, 20.59240282405983535, 8.999999999999992895 ) ) ;
#15738=CARTESIAN_POINT ( 'NONE',  ( 4.000000000000003553, 28.15000000000000213, 8.999999999999992895 ) ) ;
#15747=CARTESIAN_POINT ( 'NONE',  ( 17.74085449832164585, 19.25660402617361910, 12.99999999999999467 ) ) ;
#15749=ORIENTED_EDGE ( 'NONE', *, *, #14683, .T. ) ;
#15751=FACE_OUTER_BOUND ( 'NONE', #10713, .T. ) ;
#15759=CARTESIAN_POINT ( 'NONE',  ( -3.756430356249997882, 25.85312499938548925, 11.16877607737301226 ) ) ;
#15762=CARTESIAN_POINT ( 'NONE',  ( 0.000000000000000000, 0.000000000000000000, 20.00001200000000168 ) ) ;
#15763=CARTESIAN_POINT ( 'NONE',  ( -3.469446951953614189E-15, -30.00000000000000355, 4.999999999999992006 ) ) ;
#15764=CARTESIAN_POINT ( 'NONE',  ( 16.89101323559370016, 22.54786748508600880, 6.690598923241487306 ) ) ;
#15765=CARTESIAN_POINT ( 'NONE',  ( 18.22334004483017011, 23.53573480074883761, 8.999999999999992895 ) ) ;
#15768=CARTESIAN_POINT ( 'NONE',  ( 23.34380806741302905, 18.84377675208414971, 6.562149109989046103 ) ) ;
#15772=CARTESIAN_POINT ( 'NONE',  ( 3.999999999999996447, -25.67500000000000071, 8.999999999999992895 ) ) ;
#15789=( BOUNDED_CURVE ( )  B_SPLINE_CURVE ( 2, ( #8858, #12903, #16456, #8592, #4527, #18543, #22974, #2967, #16845 ),
 .UNSPECIFIED., .F., .F. ) 
 B_SPLINE_CURVE_WITH_KNOTS ( ( 3, 2, 2, 2, 3 ),
 ( 0.07500000000000001110, 0.08333333333333332871, 0.1000000000000000056, 0.1166666666666666685, 0.1250000000000000000 ),
 .UNSPECIFIED. ) 
 CURVE ( )  GEOMETRIC_REPRESENTATION_ITEM ( )  RATIONAL_B_SPLINE_CURVE ( ( 0.9330127018922192983, 0.9330127018922194093, 1.000000000000000000, 0.8660254037844387076, 1.000000000000000000, 0.8660254037844387076, 1.000000000000000000, 0.9330127018922194093, 0.9330127018922194093 ) ) 
 REPRESENTATION_ITEM ( '' )  );
#15793=CARTESIAN_POINT ( 'NONE',  ( -1.152368580279349075, -29.97923206407486774, 12.84165680230635509 ) ) ;
#15794=CARTESIAN_POINT ( 'NONE',  ( 21.21320343559646915, 21.21320343559638744, 12.99999999999999289 ) ) ;
#15795=LINE ( 'NONE', #16064, #14565 ) ;
#15796=CARTESIAN_POINT ( 'NONE',  ( 15.26024822061316399, 20.91710247010547619, 6.690598923241487306 ) ) ;
#15813=ORIENTED_EDGE ( 'NONE', *, *, #7588, .F. ) ;
#15824=CARTESIAN_POINT ( 'NONE',  ( 1.878215178125004048, 29.37812499938548783, 5.746835883940462963 ) ) ;
#15829=DIRECTION ( 'NONE',  ( 0.000000000000000000, -1.000000000000000000, 0.000000000000000000 ) ) ;
#15830=CARTESIAN_POINT ( 'NONE',  ( 5.577813053751546416E-15, 25.73124999877097352, 12.99999999999999289 ) ) ;
#15832=CARTESIAN_POINT ( 'NONE',  ( -4.000000000000003553, -29.03124999877096712, 6.690598923241489970 ) ) ;
#15833=CARTESIAN_POINT ( 'NONE',  ( 3.735045420075836212E-15, 27.61562499938548498, 4.662447845253954171 ) ) ;
#15835=ADVANCED_FACE ( 'NONE', ( #9818 ), #1465, .F. ) ;
#15837=CARTESIAN_POINT ( 'NONE',  ( 21.21320343559646915, 21.21320343559638744, 8.999999999999992895 ) ) ;
#15839=ORIENTED_EDGE ( 'NONE', *, *, #16128, .F. ) ;
#15843=ORIENTED_EDGE ( 'NONE', *, *, #19030, .F. ) ;
#15847=CARTESIAN_POINT ( 'NONE',  ( -2.672651547586948120E-15, -27.39062499938548356, 13.33755215474602984 ) ) ;
#15854=CARTESIAN_POINT ( 'NONE',  ( 3.756430356250003211, 26.64062499938548356, 6.831223922626973533 ) ) ;
#15858=DIRECTION ( 'NONE',  ( -0.7071067811865487940, -0.7071067811865463515, 0.000000000000000000 ) ) ;
#15859=CARTESIAN_POINT ( 'NONE',  ( 19.84539375530421168, 19.84539375530412997, 4.662447845253954171 ) ) ;
#15864=EDGE_CURVE ( 'NONE', #7056, #7828, #20147, .T. ) ;
#15865=CARTESIAN_POINT ( 'NONE',  ( -1.999999999999995781, 29.19999999999999929, 5.535898384862237620 ) ) ;
#15867=CARTESIAN_POINT ( 'NONE',  ( 17.58694394176227149, 22.89933869768094610, 8.999999999999992895 ) ) ;
#15874=ORIENTED_EDGE ( 'NONE', *, *, #6465, .F. ) ;
#15876=CARTESIAN_POINT ( 'NONE',  ( 1.878215178125000939, 25.62812499938548783, 12.25316411605952283 ) ) ;
#15880=EDGE_CURVE ( 'NONE', #7544, #8072, #22097, .T. ) ;
#15881=ORIENTED_EDGE ( 'NONE', *, *, #6827, .T. ) ;
#15882=CARTESIAN_POINT ( 'NONE',  ( 3.999999999999995559, -25.63749999999999929, 6.690598923241487306 ) ) ;
#15886=DIRECTION ( 'NONE',  ( 0.000000000000000000, 1.000000000000000000, 0.000000000000000000 ) ) ;
#15891=CARTESIAN_POINT ( 'NONE',  ( 4.000000000000001776, 29.40624999877096357, 11.30940107675849760 ) ) ;
#15898=CARTESIAN_POINT ( 'NONE',  ( 20.73590635829554429, 17.90747923354928162, 5.535898384862238508 ) ) ;
#15899=CARTESIAN_POINT ( 'NONE',  ( 16.63234978716043244, 21.94474454307910705, 8.999999999999992895 ) ) ;
#15900=DIRECTION ( 'NONE',  ( 1.000000000000000000, 0.000000000000000000, -0.000000000000000000 ) ) ;
#15906=ORIENTED_EDGE ( 'NONE', *, *, #24557, .F. ) ;
#15908=CARTESIAN_POINT ( 'NONE',  ( -3.752267015613588906E-15, -26.01249999999999929, 4.381197846482986158 ) ) ;
#15918=ORIENTED_EDGE ( 'NONE', *, *, #15626, .T. ) ;
#15919=EDGE_CURVE ( 'NONE', #22563, #10227, #24191, .T. ) ;
#15933=CARTESIAN_POINT ( 'NONE',  ( 20.89942480057588980, 20.89942480057579033, 4.999999999999992006 ) ) ;
#15935=CARTESIAN_POINT ( 'NONE',  ( 16.96614333022570875, 19.79457045497182577, 5.535898384862237620 ) ) ;
#15938=CARTESIAN_POINT ( 'NONE',  ( 3.013468763610312351, 29.84883905190463338, 6.356741067357151387 ) ) ;
#15940=CYLINDRICAL_SURFACE ( 'NONE', #783, 4.000000000000000000 ) ;
#15941=VECTOR ( 'NONE', #1661, 1000.000000000000000 ) ;
#15942=CARTESIAN_POINT ( 'NONE',  ( -1.071796769724487230, 26.42634618820330061, 4.999999999999992006 ) ) ;
#15944=ORIENTED_EDGE ( 'NONE', *, *, #24471, .T. ) ;
#15946=CARTESIAN_POINT ( 'NONE',  ( -3.999999999999996003, 26.03124999877097068, 6.690598923241487306 ) ) ;
#15948=CARTESIAN_POINT ( 'NONE',  ( 1.071796769724487230, -26.42634618820330061, 4.999999999999992006 ) ) ;
#15952=ORIENTED_EDGE ( 'NONE', *, *, #7141, .T. ) ;
#15953=ORIENTED_EDGE ( 'NONE', *, *, #18568, .T. ) ;
#15956=( BOUNDED_CURVE ( )  B_SPLINE_CURVE ( 2, ( #18888, #20586, #6853, #10634, #20981, #18626, #16929, #5018, #13001 ),
 .UNSPECIFIED., .F., .F. ) 
 B_SPLINE_CURVE_WITH_KNOTS ( ( 3, 2, 2, 2, 3 ),
 ( 0.3250000000000000111, 0.3333333333333333148, 0.3499999999999999778, 0.3666666666666666408, 0.3750000000000000000 ),
 .UNSPECIFIED. ) 
 CURVE ( )  GEOMETRIC_REPRESENTATION_ITEM ( )  RATIONAL_B_SPLINE_CURVE ( ( 0.9330127018922194093, 0.9330127018922196314, 1.000000000000000000, 0.8660254037844387076, 1.000000000000000000, 0.8660254037844387076, 1.000000000000000000, 0.9330127018922194093, 0.9330127018922194093 ) ) 
 REPRESENTATION_ITEM ( '' )  );
#15957=VECTOR ( 'NONE', #6443, 1000.000000000000000 ) ;
#15961=( BOUNDED_CURVE ( )  B_SPLINE_CURVE ( 2, ( #20224, #2320, #4776, #11153, #22940, #20845, #9462, #21228, #1489 ),
 .UNSPECIFIED., .F., .F. ) 
 B_SPLINE_CURVE_WITH_KNOTS ( ( 3, 2, 2, 2, 3 ),
 ( 0.2750000000000000222, 0.2833333333333333259, 0.2999999999999999889, 0.3166666666666666519, 0.3250000000000000111 ),
 .UNSPECIFIED. ) 
 CURVE ( )  GEOMETRIC_REPRESENTATION_ITEM ( )  RATIONAL_B_SPLINE_CURVE ( ( 0.9330127018922194093, 0.9330127018922196314, 1.000000000000000000, 0.8660254037844387076, 1.000000000000000000, 0.8660254037844387076, 1.000000000000000000, 0.9330127018922191873, 0.9330127018922194093 ) ) 
 REPRESENTATION_ITEM ( '' )  );
#15967=CARTESIAN_POINT ( 'NONE',  ( -1.878215178124998497, 28.25312499938548427, 12.25316411605951927 ) ) ;
#15977=CARTESIAN_POINT ( 'NONE',  ( -4.000000000000001776, -29.85624999877096997, 11.30940107675849760 ) ) ;
#15979=CARTESIAN_POINT ( 'NONE',  ( 3.756430356250003655, 27.50312499938548427, 8.999999999999992895 ) ) ;
#15982=DIRECTION ( 'NONE',  ( 0.7071067811865487940, 0.7071067811865463515, 0.000000000000000000 ) ) ;
#15983=ORIENTED_EDGE ( 'NONE', *, *, #19707, .T. ) ;
#15985=CARTESIAN_POINT ( 'NONE',  ( 3.756430356249996105, -29.37812499938548427, 6.831223922626973533 ) ) ;
#15993=EDGE_LOOP ( 'NONE', ( #4757, #14549, #1028, #15693 ) ) ;
#15995=CARTESIAN_POINT ( 'NONE',  ( -3.756430356249996105, 25.44062499938548427, 6.831223922626973533 ) ) ;
#15999=CARTESIAN_POINT ( 'NONE',  ( 16.84448182151639628, 22.15687657743507089, 6.831223922626973533 ) ) ;
#16003=CARTESIAN_POINT ( 'NONE',  ( 3.752267015613588906E-15, 28.26250000000000284, 4.381197846482986158 ) ) ;
#16007=CARTESIAN_POINT ( 'NONE',  ( 23.66831732222138740, 18.35592256630256003, 11.16877607737301403 ) ) ;
#16015=CARTESIAN_POINT ( 'NONE',  ( 2.000000000000003997, 29.51874999877096784, 5.535898384862238508 ) ) ;
#16016=CARTESIAN_POINT ( 'NONE',  ( 15.63147928073609982, 21.28833353022841379, 11.30940107675849404 ) ) ;
#16021=ORIENTED_EDGE ( 'NONE', *, *, #21544, .F. ) ;
#16030=CARTESIAN_POINT ( 'NONE',  ( 2.672651547586948120E-15, 25.47812499938548569, 13.33755215474602984 ) ) ;
#16033=SHAPE_REPRESENTATION ( 'casing', ( #21036 ), #8093 ) ;
#16036=CARTESIAN_POINT ( 'NONE',  ( 16.30765014111479516, 21.96450439060710380, 11.30940107675849404 ) ) ;
#16040=CARTESIAN_POINT ( 'NONE',  ( 2.000000000000003997, 25.07499999999999929, 5.535898384862238508 ) ) ;
#16042=CARTESIAN_POINT ( 'NONE',  ( 20.40224034548861809, 20.40224034548853993, 4.662447845253954171 ) ) ;
#16045=CARTESIAN_POINT ( 'NONE',  ( -3.752267015613588906E-15, -27.81250000000000000, 4.381197846482986158 ) ) ;
#16054=CARTESIAN_POINT ( 'NONE',  ( 4.000000000000001776, 28.05624999877096570, 11.30940107675849760 ) ) ;
#16058=CYLINDRICAL_SURFACE ( 'NONE', #14594, 30.00000000000000355 ) ;
#16063=CARTESIAN_POINT ( 'NONE',  ( 20.62100150635272300, 20.62100150635266260, 4.999999999999992006 ) ) ;
#16064=CARTESIAN_POINT ( 'NONE',  ( -3.959305671612554781E-15, -30.00000000000000355, 12.99999999999999289 ) ) ;
#16065=CARTESIAN_POINT ( 'NONE',  ( 20.59006558380675855, 17.76163845906049943, 12.46410161513774817 ) ) ;
#16072=CARTESIAN_POINT ( 'NONE',  ( -1.773386257881301553, 29.94852044693267246, 12.59496732558994125 ) ) ;
#16076=CARTESIAN_POINT ( 'NONE',  ( 1.071796769724492338, 27.10134618820329777, 12.99999999999999467 ) ) ;
#16077=CARTESIAN_POINT ( 'NONE',  ( 25.99307600111999150, 0.5999999999999998668, 19.59999999999999787 ) ) ;
#16086=CARTESIAN_POINT ( 'NONE',  ( 0.000000000000000000, 10.00000000000000000, 15.00000000000000178 ) ) ;
#16090=CARTESIAN_POINT ( 'NONE',  ( -3.756430356249996994, 26.26562499938548711, 8.999999999999992895 ) ) ;
#16093=EDGE_CURVE ( 'NONE', #4544, #15602, #24850, .T. ) ;
#16096=CARTESIAN_POINT ( 'NONE',  ( 1.999999999999995781, -25.54374999877096997, 5.535898384862237620 ) ) ;
#16098=CARTESIAN_POINT ( 'NONE',  ( 1.999999999999995781, -29.59374999877096712, 5.535898384862237620 ) ) ;
#16099=CARTESIAN_POINT ( 'NONE',  ( -1.878215178124995832, 29.00312499938548427, 5.746835883940462963 ) ) ;
#16102=CARTESIAN_POINT ( 'NONE',  ( -3.999999999999995559, 29.63124999877096855, 6.690598923241487306 ) ) ;
#16104=EDGE_LOOP ( 'NONE', ( #16980, #160, #1275, #15721, #11651, #6358 ) ) ;
#16106=CARTESIAN_POINT ( 'NONE',  ( -3.756430356250003655, -28.74062499938548498, 8.999999999999992895 ) ) ;
#16107=EDGE_LOOP ( 'NONE', ( #2281, #21280, #8578, #17873 ) ) ;
#16114=( BOUNDED_CURVE ( )  B_SPLINE_CURVE ( 2, ( #2237, #12548, #20260, #10194, #274, #24188, #6659, #2742, #10448 ),
 .UNSPECIFIED., .F., .F. ) 
 B_SPLINE_CURVE_WITH_KNOTS ( ( 3, 2, 2, 2, 3 ),
 ( 0.1249999999999999861, 0.1333333333333333315, 0.1499999999999999944, 0.1666666666666666574, 0.1750000000000000167 ),
 .UNSPECIFIED. ) 
 CURVE ( )  GEOMETRIC_REPRESENTATION_ITEM ( )  RATIONAL_B_SPLINE_CURVE ( ( 0.9330127018922194093, 0.9330127018922192983, 1.000000000000000000, 0.8660254037844387076, 1.000000000000000000, 0.8660254037844387076, 1.000000000000000000, 0.9330127018922191873, 0.9330127018922194093 ) ) 
 REPRESENTATION_ITEM ( '' )  );
#16118=CARTESIAN_POINT ( 'NONE',  ( 1.878215178125000939, 26.97812499938548569, 12.25316411605952283 ) ) ;
#16122=CARTESIAN_POINT ( 'NONE',  ( 18.65215106205190310, 18.65215106205183915, 13.33755215474602984 ) ) ;
#16127=CARTESIAN_POINT ( 'NONE',  ( -1.999999999999998224, 28.44999999999999929, 12.46410161513774639 ) ) ;
#16128=EDGE_CURVE ( 'NONE', #12209, #4122, #23146, .T. ) ;
#16130=PLANE ( 'NONE',  #17158 ) ;
#16131=CARTESIAN_POINT ( 'NONE',  ( 21.78337204305729458, 19.12717466509784003, 5.746835883940462963 ) ) ;
#16133=ORIENTED_EDGE ( 'NONE', *, *, #2336, .T. ) ;
#16139=CARTESIAN_POINT ( 'NONE',  ( 1.878215178125004048, 26.22812499938548569, 5.746835883940462963 ) ) ;
#16143=ADVANCED_FACE ( 'NONE', ( #24718 ), #19081, .F. ) ;
#16152=FACE_OUTER_BOUND ( 'NONE', #11436, .T. ) ;
#16157=DIRECTION ( 'NONE',  ( 1.000000000000000000, 0.000000000000000000, 0.000000000000000000 ) ) ;
#16158=CARTESIAN_POINT ( 'NONE',  ( -3.735045420075836212E-15, -25.25312499938548427, 4.662447845253954171 ) ) ;
#16159=EDGE_CURVE ( 'NONE', #11855, #1614, #6804, .T. ) ;
#16163=CARTESIAN_POINT ( 'NONE',  ( 3.999999999999997335, -28.86250000000000071, 11.30940107675849404 ) ) ;
#16169=ORIENTED_EDGE ( 'NONE', *, *, #10752, .F. ) ;
#16172=CARTESIAN_POINT ( 'NONE',  ( 4.000000000000003553, 28.09374999877097068, 8.999999999999992895 ) ) ;
#16179=CARTESIAN_POINT ( 'NONE',  ( 19.09750500040671284, 17.58175547255459747, 4.999999999999993783 ) ) ;
#16181=CARTESIAN_POINT ( 'NONE',  ( 16.57931677857143882, 21.89171153449011697, 11.16877607737301226 ) ) ;
#16183=CARTESIAN_POINT ( 'NONE',  ( 22.72022476213123099, 17.06337051263877669, 6.690598923241489970 ) ) ;
#16188=CARTESIAN_POINT ( 'NONE',  ( -3.871674220476135631, 29.74916513505594295, 7.961019890438434388 ) ) ;
#16190=CARTESIAN_POINT ( 'NONE',  ( 18.87091222291601866, 18.87091222291595827, 12.99999999999999289 ) ) ;
#16194=CARTESIAN_POINT ( 'NONE',  ( 1.878215178124995832, -27.09062499938548640, 5.746835883940462963 ) ) ;
#16196=ORIENTED_EDGE ( 'NONE', *, *, #21594, .T. ) ;
#16197=ORIENTED_EDGE ( 'NONE', *, *, #14086, .T. ) ;
#16200=ADVANCED_FACE ( 'NONE', ( #3384 ), #5861, .T. ) ;
#16208=( BOUNDED_CURVE ( )  B_SPLINE_CURVE ( 2, ( #10633, #12218, #14449, #710, #18625, #14326, #22289, #16660, #16418 ),
 .UNSPECIFIED., .F., .F. ) 
 B_SPLINE_CURVE_WITH_KNOTS ( ( 3, 2, 2, 2, 3 ),
 ( 0.3750000000000000000, 0.3833333333333333592, 0.4000000000000000222, 0.4166666666666666852, 0.4250000000000000444 ),
 .UNSPECIFIED. ) 
 CURVE ( )  GEOMETRIC_REPRESENTATION_ITEM ( )  RATIONAL_B_SPLINE_CURVE ( ( 0.9330127018922194093, 0.9330127018922194093, 1.000000000000000000, 0.8660254037844387076, 1.000000000000000000, 0.8660254037844387076, 1.000000000000000000, 0.9330127018922191873, 0.9330127018922194093 ) ) 
 REPRESENTATION_ITEM ( '' )  );
#16212=CARTESIAN_POINT ( 'NONE',  ( -3.756430356249997882, 26.75312499938548427, 11.16877607737301226 ) ) ;
#16213=CARTESIAN_POINT ( 'NONE',  ( -3.137519842735244810E-15, 27.30624999877096926, 4.999999999999991118 ) ) ;
#16219=CARTESIAN_POINT ( 'NONE',  ( -3.756430356250002323, -25.66562499938548569, 11.16877607737301226 ) ) ;
#16220=CARTESIAN_POINT ( 'NONE',  ( 20.14370442905180525, 20.14370442905174130, 12.99999999999999289 ) ) ;
#16222=VECTOR ( 'NONE', #16915, 1000.000000000000000 ) ;
#16224=CARTESIAN_POINT ( 'NONE',  ( 3.471149744654747238, -29.79887180468049479, 6.994934987683496530 ) ) ;
#16229=VECTOR ( 'NONE', #7096, 999.9999999999998863 ) ;
#16233=EDGE_LOOP ( 'NONE', ( #8334, #19409 ) ) ;
#16235=CARTESIAN_POINT ( 'NONE',  ( 22.73348301514753800, 17.07662876565508370, 8.999999999999992895 ) ) ;
#16236=ORIENTED_EDGE ( 'NONE', *, *, #1096, .T. ) ;
#16239=CARTESIAN_POINT ( 'NONE',  ( -3.756430356249997438, 26.86562499938548498, 11.16877607737301048 ) ) ;
#16245=CARTESIAN_POINT ( 'NONE',  ( 19.79463422097012426, 17.13843684301067682, 5.746835883940462963 ) ) ;
#16248=AXIS2_PLACEMENT_3D ( 'NONE', #14018, #2982, #14761 ) ;
#16253=CARTESIAN_POINT ( 'NONE',  ( 3.756430356250002323, 29.60312499938548569, 11.16877607737301403 ) ) ;
#16256=CARTESIAN_POINT ( 'NONE',  ( -2.000000000000000888, -28.07500000000000284, 12.46410161513774817 ) ) ;
#16258=ORIENTED_EDGE ( 'NONE', *, *, #25333, .T. ) ;
#16264=ORIENTED_EDGE ( 'NONE', *, *, #20808, .F. ) ;
#16265=CARTESIAN_POINT ( 'NONE',  ( 19.41570305194066037, 17.89995352408853790, 4.999999999999992895 ) ) ;
#16272=EDGE_CURVE ( 'NONE', #17199, #18353, #25498, .T. ) ;
#16275=ADVANCED_FACE ( 'NONE', ( #7820 ), #15940, .F. ) ;
#16282=CARTESIAN_POINT ( 'NONE',  ( -3.756430356249995661, 28.47812499938548569, 6.831223922626973533 ) ) ;
#16283=VECTOR ( 'NONE', #6102, 1000.000000000000000 ) ;
#16287=CARTESIAN_POINT ( 'NONE',  ( 19.23330444827413643, 22.06173157302024634, 5.535898384862237620 ) ) ;
#16293=VERTEX_POINT ( 'NONE', #11362 ) ;
#16300=VECTOR ( 'NONE', #20888, 1000.000000000000000 ) ;
#16304=ORIENTED_EDGE ( 'NONE', *, *, #9962, .T. ) ;
#16305=CARTESIAN_POINT ( 'NONE',  ( 3.756430356249996105, -26.79062499938548569, 6.831223922626973533 ) ) ;
#16317=CARTESIAN_POINT ( 'NONE',  ( -1.878215178124995832, 25.29062499938548569, 5.746835883940462963 ) ) ;
#16319=CARTESIAN_POINT ( 'NONE',  ( 20.00801561637006643, 21.52376514422204323, 12.99999999999999289 ) ) ;
#16320=CARTESIAN_POINT ( 'NONE',  ( 16.52628376998245230, 21.83867852590112690, 6.831223922626973533 ) ) ;
#16321=CARTESIAN_POINT ( 'NONE',  ( 16.58607343533793710, 22.24292768483024929, 11.30940107675849404 ) ) ;
#16324=CARTESIAN_POINT ( 'NONE',  ( 20.78010053211970032, 20.78010053211962926, 12.99999999999999289 ) ) ;
#16332=DIRECTION ( 'NONE',  ( 1.000000000000000000, 0.000000000000000000, 0.000000000000000000 ) ) ;
#16333=CARTESIAN_POINT ( 'NONE',  ( 2.000000000000000888, 26.66874999877096641, 12.46410161513774817 ) ) ;
#16334=CARTESIAN_POINT ( 'NONE',  ( -3.756430356250003655, -26.49062499938548498, 8.999999999999992895 ) ) ;
#16339=CARTESIAN_POINT ( 'NONE',  ( 1.878215178124995832, -29.45312499938548356, 5.746835883940462963 ) ) ;
#16342=VERTEX_POINT ( 'NONE', #23526 ) ;
#16348=VECTOR ( 'NONE', #14361, 1000.000000000000000 ) ;
#16352=CARTESIAN_POINT ( 'NONE',  ( -1.878215178124998497, 25.44062499938548427, 12.25316411605951927 ) ) ;
#16360=CARTESIAN_POINT ( 'NONE',  ( -1.859271017917182139E-15, -26.68750000000000000, 12.99999999999999289 ) ) ;
#16362=CARTESIAN_POINT ( 'NONE',  ( -4.000000000000001776, -28.50624999877096855, 11.30940107675849760 ) ) ;
#16364=CARTESIAN_POINT ( 'NONE',  ( -3.756430356249995661, 29.49062499938548498, 6.831223922626973533 ) ) ;
#16365=VECTOR ( 'NONE', #18271, 1000.000000000000000 ) ;
#16370=EDGE_CURVE ( 'NONE', #18353, #21212, #14486, .T. ) ;
#16384=CARTESIAN_POINT ( 'NONE',  ( 3.735045420075836212E-15, 27.61562499938548498, 4.662447845253954171 ) ) ;
#16388=CARTESIAN_POINT ( 'NONE',  ( 22.34249210749660364, 17.03009735157778337, 8.999999999999992895 ) ) ;
#16389=VECTOR ( 'NONE', #8585, 1000.000000000000000 ) ;
#16395=CARTESIAN_POINT ( 'NONE',  ( 2.672651547586948120E-15, 29.07812499938548356, 13.33755215474603162 ) ) ;
#16397=LINE ( 'NONE', #10342, #15957 ) ;
#16400=EDGE_LOOP ( 'NONE', ( #18736, #7379, #20303, #12530 ) ) ;
#16405=ORIENTED_EDGE ( 'NONE', *, *, #9966, .F. ) ;
#16408=CARTESIAN_POINT ( 'NONE',  ( 8.831537335106614961E-15, 26.23749999999999716, 12.99999999999999112 ) ) ;
#16411=EDGE_CURVE ( 'NONE', #5788, #25106, #9402, .T. ) ;
#16412=CARTESIAN_POINT ( 'NONE',  ( 1.071796769724487230, -25.58259618943233704, 4.999999999999992006 ) ) ;
#16418=CARTESIAN_POINT ( 'NONE',  ( -3.137519842735244810E-15, 26.91249999999999787, 4.999999999999991118 ) ) ;
#16419=CARTESIAN_POINT ( 'NONE',  ( 4.000000000000003553, 29.44374999877096855, 8.999999999999992895 ) ) ;
#16422=CARTESIAN_POINT ( 'NONE',  ( 3.735045420075836212E-15, 28.85312499938548569, 4.662447845253954171 ) ) ;
#16427=CARTESIAN_POINT ( 'NONE',  ( 18.70297436238422506, 21.53140148713034208, 12.46410161513774639 ) ) ;
#16428=CARTESIAN_POINT ( 'NONE',  ( -1.999999999999998224, 29.35000000000000142, 12.46410161513774639 ) ) ;
#16431=EDGE_CURVE ( 'NONE', #12726, #15349, #24295, .T. ) ;
#16434=EDGE_LOOP ( 'NONE', ( #15843, #4978, #15620, #8640 ) ) ;
#16436=CARTESIAN_POINT ( 'NONE',  ( -4.000000000000001776, -28.56249999999999645, 11.30940107675849760 ) ) ;
#16438=ORIENTED_EDGE ( 'NONE', *, *, #11382, .F. ) ;
#16439=ORIENTED_EDGE ( 'NONE', *, *, #24073, .T. ) ;
#16440=CARTESIAN_POINT ( 'NONE',  ( 1.999999999999998224, -29.29374999877096997, 12.46410161513774639 ) ) ;
#16441=CYLINDRICAL_SURFACE ( 'NONE', #24675, 4.000000000000000000 ) ;
#16443=ORIENTED_EDGE ( 'NONE', *, *, #12659, .F. ) ;
#16445=CARTESIAN_POINT ( 'NONE',  ( -3.756430356250003211, -25.74062499938548498, 6.831223922626973533 ) ) ;
#16447=CARTESIAN_POINT ( 'NONE',  ( 2.000000000000000888, 28.01874999877096784, 12.46410161513774817 ) ) ;
#16454=LINE ( 'NONE', #4668, #9247 ) ;
#16456=CARTESIAN_POINT ( 'NONE',  ( 2.000000000000000888, 25.37500000000000000, 12.46410161513774817 ) ) ;
#16457=CARTESIAN_POINT ( 'NONE',  ( 21.06969990136081705, 15.75730514544200211, 8.999999999999992895 ) ) ;
#16458=CARTESIAN_POINT ( 'NONE',  ( 23.64830241243857500, 17.99144816294611715, 8.999999999999992895 ) ) ;
#16460=CARTESIAN_POINT ( 'NONE',  ( 1.859271017917182139E-15, 26.18124999877096570, 12.99999999999999289 ) ) ;
#16462=CARTESIAN_POINT ( 'NONE',  ( -1.774938052278379752, 29.94842879300231075, 5.405792698933810314 ) ) ;
#16466=DIRECTION ( 'NONE',  ( 1.000000000000000000, 0.000000000000000000, 0.000000000000000000 ) ) ;
#16467=ORIENTED_EDGE ( 'NONE', *, *, #1394, .T. ) ;
#16468=CARTESIAN_POINT ( 'NONE',  ( -3.137519842735244810E-15, 27.30624999877096926, 4.999999999999991118 ) ) ;
#16469=CARTESIAN_POINT ( 'NONE',  ( -3.999999999999996003, 26.48124999877096641, 6.690598923241487306 ) ) ;
#16470=CARTESIAN_POINT ( 'NONE',  ( 1.878215178124995832, -27.54062499938548214, 5.746835883940462963 ) ) ;
#16471=CARTESIAN_POINT ( 'NONE',  ( 17.00591808753650724, 19.83434521228262426, 5.535898384862237620 ) ) ;
#16473=PLANE ( 'NONE',  #16248 ) ;
#16475=ORIENTED_EDGE ( 'NONE', *, *, #12460, .F. ) ;
#16476=CARTESIAN_POINT ( 'NONE',  ( 3.756430356249996994, -25.81562499938548427, 8.999999999999992895 ) ) ;
#16485=CARTESIAN_POINT ( 'NONE',  ( 1.878215178125000939, 25.51562499938548356, 12.25316411605952283 ) ) ;
#16492=CARTESIAN_POINT ( 'NONE',  ( -1.878215178125004048, -27.12812499938548783, 5.746835883940462963 ) ) ;
#16496=CARTESIAN_POINT ( 'NONE',  ( -1.999999999999995781, 27.85000000000000142, 5.535898384862237620 ) ) ;
#16499=DIRECTION ( 'NONE',  ( 0.8660254037844397068, -0.4999999999999983347, 0.000000000000000000 ) ) ;
#16507=DIRECTION ( 'NONE',  ( -0.000000000000000000, -0.000000000000000000, 1.000000000000000000 ) ) ;
#16509=EDGE_LOOP ( 'NONE', ( #7168, #10911, #10356, #14465 ) ) ;
#16510=EDGE_CURVE ( 'NONE', #23536, #11588, #14151, .T. ) ;
#16515=CARTESIAN_POINT ( 'NONE',  ( 16.26111872703749128, 21.57351348295617299, 11.16877607737301226 ) ) ;
#16523=CARTESIAN_POINT ( 'NONE',  ( -1.878215178124998497, 28.59062499938548285, 12.25316411605951927 ) ) ;
#16525=CARTESIAN_POINT ( 'NONE',  ( 1.071796769724495668, 27.55134618820330061, 12.99999999999999112 ) ) ;
#16536=ORIENTED_EDGE ( 'NONE', *, *, #13962, .F. ) ;
#16547=CARTESIAN_POINT ( 'NONE',  ( -3.756430356249997882, 28.55312499938548498, 11.16877607737301226 ) ) ;
#16548=CARTESIAN_POINT ( 'NONE',  ( 15.38607408531914089, 20.69846884123781550, 11.16877607737301048 ) ) ;
#16549=CARTESIAN_POINT ( 'NONE',  ( 19.33937046545212013, 22.16779759019823359, 12.46410161513774639 ) ) ;
#16551=CARTESIAN_POINT ( 'NONE',  ( 20.10392967174102097, 20.10392967174092860, 12.99999999999999289 ) ) ;
#16552=CARTESIAN_POINT ( 'NONE',  ( 1.878215178124998497, -26.34062499938548285, 12.25316411605951927 ) ) ;
#16556=CARTESIAN_POINT ( 'NONE',  ( -4.000000000000003553, -29.05000000000000071, 8.999999999999992895 ) ) ;
#16563=CARTESIAN_POINT ( 'NONE',  ( -3.735045420075836212E-15, -27.61562499938548498, 4.662447845253954171 ) ) ;
#16565=CARTESIAN_POINT ( 'NONE',  ( -1.071796769724487675, -29.08615380933863293, 4.999999999999988454 ) ) ;
#16568=EDGE_CURVE ( 'NONE', #6938, #10501, #21143, .T. ) ;
#16569=LINE ( 'NONE', #10661, #19610 ) ;
#16571=CARTESIAN_POINT ( 'NONE',  ( 17.96051224213834985, 20.78893936688446331, 5.535898384862237620 ) ) ;
#16573=CARTESIAN_POINT ( 'NONE',  ( 3.756430356250003655, 25.14062499938548356, 8.999999999999992895 ) ) ;
#16574=CARTESIAN_POINT ( 'NONE',  ( 20.27186753227280747, 17.44344040752655545, 12.46410161513774817 ) ) ;
#16575=CARTESIAN_POINT ( 'NONE',  ( 20.00676625532608455, 17.35056887736664422, 12.25316411605952283 ) ) ;
#16576=CARTESIAN_POINT ( 'NONE',  ( 21.01432965251868978, 18.18590252777242711, 5.535898384862238508 ) ) ;
#16581=ORIENTED_EDGE ( 'NONE', *, *, #23161, .F. ) ;
#16583=CARTESIAN_POINT ( 'NONE',  ( -3.959305671612554781E-15, -30.00000000000000355, 12.99999999999999289 ) ) ;
#16586=CARTESIAN_POINT ( 'NONE',  ( 4.000000000000001776, 28.05624999877096926, 11.30940107675849760 ) ) ;
#16587=CARTESIAN_POINT ( 'NONE',  ( -3.756430356250002323, -26.90312499938548640, 11.16877607737301226 ) ) ;
#16593=CARTESIAN_POINT ( 'NONE',  ( -2.672651547586948120E-15, -25.92812499938548498, 13.33755215474602984 ) ) ;
#16597=CARTESIAN_POINT ( 'NONE',  ( 4.000000000000003553, 27.73750000000000071, 6.690598923241489970 ) ) ;
#16600=CARTESIAN_POINT ( 'NONE',  ( -1.878215178124995832, 26.19062499938548427, 5.746835883940462963 ) ) ;
#16605=FACE_OUTER_BOUND ( 'NONE', #7919, .T. ) ;
#16608=CARTESIAN_POINT ( 'NONE',  ( 3.756430356249995661, -27.24062499938548498, 6.831223922626973533 ) ) ;
#16609=CARTESIAN_POINT ( 'NONE',  ( 3.735045420075836212E-15, 29.41562499938548569, 4.662447845253954171 ) ) ;
#16614=VERTEX_POINT ( 'NONE', #12909 ) ;
#16626=CARTESIAN_POINT ( 'NONE',  ( 1.878215178125000939, 27.87812499938548427, 12.25316411605952283 ) ) ;
#16629=CARTESIAN_POINT ( 'NONE',  ( 20.56133937125558830, 20.56133937125551370, 13.33755215474602984 ) ) ;
#16642=AXIS2_PLACEMENT_3D ( 'NONE', #20562, #8931, #8789 ) ;
#16645=ORIENTED_EDGE ( 'NONE', *, *, #12222, .F. ) ;
#16650=CARTESIAN_POINT ( 'NONE',  ( 1.878215178124995832, -25.40312499938548640, 5.746835883940462963 ) ) ;
#16656=CYLINDRICAL_SURFACE ( 'NONE', #13925, 4.000000000000000000 ) ;
#16660=CARTESIAN_POINT ( 'NONE',  ( 1.071796769724491227, 26.89240381056766793, 4.999999999999989342 ) ) ;
#16662=EDGE_CURVE ( 'NONE', #18727, #16889, #10636, .T. ) ;
#16663=CARTESIAN_POINT ( 'NONE',  ( 22.10384356884614121, 16.79144881292732450, 8.999999999999992895 ) ) ;
#16664=CARTESIAN_POINT ( 'NONE',  ( 3.756430356250003655, 26.94062499938548427, 8.999999999999992895 ) ) ;
#16668=CARTESIAN_POINT ( 'NONE',  ( 20.62100150635273366, 20.62100150635265905, 4.381197846482986158 ) ) ;
#16672=VECTOR ( 'NONE', #16717, 1000.000000000000000 ) ;
#16673=CARTESIAN_POINT ( 'NONE',  ( -1.878215178125004048, -27.01562499938548711, 5.746835883940462963 ) ) ;
#16682=VERTEX_POINT ( 'NONE', #13435 ) ;
#16686=CARTESIAN_POINT ( 'NONE',  ( 3.756430356249997438, -26.86562499938548498, 11.16877607737301048 ) ) ;
#16699=CIRCLE ( 'NONE', #10401, 4.000000000000000000 ) ;
#16701=CARTESIAN_POINT ( 'NONE',  ( 21.27955846146187113, 18.62336108350243080, 12.25316411605952283 ) ) ;
#16702=CARTESIAN_POINT ( 'NONE',  ( 20.85756786700484966, 15.54517311108603472, 6.831223922626973533 ) ) ;
#16712=CARTESIAN_POINT ( 'NONE',  ( -3.999999999999997335, 27.90624999877097068, 11.30940107675849404 ) ) ;
#16713=CARTESIAN_POINT ( 'NONE',  ( 1.878215178124998497, -25.44062499938548427, 12.25316411605951927 ) ) ;
#16717=DIRECTION ( 'NONE',  ( 1.000000000000000000, 0.000000000000000000, 0.000000000000000000 ) ) ;
#16719=ADVANCED_FACE ( 'NONE', ( #23616 ), #23230, .F. ) ;
#16721=CARTESIAN_POINT ( 'NONE',  ( 3.756430356249997882, -29.56562499938549138, 11.16877607737301226 ) ) ;
#16723=ORIENTED_EDGE ( 'NONE', *, *, #16272, .T. ) ;
#16734=LINE ( 'NONE', #14775, #14712 ) ;
#16735=CARTESIAN_POINT ( 'NONE',  ( 1.878215178125004048, 27.91562499938548569, 5.746835883940462963 ) ) ;
#16742=CARTESIAN_POINT ( 'NONE',  ( 23.14903047711951345, 19.08292775625380600, 11.79623638833883881 ) ) ;
#16744=CARTESIAN_POINT ( 'NONE',  ( -3.756430356250003655, -27.50312499938548427, 8.999999999999992895 ) ) ;
#16746=CARTESIAN_POINT ( 'NONE',  ( -27.10000000000000497, -0.5999999999999998668, 19.59999999999999787 ) ) ;
#16749=CARTESIAN_POINT ( 'NONE',  ( 3.834746474454188013E-15, 27.81249999999999645, 4.999999999999992006 ) ) ;
#16752=DIRECTION ( 'NONE',  ( 0.000000000000000000, 1.000000000000000000, 0.000000000000000000 ) ) ;
#16758=ORIENTED_EDGE ( 'NONE', *, *, #12674, .F. ) ;
#16762=CARTESIAN_POINT ( 'NONE',  ( -2.000000000000000888, -27.62500000000000000, 12.46410161513774817 ) ) ;
#16766=CARTESIAN_POINT ( 'NONE',  ( -1.878215178124995832, 29.45312499938548356, 5.746835883940462963 ) ) ;
#16772=AXIS2_PLACEMENT_3D ( 'NONE', #11995, #9911, #14241 ) ;
#16775=CARTESIAN_POINT ( 'NONE',  ( -3.959305671612554781E-15, -30.00000000000000355, 12.99999999999999289 ) ) ;
#16783=CARTESIAN_POINT ( 'NONE',  ( 1.999999999999995781, -26.50000000000000355, 5.535898384862237620 ) ) ;
#16795=VECTOR ( 'NONE', #17257, 1000.000000000000000 ) ;
#16803=DIRECTION ( 'NONE',  ( 0.000000000000000000, 0.000000000000000000, -1.000000000000000000 ) ) ;
#16805=CARTESIAN_POINT ( 'NONE',  ( 27.09999999999999787, -0.5999999999999998668, 19.00000000000000000 ) ) ;
#16807=CARTESIAN_POINT ( 'NONE',  ( 18.57260154916842154, 18.57260154916834693, 4.662447845253954171 ) ) ;
#16808=( BOUNDED_CURVE ( )  B_SPLINE_CURVE ( 2, ( #24257, #24396, #2297, #16158, #12356, #2411, #11961, #10373, #18373, #4115, #20070, #10133, #17859, #22169, #12477, #19930, #18137, #8181, #4256, #2034, #329, #12230, #10003, #6472, #20197, #14458, #1914, #17998, #10254, #22420, #14580, #14967, #16552, #3071, #848, #20596, #20850, #24511, #4896, #7123, #6864, #2939, #22559, #14847, #10520, #22820, #18516, #11038, #10768, #24909, #16673, #720, #8964, #20994, #22698, #5030, #8686, #19017, #10904, #16939, #4641, #24640, #23083, #6728, #18637, #18901, #12624, #10642, #1101, #603, #6593, #20725, #9077, #14721, #2682, #983, #4780, #8829, #12753, #8570, #25033, #13011, #6985, #2803, #16818, #18758, #24781, #12873, #22946, #17060, #15109, #5169, #20450, #2550, #15491, #7255, #16106, #7374, #2108, #21861, #19272, #17203, #1373, #25174, #15235, #6031, #19878, #23321, #19403, #13399, #9348, #3455, #22, #15985, #9212, #1494, #23949, #159, #23460, #23200, #24070 ),
 .UNSPECIFIED., .F., .F. ) 
 B_SPLINE_CURVE_WITH_KNOTS ( ( 3, 2, 2, 2, 2, 2, 2, 2, 2, 2, 2, 2, 2, 2, 2, 2, 2, 2, 2, 2, 2, 2, 2, 2, 2, 2, 2, 2, 2, 2, 2, 2, 2, 2, 2, 2, 2, 2, 2, 2, 2, 2, 2, 2, 2, 2, 2, 2, 2, 2, 2, 2, 2, 2, 2, 2, 2, 2, 2, 2, 3 ),
 ( 0.000000000000000000, 0.01666666666666666644, 0.03333333333333333287, 0.05000000000000000278, 0.06666666666666666574, 0.08333333333333332871, 0.1000000000000000056, 0.1166666666666666685, 0.1333333333333333315, 0.1499999999999999944, 0.1666666666666666574, 0.1833333333333333204, 0.2000000000000000111, 0.2166666666666666741, 0.2333333333333333370, 0.2500000000000000000, 0.2666666666666666630, 0.2833333333333333259, 0.2999999999999999889, 0.3166666666666666519, 0.3333333333333333148, 0.3499999999999999778, 0.3666666666666666408, 0.3833333333333333592, 0.4000000000000000222, 0.4166666666666666852, 0.4333333333333333481, 0.4500000000000000111, 0.4666666666666666741, 0.4833333333333333370, 0.5000000000000000000, 0.5166666666666667185, 0.5333333333333333259, 0.5500000000000000444, 0.5666666666666666519, 0.5833333333333333703, 0.5999999999999999778, 0.6166666666666666963, 0.6333333333333333037, 0.6500000000000000222, 0.6666666666666666297, 0.6833333333333333481, 0.6999999999999999556, 0.7166666666666666741, 0.7333333333333332815, 0.7500000000000000000, 0.7666666666666667185, 0.7833333333333333259, 0.8000000000000000444, 0.8166666666666666519, 0.8333333333333333703, 0.8499999999999999778, 0.8666666666666666963, 0.8833333333333333037, 0.9000000000000000222, 0.9166666666666666297, 0.9333333333333333481, 0.9499999999999999556, 0.9666666666666666741, 0.9833333333333332815, 1.000000000000000000 ),
 .UNSPECIFIED. ) 
 CURVE ( )  GEOMETRIC_REPRESENTATION_ITEM ( )  RATIONAL_B_SPLINE_CURVE ( ( 1.000000000000000000, 0.8660254037844387076, 1.000000000000000000, 0.8660254037844387076, 1.000000000000000000, 0.8660254037844387076, 1.000000000000000000, 0.8660254037844387076, 1.000000000000000000, 0.8660254037844387076, 1.000000000000000000, 0.8660254037844387076, 1.000000000000000000, 0.8660254037844387076, 1.000000000000000000, 0.8660254037844387076, 1.000000000000000000, 0.8660254037844387076, 1.000000000000000000, 0.8660254037844387076, 1.000000000000000000, 0.8660254037844387076, 1.000000000000000000, 0.8660254037844387076, 1.000000000000000000, 0.8660254037844387076, 1.000000000000000000, 0.8660254037844387076, 1.000000000000000000, 0.8660254037844387076, 1.000000000000000000, 0.8660254037844387076, 1.000000000000000000, 0.8660254037844387076, 1.000000000000000000, 0.8660254037844387076, 1.000000000000000000, 0.8660254037844387076, 1.000000000000000000, 0.8660254037844387076, 1.000000000000000000, 0.8660254037844387076, 1.000000000000000000, 0.8660254037844387076, 1.000000000000000000, 0.8660254037844387076, 1.000000000000000000, 0.8660254037844387076, 1.000000000000000000, 0.8660254037844387076, 1.000000000000000000, 0.8660254037844387076, 1.000000000000000000, 0.8660254037844387076, 1.000000000000000000, 0.8660254037844387076, 1.000000000000000000, 0.8660254037844387076, 1.000000000000000000, 0.8660254037844387076, 1.000000000000000000, 0.8660254037844387076, 1.000000000000000000, 0.8660254037844387076, 1.000000000000000000, 0.8660254037844387076, 1.000000000000000000, 0.8660254037844387076, 1.000000000000000000, 0.8660254037844387076, 1.000000000000000000, 0.8660254037844387076, 1.000000000000000000, 0.8660254037844387076, 1.000000000000000000, 0.8660254037844387076, 1.000000000000000000, 0.8660254037844387076, 1.000000000000000000, 0.8660254037844387076, 1.000000000000000000, 0.8660254037844387076, 1.000000000000000000, 0.8660254037844387076, 1.000000000000000000, 0.8660254037844387076, 1.000000000000000000, 0.8660254037844387076, 1.000000000000000000, 0.8660254037844387076, 1.000000000000000000, 0.8660254037844387076, 1.000000000000000000, 0.8660254037844387076, 1.000000000000000000, 0.8660254037844387076, 1.000000000000000000, 0.8660254037844387076, 1.000000000000000000, 0.8660254037844387076, 1.000000000000000000, 0.8660254037844387076, 1.000000000000000000, 0.8660254037844387076, 1.000000000000000000, 0.8660254037844387076, 1.000000000000000000, 0.8660254037844387076, 1.000000000000000000, 0.8660254037844387076, 1.000000000000000000, 0.8660254037844387076, 1.000000000000000000, 0.8660254037844387076, 1.000000000000000000, 0.8660254037844387076, 1.000000000000000000, 0.8660254037844387076, 1.000000000000000000, 0.8660254037844387076, 1.000000000000000000 ) ) 
 REPRESENTATION_ITEM ( '' )  );
#16809=AXIS2_PLACEMENT_3D ( 'NONE', #6816, #6425, #9031 ) ;
#16810=CARTESIAN_POINT ( 'NONE',  ( 1.878215178125000939, 29.11562499938548498, 12.25316411605952283 ) ) ;
#16811=AXIS2_PLACEMENT_3D ( 'NONE', #13226, #9690, #23417 ) ;
#16814=CARTESIAN_POINT ( 'NONE',  ( 18.96682627828696610, 17.45107675043485429, 12.99999999999999467 ) ) ;
#16818=CARTESIAN_POINT ( 'NONE',  ( -3.756430356250003655, -28.29062499938548569, 8.999999999999992895 ) ) ;
#16821=CARTESIAN_POINT ( 'NONE',  ( 1.952783444825901382, 29.93753283725207481, 12.50294890599017172 ) ) ;
#16829=CARTESIAN_POINT ( 'NONE',  ( -2.672651547586948120E-15, -27.39062499938548356, 13.33755215474603162 ) ) ;
#16839=LINE ( 'NONE', #622, #12111 ) ;
#16844=CARTESIAN_POINT ( 'NONE',  ( 3.756430356250003655, 25.59062499938548285, 8.999999999999992895 ) ) ;
#16845=CARTESIAN_POINT ( 'NONE',  ( 3.834746474454188013E-15, 25.56250000000000000, 4.999999999999992006 ) ) ;
#16846=CARTESIAN_POINT ( 'NONE',  ( 20.79777820164935775, 15.14092395215691234, 11.30940107675849760 ) ) ;
#16847=CARTESIAN_POINT ( 'NONE',  ( 18.41350252340144422, 18.41350252340138383, 13.33755215474602984 ) ) ;
#16852=CARTESIAN_POINT ( 'NONE',  ( 18.49305203628493643, 18.49305203628486183, 4.662447845253954171 ) ) ;
#16856=CARTESIAN_POINT ( 'NONE',  ( -1.999999999999998224, 27.49374999877096926, 12.46410161513774639 ) ) ;
#16857=CARTESIAN_POINT ( 'NONE',  ( -1.878215178125004048, -29.26562499938548356, 5.746835883940462963 ) ) ;
#16858=CARTESIAN_POINT ( 'NONE',  ( -1.999999999999998224, 25.30000000000000426, 12.46410161513774639 ) ) ;
#16859=ORIENTED_EDGE ( 'NONE', *, *, #2432, .T. ) ;
#16862=ORIENTED_EDGE ( 'NONE', *, *, #14086, .F. ) ;
#16863=CARTESIAN_POINT ( 'NONE',  ( -2.672651547586948120E-15, -26.37812499938548427, 13.33755215474602984 ) ) ;
#16868=AXIS2_PLACEMENT_3D ( 'NONE', #14388, #14504, #24443 ) ;
#16872=EDGE_CURVE ( 'NONE', #16293, #1927, #16808, .T. ) ;
#16874=CARTESIAN_POINT ( 'NONE',  ( -1.878215178124998497, 28.59062499938548285, 12.25316411605951927 ) ) ;
#16879=CARTESIAN_POINT ( 'NONE',  ( 16.87775498257738960, 22.53460923206970179, 8.999999999999992895 ) ) ;
#16883=CARTESIAN_POINT ( 'NONE',  ( -3.756430356250002323, -26.56562499938548427, 11.16877607737301226 ) ) ;
#16885=CARTESIAN_POINT ( 'NONE',  ( 25.99307600111999150, 0.6000000000000000888, 20.00001200000000168 ) ) ;
#16888=CARTESIAN_POINT ( 'NONE',  ( 3.180741987853693331, -29.83126030492351788, 11.43940974718624837 ) ) ;
#16889=VERTEX_POINT ( 'NONE', #21111 ) ;
#16895=EDGE_LOOP ( 'NONE', ( #21229, #10916, #23334, #23892 ) ) ;
#16897=CARTESIAN_POINT ( 'NONE',  ( -2.000000000000003997, -27.77500000000000213, 5.535898384862238508 ) ) ;
#16899=ORIENTED_EDGE ( 'NONE', *, *, #11563, .F. ) ;
#16901=CARTESIAN_POINT ( 'NONE',  ( -1.878215178124998497, 28.70312499938548356, 12.25316411605951927 ) ) ;
#16905=CARTESIAN_POINT ( 'NONE',  ( -4.000000000000003553, -25.43124999877097281, 6.690598923241489970 ) ) ;
#16907=EDGE_CURVE ( 'NONE', #15184, #22241, #17931, .T. ) ;
#16908=CARTESIAN_POINT ( 'NONE',  ( -11.52193136556784658, -23.36965697125209118, 20.00001200000000168 ) ) ;
#16910=CARTESIAN_POINT ( 'NONE',  ( 30.00000000000000355, 3.673940397442059967E-15, 0.000000000000000000 ) ) ;
#16911=FACE_OUTER_BOUND ( 'NONE', #17210, .T. ) ;
#16915=DIRECTION ( 'NONE',  ( -0.7071067811865487940, -0.7071067811865463515, -0.000000000000000000 ) ) ;
#16916=CARTESIAN_POINT ( 'NONE',  ( -3.834746474454188013E-15, -26.01249999999999574, 4.999999999999992006 ) ) ;
#16917=ORIENTED_EDGE ( 'NONE', *, *, #7830, .T. ) ;
#16922=CARTESIAN_POINT ( 'NONE',  ( 3.756430356249995661, -26.34062499938548285, 6.831223922626973533 ) ) ;
#16929=CARTESIAN_POINT ( 'NONE',  ( 17.43018215624843847, 20.25860928099455904, 12.46410161513774639 ) ) ;
#16930=CARTESIAN_POINT ( 'NONE',  ( 22.39552511608559371, 17.08313036016677700, 11.16877607737301226 ) ) ;
#16931=ADVANCED_FACE ( 'NONE', ( #20007 ), #9467, .F. ) ;
#16933=CARTESIAN_POINT ( 'NONE',  ( 3.735045420075836212E-15, 29.30312499938548498, 4.662447845253954171 ) ) ;
#16935=CARTESIAN_POINT ( 'NONE',  ( 16.65886629145492748, 21.97126104737360563, 11.16877607737301048 ) ) ;
#16939=CARTESIAN_POINT ( 'NONE',  ( -3.756430356250002323, -27.35312499938547859, 11.16877607737301403 ) ) ;
#16947=( BOUNDED_SURFACE ( )  B_SPLINE_SURFACE ( 1, 2, ( 
 ( #25859, #4019, #23906, #2202, #11985, #19577, #3899, #9657, #18029, #1818, #19959, #10162, #1680, #9782, #17762, #25731, #13838, #11870, #19837, #1938, #2322, #12651, #14364, #8332, #16457, #4528, #24289, #18274, #22324, #4286, #6374, #501, #24419, #10280, #16575, #24672, #12509, #20483, #6760, #12258, #24148, #20226, #745, #237, #8471, #4671, #8208, #361, #22199, #10797, #22448, #14745, #2581, #16320, #22589, #16181, #10403, #14481, #22724, #6496, #4804, #6238, #10545, #18544, #14228, #12381, #6619, #626, #4405, #12779, #8593, #14608, #24534, #20346, #2443, #18403, #20623, #2706, #2829, #10667, #18658, #8714, #16701, #20750, #25318, #19300, #20880, #7281, #3480, #24931, #14871, #1258, #25061, #5309, #7150, #1399, #12904, #7397, #21020, #7010, #9372, #11320, #3344, #1125, #22846, #21401, #5062, #13287, #14996, #4919, #17353, #15377, #23349, #24809, #13041, #5438, #23225, #21263, #13429, #18789, #2968 ),
 ( #10935, #16964, #19042, #17089, #18926, #9242, #876, #23109, #5191, #8859, #1010, #16846, #8987, #6888, #22975, #9100, #3097, #11064, #15140, #13169, #21138, #3211, #11181, #19165, #17231, #15258, #25203, #21641, #25703, #17992, #9752, #82, #22029, #11706, #21781, #9486, #23611, #17855, #5818, #19426, #8053, #19809, #25827, #1785, #21520, #9620, #17599, #1911, #7662, #14063, #25577, #15645, #9871, #5574, #1644, #16036, #11957, #13553, #7911, #11453, #5691, #7523, #15898, #13670, #17732, #3601, #1517, #23998, #23871, #6077, #23488, #3724, #7783, #25439, #11571, #17467, #19684, #15764, #15520, #3865, #23730, #2029, #13802, #19541, #11838, #5956, #13941, #21908, #3990, #19926, #9998, #18132, #16427, #717, #14455, #24392, #2168, #12619, #20317, #8566, #325, #10249, #18513, #4636, #6340, #14576, #18244, #20593, #4497, #2292, #8300, #16668, #16287, #8439, #24253, #20448, #16549, #206, #10369, #468, #14716 ) ),
 .UNSPECIFIED., .F., .F., .F. ) 
 B_SPLINE_SURFACE_WITH_KNOTS ( ( 2, 2 ),
 ( 3, 2, 2, 2, 2, 2, 2, 2, 2, 2, 2, 2, 2, 2, 2, 2, 2, 2, 2, 2, 2, 2, 2, 2, 2, 2, 2, 2, 2, 2, 2, 2, 2, 2, 2, 2, 2, 2, 2, 2, 2, 2, 2, 2, 2, 2, 2, 2, 2, 2, 2, 2, 2, 2, 2, 2, 2, 2, 2, 2, 3 ),
 ( 0.000000000000000000, 1.000000000000000000 ),
 ( 0.000000000000000000, 0.01666666666666666644, 0.03333333333333333287, 0.05000000000000000278, 0.06666666666666666574, 0.08333333333333332871, 0.1000000000000000056, 0.1166666666666666685, 0.1333333333333333315, 0.1499999999999999944, 0.1666666666666666574, 0.1833333333333333204, 0.2000000000000000111, 0.2166666666666666741, 0.2333333333333333370, 0.2500000000000000000, 0.2666666666666666630, 0.2833333333333333259, 0.2999999999999999889, 0.3166666666666666519, 0.3333333333333333148, 0.3499999999999999778, 0.3666666666666666408, 0.3833333333333333592, 0.4000000000000000222, 0.4166666666666666852, 0.4333333333333333481, 0.4500000000000000111, 0.4666666666666666741, 0.4833333333333333370, 0.5000000000000000000, 0.5166666666666667185, 0.5333333333333333259, 0.5500000000000000444, 0.5666666666666666519, 0.5833333333333333703, 0.5999999999999999778, 0.6166666666666666963, 0.6333333333333333037, 0.6500000000000000222, 0.6666666666666666297, 0.6833333333333333481, 0.6999999999999999556, 0.7166666666666666741, 0.7333333333333332815, 0.7500000000000000000, 0.7666666666666667185, 0.7833333333333333259, 0.8000000000000000444, 0.8166666666666666519, 0.8333333333333333703, 0.8499999999999999778, 0.8666666666666666963, 0.8833333333333333037, 0.9000000000000000222, 0.9166666666666666297, 0.9333333333333333481, 0.9499999999999999556, 0.9666666666666666741, 0.9833333333333332815, 1.000000000000000000 ),
 .UNSPECIFIED. ) 
 GEOMETRIC_REPRESENTATION_ITEM ( )  RATIONAL_B_SPLINE_SURFACE ( (
 ( 1.000000000000000000, 0.8660254037844387076, 1.000000000000000000, 0.8660254037844387076, 1.000000000000000000, 0.8660254037844387076, 1.000000000000000000, 0.8660254037844387076, 1.000000000000000000, 0.8660254037844387076, 1.000000000000000000, 0.8660254037844387076, 1.000000000000000000, 0.8660254037844387076, 1.000000000000000000, 0.8660254037844387076, 1.000000000000000000, 0.8660254037844387076, 1.000000000000000000, 0.8660254037844387076, 1.000000000000000000, 0.8660254037844387076, 1.000000000000000000, 0.8660254037844387076, 1.000000000000000000, 0.8660254037844387076, 1.000000000000000000, 0.8660254037844387076, 1.000000000000000000, 0.8660254037844387076, 1.000000000000000000, 0.8660254037844387076, 1.000000000000000000, 0.8660254037844387076, 1.000000000000000000, 0.8660254037844387076, 1.000000000000000000, 0.8660254037844387076, 1.000000000000000000, 0.8660254037844387076, 1.000000000000000000, 0.8660254037844387076, 1.000000000000000000, 0.8660254037844387076, 1.000000000000000000, 0.8660254037844387076, 1.000000000000000000, 0.8660254037844387076, 1.000000000000000000, 0.8660254037844387076, 1.000000000000000000, 0.8660254037844387076, 1.000000000000000000, 0.8660254037844387076, 1.000000000000000000, 0.8660254037844387076, 1.000000000000000000, 0.8660254037844387076, 1.000000000000000000, 0.8660254037844387076, 1.000000000000000000, 0.8660254037844387076, 1.000000000000000000, 0.8660254037844387076, 1.000000000000000000, 0.8660254037844387076, 1.000000000000000000, 0.8660254037844387076, 1.000000000000000000, 0.8660254037844387076, 1.000000000000000000, 0.8660254037844387076, 1.000000000000000000, 0.8660254037844387076, 1.000000000000000000, 0.8660254037844387076, 1.000000000000000000, 0.8660254037844387076, 1.000000000000000000, 0.8660254037844387076, 1.000000000000000000, 0.8660254037844387076, 1.000000000000000000, 0.8660254037844387076, 1.000000000000000000, 0.8660254037844387076, 1.000000000000000000, 0.8660254037844387076, 1.000000000000000000, 0.8660254037844387076, 1.000000000000000000, 0.8660254037844387076, 1.000000000000000000, 0.8660254037844387076, 1.000000000000000000, 0.8660254037844387076, 1.000000000000000000, 0.8660254037844387076, 1.000000000000000000, 0.8660254037844387076, 1.000000000000000000, 0.8660254037844387076, 1.000000000000000000, 0.8660254037844387076, 1.000000000000000000, 0.8660254037844387076, 1.000000000000000000, 0.8660254037844387076, 1.000000000000000000, 0.8660254037844387076, 1.000000000000000000, 0.8660254037844387076, 1.000000000000000000, 0.8660254037844387076, 1.000000000000000000, 0.8660254037844387076, 1.000000000000000000, 0.8660254037844387076, 1.000000000000000000, 0.8660254037844387076, 1.000000000000000000),
 ( 1.000000000000000000, 0.8660254037844387076, 1.000000000000000000, 0.8660254037844387076, 1.000000000000000000, 0.8660254037844387076, 1.000000000000000000, 0.8660254037844387076, 1.000000000000000000, 0.8660254037844387076, 1.000000000000000000, 0.8660254037844387076, 1.000000000000000000, 0.8660254037844387076, 1.000000000000000000, 0.8660254037844387076, 1.000000000000000000, 0.8660254037844387076, 1.000000000000000000, 0.8660254037844387076, 1.000000000000000000, 0.8660254037844387076, 1.000000000000000000, 0.8660254037844387076, 1.000000000000000000, 0.8660254037844387076, 1.000000000000000000, 0.8660254037844387076, 1.000000000000000000, 0.8660254037844387076, 1.000000000000000000, 0.8660254037844387076, 1.000000000000000000, 0.8660254037844387076, 1.000000000000000000, 0.8660254037844387076, 1.000000000000000000, 0.8660254037844387076, 1.000000000000000000, 0.8660254037844387076, 1.000000000000000000, 0.8660254037844387076, 1.000000000000000000, 0.8660254037844387076, 1.000000000000000000, 0.8660254037844387076, 1.000000000000000000, 0.8660254037844387076, 1.000000000000000000, 0.8660254037844387076, 1.000000000000000000, 0.8660254037844387076, 1.000000000000000000, 0.8660254037844387076, 1.000000000000000000, 0.8660254037844387076, 1.000000000000000000, 0.8660254037844387076, 1.000000000000000000, 0.8660254037844387076, 1.000000000000000000, 0.8660254037844387076, 1.000000000000000000, 0.8660254037844387076, 1.000000000000000000, 0.8660254037844387076, 1.000000000000000000, 0.8660254037844387076, 1.000000000000000000, 0.8660254037844387076, 1.000000000000000000, 0.8660254037844387076, 1.000000000000000000, 0.8660254037844387076, 1.000000000000000000, 0.8660254037844387076, 1.000000000000000000, 0.8660254037844387076, 1.000000000000000000, 0.8660254037844387076, 1.000000000000000000, 0.8660254037844387076, 1.000000000000000000, 0.8660254037844387076, 1.000000000000000000, 0.8660254037844387076, 1.000000000000000000, 0.8660254037844387076, 1.000000000000000000, 0.8660254037844387076, 1.000000000000000000, 0.8660254037844387076, 1.000000000000000000, 0.8660254037844387076, 1.000000000000000000, 0.8660254037844387076, 1.000000000000000000, 0.8660254037844387076, 1.000000000000000000, 0.8660254037844387076, 1.000000000000000000, 0.8660254037844387076, 1.000000000000000000, 0.8660254037844387076, 1.000000000000000000, 0.8660254037844387076, 1.000000000000000000, 0.8660254037844387076, 1.000000000000000000, 0.8660254037844387076, 1.000000000000000000, 0.8660254037844387076, 1.000000000000000000, 0.8660254037844387076, 1.000000000000000000, 0.8660254037844387076, 1.000000000000000000, 0.8660254037844387076, 1.000000000000000000, 0.8660254037844387076, 1.000000000000000000) ) ) 
 REPRESENTATION_ITEM ( '' )  SURFACE ( )  );
#16948=CARTESIAN_POINT ( 'NONE',  ( -1.057460391440397258E-14, 29.55624999877096926, 4.999999999999992006 ) ) ;
#16951=CARTESIAN_POINT ( 'NONE',  ( -1.878215178125004048, -29.37812499938548783, 5.746835883940462963 ) ) ;
#16952=CARTESIAN_POINT ( 'NONE',  ( 23.69483382651587888, 18.38243907059705151, 8.999999999999992895 ) ) ;
#16953=( BOUNDED_CURVE ( )  B_SPLINE_CURVE ( 2, ( #19693, #25448, #7534, #13563, #1268, #3219, #15266, #21409, #5317 ),
 .UNSPECIFIED., .F., .F. ) 
 B_SPLINE_CURVE_WITH_KNOTS ( ( 3, 2, 2, 2, 3 ),
 ( 0.2750000000000000222, 0.2833333333333333259, 0.2999999999999999889, 0.3166666666666666519, 0.3250000000000000111 ),
 .UNSPECIFIED. ) 
 CURVE ( )  GEOMETRIC_REPRESENTATION_ITEM ( )  RATIONAL_B_SPLINE_CURVE ( ( 0.9330127018922194093, 0.9330127018922196314, 1.000000000000000000, 0.8660254037844387076, 1.000000000000000000, 0.8660254037844387076, 1.000000000000000000, 0.9330127018922191873, 0.9330127018922194093 ) ) 
 REPRESENTATION_ITEM ( '' )  );
#16961=EDGE_CURVE ( 'NONE', #8582, #125, #22130, .T. ) ;
#16962=CARTESIAN_POINT ( 'NONE',  ( 3.735045420075836212E-15, 27.95312499938548001, 4.662447845253954171 ) ) ;
#16963=CARTESIAN_POINT ( 'NONE',  ( 21.73911410323489690, 16.08225985374244615, 8.999999999999992895 ) ) ;
#16964=CARTESIAN_POINT ( 'NONE',  ( 20.53261315870440740, 14.87575890921195665, 6.690598923241489970 ) ) ;
#16965=CARTESIAN_POINT ( 'NONE',  ( 20.08631576820957321, 17.43011839025013288, 12.25316411605952283 ) ) ;
#16970=CARTESIAN_POINT ( 'NONE',  ( 16.87099832581089132, 22.18339308172956237, 8.999999999999992895 ) ) ;
#16971=CARTESIAN_POINT ( 'NONE',  ( 20.74032577480890183, 20.74032577480883077, 12.99999999999999289 ) ) ;
#16973=ORIENTED_EDGE ( 'NONE', *, *, #14358, .F. ) ;
#16975=CARTESIAN_POINT ( 'NONE',  ( 3.752267015613588906E-15, 28.20624999877096784, 4.381197846482986158 ) ) ;
#16976=CARTESIAN_POINT ( 'NONE',  ( 1.999999999999998224, -25.30000000000000426, 12.46410161513774639 ) ) ;
#16980=ORIENTED_EDGE ( 'NONE', *, *, #13131, .F. ) ;
#16981=CARTESIAN_POINT ( 'NONE',  ( 1.878215178124998497, -27.69062499938548427, 12.25316411605951927 ) ) ;
#16982=ORIENTED_EDGE ( 'NONE', *, *, #4922, .T. ) ;
#16983=ADVANCED_FACE ( 'NONE', ( #14522 ), #24579, .F. ) ;
#16985=CARTESIAN_POINT ( 'NONE',  ( 20.83968866226292249, 21.58177178539264318, 5.025996973432255821 ) ) ;
#16992=CARTESIAN_POINT ( 'NONE',  ( -1.878215178124995832, 28.44062499938548427, 5.746835883940462963 ) ) ;
#16994=DIRECTION ( 'NONE',  ( -0.7071067811865487940, -0.7071067811865463515, 0.000000000000000000 ) ) ;
#16998=CARTESIAN_POINT ( 'NONE',  ( 3.959305671612554781E-15, 30.00000000000000355, 12.99999999999999289 ) ) ;
#17001=CARTESIAN_POINT ( 'NONE',  ( 3.756430356249995661, -25.89062499938548356, 6.831223922626973533 ) ) ;
#17010=EDGE_CURVE ( 'NONE', #12604, #1927, #548, .T. ) ;
#17020=CARTESIAN_POINT ( 'NONE',  ( 3.756430356250003211, 29.34062499938548640, 6.831223922626973533 ) ) ;
#17023=CARTESIAN_POINT ( 'NONE',  ( 20.40224034548861809, 20.40224034548853638, 4.662447845253954171 ) ) ;
#17024=CARTESIAN_POINT ( 'NONE',  ( 2.672651547586948120E-15, 26.94062499938548783, 13.33755215474602984 ) ) ;
#17025=CARTESIAN_POINT ( 'NONE',  ( -25.16843286583315376, -6.741346781237213648, 20.00001200000000168 ) ) ;
#17033=CARTESIAN_POINT ( 'NONE',  ( -1.071796769724492338, -25.80759618943233491, 12.99999999999999467 ) ) ;
#17040=EDGE_CURVE ( 'NONE', #3427, #20732, #22639, .T. ) ;
#17041=ORIENTED_EDGE ( 'NONE', *, *, #15059, .F. ) ;
#17047=CARTESIAN_POINT ( 'NONE',  ( 1.071796769724481901, -27.56740381056766864, 12.99999999999999645 ) ) ;
#17050=DIRECTION ( 'NONE',  ( 0.000000000000000000, 0.000000000000000000, 1.000000000000000000 ) ) ;
#17051=CARTESIAN_POINT ( 'NONE',  ( 21.14924941424430571, 15.83685465832548900, 8.999999999999992895 ) ) ;
#17055=CARTESIAN_POINT ( 'NONE',  ( 4.000000000000003553, 25.90000000000000213, 8.999999999999992895 ) ) ;
#17056=CARTESIAN_POINT ( 'NONE',  ( 17.29526239452281899, 22.60765715044149715, 11.16877607737301048 ) ) ;
#17057=CARTESIAN_POINT ( 'NONE',  ( -3.469446951953614189E-15, -30.00000000000000355, 4.999999999999992006 ) ) ;
#17058=EDGE_LOOP ( 'NONE', ( #8161, #8769, #7612, #23 ) ) ;
#17060=CARTESIAN_POINT ( 'NONE',  ( 3.756430356249996105, -28.47812499938548569, 6.831223922626973533 ) ) ;
#17064=CARTESIAN_POINT ( 'NONE',  ( 2.205873879792267900, 29.91968208057595646, 12.34935938736416894 ) ) ;
#17067=ORIENTED_EDGE ( 'NONE', *, *, #20094, .F. ) ;
#17069=AXIS2_PLACEMENT_3D ( 'NONE', #3554, #5764, #13750 ) ;
#17075=FACE_OUTER_BOUND ( 'NONE', #25180, .T. ) ;
#17077=CARTESIAN_POINT ( 'NONE',  ( 22.41528496361359046, 16.75843071412113972, 8.999999999999992895 ) ) ;
#17079=ADVANCED_FACE ( 'NONE', ( #283 ), #6417, .F. ) ;
#17086=CARTESIAN_POINT ( 'NONE',  ( -3.756430356249996105, 26.22812499938548214, 6.831223922626973533 ) ) ;
#17089=CARTESIAN_POINT ( 'NONE',  ( 17.75721904254720940, 17.75721904254714545, 4.381197846482986158 ) ) ;
#17090=CARTESIAN_POINT ( 'NONE',  ( 21.12273290994980712, 15.81033815403099752, 11.16877607737301226 ) ) ;
#17094=CARTESIAN_POINT ( 'NONE',  ( 20.11283227250407180, 17.45663489454462436, 5.746835883940462963 ) ) ;
#17095=CARTESIAN_POINT ( 'NONE',  ( 23.64830241243857500, 17.99144816294611715, 8.999999999999992895 ) ) ;
#17096=ORIENTED_EDGE ( 'NONE', *, *, #3561, .T. ) ;
#17098=CARTESIAN_POINT ( 'NONE',  ( -1.999999999999995781, 28.69374999877096855, 5.535898384862237620 ) ) ;
#17099=CARTESIAN_POINT ( 'NONE',  ( -4.000000000000003553, -25.44999999999999929, 8.999999999999992895 ) ) ;
#17103=( BOUNDED_CURVE ( )  B_SPLINE_CURVE ( 2, ( #156, #20004, #13746, #20141, #21722, #21858, #1859, #5897, #23810 ),
 .UNSPECIFIED., .F., .F. ) 
 B_SPLINE_CURVE_WITH_KNOTS ( ( 3, 2, 2, 2, 3 ),
 ( 0.1250000000000000000, 0.1333333333333333315, 0.1499999999999999944, 0.1666666666666666574, 0.1749999999999999889 ),
 .UNSPECIFIED. ) 
 CURVE ( )  GEOMETRIC_REPRESENTATION_ITEM ( )  RATIONAL_B_SPLINE_CURVE ( ( 0.9330127018922194093, 0.9330127018922194093, 1.000000000000000000, 0.8660254037844387076, 1.000000000000000000, 0.8660254037844387076, 1.000000000000000000, 0.9330127018922194093, 0.9330127018922194093 ) ) 
 REPRESENTATION_ITEM ( '' )  );
#17106=CARTESIAN_POINT ( 'NONE',  ( -3.735045420075836212E-15, -29.30312499938548498, 4.662447845253954171 ) ) ;
#17109=CARTESIAN_POINT ( 'NONE',  ( 18.19544668900821094, 23.85216383888419855, 8.737301635141733414 ) ) ;
#17119=CARTESIAN_POINT ( 'NONE',  ( -1.071796769724495668, -27.15759618943233633, 12.99999999999999112 ) ) ;
#17123=DIRECTION ( 'NONE',  ( 0.000000000000000000, 0.000000000000000000, -1.000000000000000000 ) ) ;
#17128=CARTESIAN_POINT ( 'NONE',  ( -2.000000000000000888, -27.56874999877096855, 12.46410161513774817 ) ) ;
#17129=CARTESIAN_POINT ( 'NONE',  ( 3.756430356249995661, -28.59062499938548640, 6.831223922626973533 ) ) ;
#17140=ORIENTED_EDGE ( 'NONE', *, *, #2052, .T. ) ;
#17147=VECTOR ( 'NONE', #8788, 999.9999999999998863 ) ;
#17148=DIRECTION ( 'NONE',  ( -1.000000000000000000, 0.000000000000000000, 0.000000000000000000 ) ) ;
#17153=CARTESIAN_POINT ( 'NONE',  ( 22.97888821056449515, 17.66649345464567489, 8.999999999999992895 ) ) ;
#17155=FACE_OUTER_BOUND ( 'NONE', #14824, .T. ) ;
#17157=CARTESIAN_POINT ( 'NONE',  ( 4.000000000000001776, 28.50624999877096855, 11.30940107675849760 ) ) ;
#17158=AXIS2_PLACEMENT_3D ( 'NONE', #10101, #17960, #48 ) ;
#17168=CARTESIAN_POINT ( 'NONE',  ( 1.071796769724488563, -26.66740381056766651, 12.99999999999999289 ) ) ;
#17178=CARTESIAN_POINT ( 'NONE',  ( -3.756430356250002323, -25.66562499938548569, 11.16877607737301226 ) ) ;
#17179=ORIENTED_EDGE ( 'NONE', *, *, #25820, .F. ) ;
#17180=CARTESIAN_POINT ( 'NONE',  ( -3.999999999999997335, 28.86250000000000071, 11.30940107675849404 ) ) ;
#17182=CARTESIAN_POINT ( 'NONE',  ( 3.999999999999997335, -29.31250000000000000, 11.30940107675849404 ) ) ;
#17186=AXIS2_PLACEMENT_3D ( 'NONE', #3239, #9130, #17123 ) ;
#17189=CARTESIAN_POINT ( 'NONE',  ( -26.00000000000000355, -1.592040838891558504E-15, 20.00000599999999906 ) ) ;
#17190=CARTESIAN_POINT ( 'NONE',  ( 16.28763523133199342, 21.60002998725066448, 6.831223922626973533 ) ) ;
#17191=AXIS2_PLACEMENT_3D ( 'NONE', #19715, #6233, #2197 ) ;
#17194=CARTESIAN_POINT ( 'NONE',  ( -3.999999999999996447, 25.67500000000000071, 8.999999999999992895 ) ) ;
#17196=CARTESIAN_POINT ( 'NONE',  ( 16.92403133439988139, 22.23642609031855599, 6.831223922626973533 ) ) ;
#17197=CARTESIAN_POINT ( 'NONE',  ( 3.959305671612554781E-15, 30.00000000000000355, 12.99999999999999289 ) ) ;
#17199=VERTEX_POINT ( 'NONE', #5351 ) ;
#17203=CARTESIAN_POINT ( 'NONE',  ( 3.756430356249996105, -28.92812499938548498, 6.831223922626973533 ) ) ;
#17210=EDGE_LOOP ( 'NONE', ( #6544, #6779, #22110, #13629 ) ) ;
#17212=AXIS2_PLACEMENT_3D ( 'NONE', #6923, #22878, #24092 ) ;
#17215=CARTESIAN_POINT ( 'NONE',  ( -1.878215178125000939, -29.22812499938548569, 12.25316411605952283 ) ) ;
#17228=CARTESIAN_POINT ( 'NONE',  ( 3.469446951953614189E-15, 30.00000000000000355, 8.999999999999992895 ) ) ;
#17229=CARTESIAN_POINT ( 'NONE',  ( 3.756430356250003211, 26.97812499938547859, 6.831223922626973533 ) ) ;
#17230=LINE ( 'NONE', #1643, #6612 ) ;
#17231=CARTESIAN_POINT ( 'NONE',  ( 21.14249275747780032, 15.48563850798535491, 8.999999999999992895 ) ) ;
#17232=CARTESIAN_POINT ( 'NONE',  ( 21.17576591853879719, 15.86337116261998048, 6.831223922626973533 ) ) ;
#17235=CARTESIAN_POINT ( 'NONE',  ( 23.23716070179032656, 18.97547230650486938, 6.356741067357148722 ) ) ;
#17237=CARTESIAN_POINT ( 'NONE',  ( 21.27955846146187113, 18.62336108350243080, 12.25316411605952283 ) ) ;
#17238=CARTESIAN_POINT ( 'NONE',  ( 17.67766952966372429, 17.67766952966365679, 8.999999999999992895 ) ) ;
#17241=CARTESIAN_POINT ( 'NONE',  ( -3.756430356249995661, 26.34062499938548285, 6.831223922626973533 ) ) ;
#17242=CARTESIAN_POINT ( 'NONE',  ( -1.878215178125000939, -27.76562499938548356, 12.25316411605952283 ) ) ;
#17249=CARTESIAN_POINT ( 'NONE',  ( 3.756430356249997882, -27.65312499938548640, 11.16877607737301226 ) ) ;
#17257=DIRECTION ( 'NONE',  ( -0.000000000000000000, -0.000000000000000000, 1.000000000000000000 ) ) ;
#17259=CARTESIAN_POINT ( 'NONE',  ( 21.21320343559646915, 21.21320343559638744, 8.999999999999992895 ) ) ;
#17262=CARTESIAN_POINT ( 'NONE',  ( -1.952783444825901382, -29.93753283725207481, 12.50294890599017172 ) ) ;
#17263=CARTESIAN_POINT ( 'NONE',  ( -1.999999999999998224, 27.04374999877096641, 12.46410161513774639 ) ) ;
#17265=DIRECTION ( 'NONE',  ( 0.000000000000000000, 0.000000000000000000, 1.000000000000000000 ) ) ;
#17266=DIRECTION ( 'NONE',  ( -1.000000000000000000, 0.000000000000000000, 0.000000000000000000 ) ) ;
#17267=CARTESIAN_POINT ( 'NONE',  ( -3.735045420075836212E-15, -28.51562499938549067, 4.662447845253954171 ) ) ;
#17273=FACE_OUTER_BOUND ( 'NONE', #4325, .T. ) ;
#17290=CARTESIAN_POINT ( 'NONE',  ( -3.756430356249995661, 25.89062499938548356, 6.831223922626973533 ) ) ;
#17292=CARTESIAN_POINT ( 'NONE',  ( 21.05852382634284936, 21.05852382634277831, 12.99999999999999289 ) ) ;
#17294=CYLINDRICAL_SURFACE ( 'NONE', #12960, 4.000000000000000000 ) ;
#17297=CARTESIAN_POINT ( 'NONE',  ( -4.000000000000003553, -26.78124999877097068, 6.690598923241489970 ) ) ;
#17301=CARTESIAN_POINT ( 'NONE',  ( -3.369928719974892281E-15, -25.11250000000000426, 4.999999999999992006 ) ) ;
#17305=ORIENTED_EDGE ( 'NONE', *, *, #21354, .F. ) ;
#17310=ORIENTED_EDGE ( 'NONE', *, *, #21823, .T. ) ;
#17311=CARTESIAN_POINT ( 'NONE',  ( 1.878215178124995832, -29.00312499938548427, 5.746835883940462963 ) ) ;
#17313=VERTEX_POINT ( 'NONE', #1308 ) ;
#17315=ORIENTED_EDGE ( 'NONE', *, *, #18142, .T. ) ;
#17321=CARTESIAN_POINT ( 'NONE',  ( 19.28627369086489551, 21.94247106882419729, 12.25316411605951927 ) ) ;
#17322=DIRECTION ( 'NONE',  ( 0.000000000000000000, 0.000000000000000000, 1.000000000000000000 ) ) ;
#17324=CARTESIAN_POINT ( 'NONE',  ( -3.999999999999997335, 25.71250000000000213, 11.30940107675849404 ) ) ;
#17325=CARTESIAN_POINT ( 'NONE',  ( 19.36809667800328683, 19.36809667800321577, 13.33755215474603162 ) ) ;
#17328=VERTEX_POINT ( 'NONE', #7198 ) ;
#17331=ORIENTED_EDGE ( 'NONE', *, *, #24471, .F. ) ;
#17340=EDGE_LOOP ( 'NONE', ( #7355, #3013, #14732, #786 ) ) ;
#17342=CARTESIAN_POINT ( 'NONE',  ( -1.878215178125000939, -28.32812499938548711, 12.25316411605952283 ) ) ;
#17343=CARTESIAN_POINT ( 'NONE',  ( 5.577813053751546416E-15, 25.33750000000000213, 12.99999999999999289 ) ) ;
#17351=CARTESIAN_POINT ( 'NONE',  ( 1.878215178125004048, 27.46562499938548640, 5.746835883940462963 ) ) ;
#17353=CARTESIAN_POINT ( 'NONE',  ( 22.02202058170775345, 19.36582320374829891, 5.746835883940462963 ) ) ;
#17354=CARTESIAN_POINT ( 'NONE',  ( 17.90741546755112523, 20.56361284551042701, 5.746835883940462963 ) ) ;
#17355=CARTESIAN_POINT ( 'NONE',  ( 17.60253943329360382, 20.43096655803972084, 5.535898384862237620 ) ) ;
#17358=CARTESIAN_POINT ( 'NONE',  ( 18.81125008781888042, 18.81125008781880581, 4.662447845253954171 ) ) ;
#17359=CYLINDRICAL_SURFACE ( 'NONE', #12119, 4.000000000000000000 ) ;
#17362=CARTESIAN_POINT ( 'NONE',  ( -1.878215178124995832, 25.85312499938548569, 5.746835883940462963 ) ) ;
#17363=CARTESIAN_POINT ( 'NONE',  ( -3.752267015613588906E-15, -25.11250000000000071, 4.381197846482986158 ) ) ;
#17368=CARTESIAN_POINT ( 'NONE',  ( -1.878215178125004048, -28.36562499938548143, 5.746835883940462963 ) ) ;
#17379=CARTESIAN_POINT ( 'NONE',  ( -27.10000000000000497, -0.5999999999999998668, 19.00000000000000000 ) ) ;
#17381=LINE ( 'NONE', #16998, #12049 ) ;
#17387=DIRECTION ( 'NONE',  ( -0.000000000000000000, 1.000000000000000000, 0.000000000000000000 ) ) ;
#17389=CARTESIAN_POINT ( 'NONE',  ( -1.071796769724492338, -28.50759618943233775, 12.99999999999999467 ) ) ;
#17390=ORIENTED_EDGE ( 'NONE', *, *, #9072, .T. ) ;
#17393=CARTESIAN_POINT ( 'NONE',  ( 3.999999999999996447, -26.51874999877097139, 8.999999999999992895 ) ) ;
#17395=ORIENTED_EDGE ( 'NONE', *, *, #18302, .F. ) ;
#17396=ORIENTED_EDGE ( 'NONE', *, *, #10383, .T. ) ;
#17401=DIRECTION ( 'NONE',  ( 0.000000000000000000, 0.000000000000000000, -1.000000000000000000 ) ) ;
#17407=( NAMED_UNIT ( * ) PLANE_ANGLE_UNIT ( ) SI_UNIT ( $, .RADIAN. ) );
#17408=CARTESIAN_POINT ( 'NONE',  ( -1.878215178124995832, 27.20312499938548711, 5.746835883940462963 ) ) ;
#17409=EDGE_CURVE ( 'NONE', #7828, #13988, #9605, .T. ) ;
#17413=DIRECTION ( 'NONE',  ( 0.000000000000000000, -1.000000000000000000, 0.000000000000000000 ) ) ;
#17416=CARTESIAN_POINT ( 'NONE',  ( -4.000000000000003553, -25.84374999877096712, 8.999999999999992895 ) ) ;
#17419=LINE ( 'NONE', #22695, #12465 ) ;
#17420=CARTESIAN_POINT ( 'NONE',  ( -1.071796769724494558, -25.99240381056766580, 4.999999999999992895 ) ) ;
#17427=CARTESIAN_POINT ( 'NONE',  ( -2.672651547586948120E-15, -29.19062499938548783, 13.33755215474602984 ) ) ;
#17429=CARTESIAN_POINT ( 'NONE',  ( -1.057460391440397258E-14, 28.71250000000000213, 4.999999999999992006 ) ) ;
#17432=CARTESIAN_POINT ( 'NONE',  ( 20.10392967174102097, 20.10392967174092860, 12.99999999999999289 ) ) ;
#17433=EDGE_CURVE ( 'NONE', #10990, #19250, #18349, .T. ) ;
#17436=CARTESIAN_POINT ( 'NONE',  ( 20.64088888413906986, 20.64088888413900236, 13.33755215474602984 ) ) ;
#17438=CARTESIAN_POINT ( 'NONE',  ( -1.999999999999995781, 26.95000000000000284, 5.535898384862237620 ) ) ;
#17439=CARTESIAN_POINT ( 'NONE',  ( 15.70427213685309020, 21.01666689277176658, 11.16877607737301048 ) ) ;
#17449=ORIENTED_EDGE ( 'NONE', *, *, #16510, .T. ) ;
#17450=ORIENTED_EDGE ( 'NONE', *, *, #11626, .F. ) ;
#17452=CARTESIAN_POINT ( 'NONE',  ( -1.859271017917182139E-15, -29.78124999877096712, 12.99999999999999289 ) ) ;
#17459=EDGE_CURVE ( 'NONE', #3291, #24428, #12284, .T. ) ;
#17460=CARTESIAN_POINT ( 'NONE',  ( 1.878215178125000939, 28.21562499938548640, 12.25316411605952283 ) ) ;
#17462=CARTESIAN_POINT ( 'NONE',  ( 21.21320343559646915, 21.21320343559638744, 4.999999999999992006 ) ) ;
#17463=LINE ( 'NONE', #19039, #10484 ) ;
#17465=CARTESIAN_POINT ( 'NONE',  ( -3.756430356249997438, 26.75312499938548427, 11.16877607737301048 ) ) ;
#17466=CARTESIAN_POINT ( 'NONE',  ( -3.469446951953614189E-15, -30.00000000000000355, 4.999999999999992006 ) ) ;
#17467=CARTESIAN_POINT ( 'NONE',  ( 19.66640735175089461, 19.66640735175081645, 4.381197846482986158 ) ) ;
#17468=CARTESIAN_POINT ( 'NONE',  ( 17.58694394176227149, 22.89933869768094610, 8.999999999999992895 ) ) ;
#17472=DIRECTION ( 'NONE',  ( 0.000000000000000000, 0.000000000000000000, 1.000000000000000000 ) ) ;
#17474=CARTESIAN_POINT ( 'NONE',  ( 19.44764619088677904, 19.44764619088670088, 4.662447845253954171 ) ) ;
#17478=CARTESIAN_POINT ( 'NONE',  ( -2.000000000000003997, -25.97500000000000142, 5.535898384862238508 ) ) ;
#17480=ORIENTED_EDGE ( 'NONE', *, *, #14772, .F. ) ;
#17484=CARTESIAN_POINT ( 'NONE',  ( 3.756430356249995661, -28.02812499938548640, 6.831223922626973533 ) ) ;
#17486=EDGE_LOOP ( 'NONE', ( #19816, #19555 ) ) ;
#17493=CARTESIAN_POINT ( 'NONE',  ( 3.137519842735244810E-15, -27.30624999877096926, 4.999999999999991118 ) ) ;
#17499=DIRECTION ( 'NONE',  ( 0.000000000000000000, 1.000000000000000000, 0.000000000000000000 ) ) ;
#17503=CARTESIAN_POINT ( 'NONE',  ( -1.878215178125000939, -29.67812499938548498, 12.25316411605952283 ) ) ;
#17507=AXIS2_PLACEMENT_3D ( 'NONE', #3605, #13808, #25322 ) ;
#17509=CARTESIAN_POINT ( 'NONE',  ( 4.000000000000003553, 28.99374999877096926, 8.999999999999992895 ) ) ;
#17513=CARTESIAN_POINT ( 'NONE',  ( -1.071796769724491227, -26.44240381056766509, 4.999999999999989342 ) ) ;
#17516=CIRCLE ( 'NONE', #6225, 0.7500000000000001110 ) ;
#17521=ORIENTED_EDGE ( 'NONE', *, *, #44, .F. ) ;
#17531=SHAPE_REPRESENTATION_RELATIONSHIP ( 'NONE' , 'NONE' ,  #16033, #14134 ) ;
#17532=CARTESIAN_POINT ( 'NONE',  ( 1.878215178125000939, 27.87812499938548427, 12.25316411605952283 ) ) ;
#17534=CARTESIAN_POINT ( 'NONE',  ( -1.071796769724495668, -26.65134618820330203, 12.99999999999999112 ) ) ;
#17542=CARTESIAN_POINT ( 'NONE',  ( -2.000000000000003997, -26.36874999877096926, 5.535898384862238508 ) ) ;
#17543=CARTESIAN_POINT ( 'NONE',  ( -3.756430356249995661, 28.14062499938548356, 6.831223922626973533 ) ) ;
#17555=CARTESIAN_POINT ( 'NONE',  ( -3.756430356250002323, -27.01562499938548356, 11.16877607737301226 ) ) ;
#17557=VERTEX_POINT ( 'NONE', #14107 ) ;
#17559=ADVANCED_FACE ( 'NONE', ( #10559 ), #22071, .T. ) ;
#17566=CARTESIAN_POINT ( 'NONE',  ( 23.69483382651587888, 18.38243907059705151, 8.999999999999992895 ) ) ;
#17570=CARTESIAN_POINT ( 'NONE',  ( 4.000000000000001776, 28.56249999999999645, 11.30940107675849760 ) ) ;
#17573=DIRECTION ( 'NONE',  ( 0.000000000000000000, 0.000000000000000000, 1.000000000000000000 ) ) ;
#17575=ORIENTED_EDGE ( 'NONE', *, *, #15019, .T. ) ;
#17578=ORIENTED_EDGE ( 'NONE', *, *, #8912, .T. ) ;
#17582=CARTESIAN_POINT ( 'NONE',  ( -3.999999999999996447, 27.41874999877096641, 8.999999999999992895 ) ) ;
#17594=CARTESIAN_POINT ( 'NONE',  ( -3.756430356249997882, 29.45312499938548356, 11.16877607737301226 ) ) ;
#17596=DIRECTION ( 'NONE',  ( -1.000000000000000000, 0.000000000000000000, 0.000000000000000000 ) ) ;
#17597=CARTESIAN_POINT ( 'NONE',  ( -3.756430356249996994, 28.96562499938548285, 8.999999999999992895 ) ) ;
#17598=CARTESIAN_POINT ( 'NONE',  ( -3.013468763610312351, -29.84883905190463338, 6.356741067357151387 ) ) ;
#17599=CARTESIAN_POINT ( 'NONE',  ( 20.31164228958361306, 17.48321516483735394, 12.46410161513774817 ) ) ;
#17600=CARTESIAN_POINT ( 'NONE',  ( 20.00449278107117834, 20.00449278107111084, 13.33755215474602984 ) ) ;
#17605=EDGE_CURVE ( 'NONE', #18353, #18087, #2585, .T. ) ;
#17606=CARTESIAN_POINT ( 'NONE',  ( 21.59775651299582222, 18.94155913503637478, 12.25316411605952283 ) ) ;
#17607=CARTESIAN_POINT ( 'NONE',  ( 3.469446951953614189E-15, 30.00000000000000355, 4.999999999999992006 ) ) ;
#17610=CARTESIAN_POINT ( 'NONE',  ( 3.999999999999997335, -26.16250000000000142, 11.30940107675849404 ) ) ;
#17617=CARTESIAN_POINT ( 'NONE',  ( -24.67207871933484498, 8.377607117416790317, 20.00001200000000523 ) ) ;
#17618=CARTESIAN_POINT ( 'NONE',  ( 2.000000000000000888, 26.21874999877096712, 12.46410161513774817 ) ) ;
#17627=ADVANCED_FACE ( 'NONE', ( #12666 ), #20637, .F. ) ;
#17637=CARTESIAN_POINT ( 'NONE',  ( -1.057460391440397258E-14, 28.71250000000000213, 4.999999999999992006 ) ) ;
#17643=CARTESIAN_POINT ( 'NONE',  ( 3.974064950101062088, 29.73565934716929959, 8.475804415688518390 ) ) ;
#17644=AXIS2_PLACEMENT_3D ( 'NONE', #21545, #1151, #9127 ) ;
#17648=CARTESIAN_POINT ( 'NONE',  ( -3.999999999999997335, 26.55624999877096570, 11.30940107675849404 ) ) ;
#17651=AXIS2_PLACEMENT_3D ( 'NONE', #85, #22419, #12475 ) ;
#17655=ORIENTED_EDGE ( 'NONE', *, *, #1970, .F. ) ;
#17656=EDGE_CURVE ( 'NONE', #10748, #1228, #10600, .T. ) ;
#17658=ORIENTED_EDGE ( 'NONE', *, *, #12460, .T. ) ;
#17660=VERTEX_POINT ( 'NONE', #13300 ) ;
#17666=DIRECTION ( 'NONE',  ( -0.000000000000000000, -0.000000000000000000, -1.000000000000000000 ) ) ;
#17668=CIRCLE ( 'NONE', #20153, 4.000000000000000000 ) ;
#17671=CARTESIAN_POINT ( 'NONE',  ( 3.735045420075836212E-15, 28.51562499938549067, 4.662447845253954171 ) ) ;
#17672=CARTESIAN_POINT ( 'NONE',  ( -4.000000000000003553, -26.74374999877096926, 8.999999999999992895 ) ) ;
#17676=CARTESIAN_POINT ( 'NONE',  ( -4.000000000000003553, -25.84374999877096712, 8.999999999999992895 ) ) ;
#17679=CARTESIAN_POINT ( 'NONE',  ( 3.999999999999997335, -26.55624999877096926, 11.30940107675849404 ) ) ;
#17680=CARTESIAN_POINT ( 'NONE',  ( 3.756430356250003655, 27.05312499938548498, 8.999999999999992895 ) ) ;
#17683=LINE ( 'NONE', #6148, #2879 ) ;
#17691=CARTESIAN_POINT ( 'NONE',  ( -1.878215178125004048, -28.02812499938548640, 5.746835883940462963 ) ) ;
#17703=CARTESIAN_POINT ( 'NONE',  ( 17.29526239452281899, 22.60765715044149715, 11.16877607737301226 ) ) ;
#17706=CARTESIAN_POINT ( 'NONE',  ( 2.000000000000000888, 28.52500000000000213, 12.46410161513774817 ) ) ;
#17708=CARTESIAN_POINT ( 'NONE',  ( 23.69483382651587888, 18.38243907059705151, 8.999999999999992895 ) ) ;
#17709=CARTESIAN_POINT ( 'NONE',  ( -1.071796769724492338, -29.35134618820330488, 12.99999999999999467 ) ) ;
#17713=VERTEX_POINT ( 'NONE', #15152 ) ;
#17715=CARTESIAN_POINT ( 'NONE',  ( 18.51293941407127974, 18.51293941407120869, 12.99999999999999112 ) ) ;
#17718=CARTESIAN_POINT ( 'NONE',  ( 1.859271017917182139E-15, 28.88124999877096499, 12.99999999999999289 ) ) ;
#17727=CARTESIAN_POINT ( 'NONE',  ( 3.756430356250003655, 25.14062499938548356, 8.999999999999992895 ) ) ;
#17732=CARTESIAN_POINT ( 'NONE',  ( 17.96051224213834985, 20.78893936688446331, 5.535898384862237620 ) ) ;
#17733=CARTESIAN_POINT ( 'NONE',  ( 22.10384356884614121, 16.79144881292732450, 8.999999999999992895 ) ) ;
#17734=CARTESIAN_POINT ( 'NONE',  ( -3.213722874945784014, -29.82775332956657266, 11.39306173506716924 ) ) ;
#17736=CARTESIAN_POINT ( 'NONE',  ( 21.93836504211864025, 20.46399127338558799, 5.129272290912049392 ) ) ;
#17738=CARTESIAN_POINT ( 'NONE',  ( 19.42333939484895211, 16.59491227010269299, 5.535898384862238508 ) ) ;
#17741=CARTESIAN_POINT ( 'NONE',  ( -2.620986760973688460E-15, -27.13750000000000284, 13.61880215351699874 ) ) ;
#17756=EDGE_CURVE ( 'NONE', #24945, #8728, #14959, .T. ) ;
#17760=CARTESIAN_POINT ( 'NONE',  ( -1.999999999999998224, 26.64999999999999858, 12.46410161513774639 ) ) ;
#17762=CARTESIAN_POINT ( 'NONE',  ( 19.47643616943617317, 16.82023879147673284, 5.746835883940462963 ) ) ;
#17763=CARTESIAN_POINT ( 'NONE',  ( 21.12923450446149687, 15.47238025496904612, 6.690598923241489970 ) ) ;
#17769=FACE_OUTER_BOUND ( 'NONE', #16895, .T. ) ;
#17772=DIRECTION ( 'NONE',  ( -0.7071067811865487940, -0.7071067811865463515, 0.000000000000000000 ) ) ;
#17775=CARTESIAN_POINT ( 'NONE',  ( 3.137519842735244810E-15, -26.46249999999999858, 4.999999999999991118 ) ) ;
#17782=DIRECTION ( 'NONE',  ( 0.000000000000000000, 0.000000000000000000, -1.000000000000000000 ) ) ;
#17784=CARTESIAN_POINT ( 'NONE',  ( -1.626862140677534194E-14, -27.98124999877096997, 12.99999999999999289 ) ) ;
#17791=FILL_AREA_STYLE ('',( #1712 ) ) ;
#17792=CARTESIAN_POINT ( 'NONE',  ( 2.672651547586948120E-15, 27.39062499938548356, 13.33755215474602984 ) ) ;
#17801=CARTESIAN_POINT ( 'NONE',  ( 3.999999999999997335, -27.90624999877097068, 11.30940107675849404 ) ) ;
#17802=CARTESIAN_POINT ( 'NONE',  ( 3.756430356250004099, 27.99062499938548498, 6.831223922626973533 ) ) ;
#17803=DIRECTION ( 'NONE',  ( -0.7071067811865487940, -0.7071067811865463515, 0.000000000000000000 ) ) ;
#17806=ORIENTED_EDGE ( 'NONE', *, *, #6265, .F. ) ;
#17808=CARTESIAN_POINT ( 'NONE',  ( 4.000000000000003553, 25.39374999877096784, 8.999999999999992895 ) ) ;
#17811=CARTESIAN_POINT ( 'NONE',  ( 3.878215178125003604, 29.57031249969274356, 8.999999999999992895 ) ) ;
#17813=CARTESIAN_POINT ( 'NONE',  ( 1.878215178124998497, -27.80312499938548498, 12.25316411605951927 ) ) ;
#17814=ORIENTED_EDGE ( 'NONE', *, *, #22691, .F. ) ;
#17821=CARTESIAN_POINT ( 'NONE',  ( 18.86200962215296784, 21.51820700011226606, 5.746835883940462963 ) ) ;
#17823=CARTESIAN_POINT ( 'NONE',  ( 20.78010053211970032, 20.78010053211962926, 12.99999999999999289 ) ) ;
#17825=CARTESIAN_POINT ( 'NONE',  ( 3.752267015613588906E-15, 27.36250000000000071, 4.381197846482986158 ) ) ;
#17827=CARTESIAN_POINT ( 'NONE',  ( 21.46517399152334704, 18.80897661356389605, 5.746835883940462963 ) ) ;
#17828=CARTESIAN_POINT ( 'NONE',  ( 8.000000000000000000, 10.00000000000000000, 15.00000000000000178 ) ) ;
#17829=VERTEX_POINT ( 'NONE', #7794 ) ;
#17836=CARTESIAN_POINT ( 'NONE',  ( -1.999999999999998224, 29.29374999877096997, 12.46410161513774639 ) ) ;
#17850=CARTESIAN_POINT ( 'NONE',  ( -1.878215178124995832, 25.74062499938548498, 5.746835883940462963 ) ) ;
#17853=CYLINDRICAL_SURFACE ( 'NONE', #14707, 26.00000000000000355 ) ;
#17855=CARTESIAN_POINT ( 'NONE',  ( 21.48720731330624645, 15.83035306381379748, 6.690598923241489970 ) ) ;
#17856=CARTESIAN_POINT ( 'NONE',  ( 17.29526239452281899, 22.60765715044149715, 11.16877607737301226 ) ) ;
#17859=CARTESIAN_POINT ( 'NONE',  ( -3.756430356250003655, -25.59062499938548285, 8.999999999999992895 ) ) ;
#17860=EDGE_CURVE ( 'NONE', #1173, #18977, #11332, .T. ) ;
#17866=CARTESIAN_POINT ( 'NONE',  ( -4.000000000000003553, -27.25000000000000000, 8.999999999999992895 ) ) ;
#17871=CARTESIAN_POINT ( 'NONE',  ( 8.377607117416813409, 24.67207871933482366, 20.00001200000000523 ) ) ;
#17873=ORIENTED_EDGE ( 'NONE', *, *, #11379, .F. ) ;
#17874=ORIENTED_EDGE ( 'NONE', *, *, #3174, .T. ) ;
#17881=CARTESIAN_POINT ( 'NONE',  ( 26.00000000000000355, 3.184081677783117796E-15, 20.00001200000000168 ) ) ;
#17884=CARTESIAN_POINT ( 'NONE',  ( 18.35384038830430597, 18.35384038830423492, 4.999999999999992006 ) ) ;
#17887=CARTESIAN_POINT ( 'NONE',  ( 21.10271800016700183, 15.44586375067455464, 8.999999999999992895 ) ) ;
#17889=CARTESIAN_POINT ( 'NONE',  ( -27.10000000000000497, -0.5999999999999998668, 19.59999999999999787 ) ) ;
#17890=CARTESIAN_POINT ( 'NONE',  ( 3.594806220554922049, 29.78401552627944326, 7.226316032987424975 ) ) ;
#17892=CARTESIAN_POINT ( 'NONE',  ( 19.13727975771751488, 17.62153022986539241, 4.999999999999992895 ) ) ;
#17895=CARTESIAN_POINT ( 'NONE',  ( 4.000000000000003553, 27.23124999877096641, 6.690598923241489970 ) ) ;
#17898=VERTEX_POINT ( 'NONE', #13565 ) ;
#17903=ORIENTED_EDGE ( 'NONE', *, *, #6083, .T. ) ;
#17905=CARTESIAN_POINT ( 'NONE',  ( 3.137519842735244810E-15, -26.91249999999999787, 4.999999999999991118 ) ) ;
#17906=AXIS2_PLACEMENT_3D ( 'NONE', #9055, #10745, #20824 ) ;
#17913=CARTESIAN_POINT ( 'NONE',  ( 3.756430356250004099, 27.99062499938548498, 6.831223922626973533 ) ) ;
#17920=CARTESIAN_POINT ( 'NONE',  ( 1.071796769724487230, -25.71115380933864003, 12.99999999999999467 ) ) ;
#17922=CARTESIAN_POINT ( 'NONE',  ( -2.000000000000000888, -28.46874999877097068, 12.46410161513774817 ) ) ;
#17923=CARTESIAN_POINT ( 'NONE',  ( -3.756430356249996994, 27.27812499938548640, 8.999999999999992895 ) ) ;
#17926=CARTESIAN_POINT ( 'NONE',  ( 0.5000000000000001110, 10.00000000000000000, 13.00000000000000178 ) ) ;
#17930=CARTESIAN_POINT ( 'NONE',  ( -4.000000000000003553, -29.05000000000000071, 8.999999999999992895 ) ) ;
#17931=LINE ( 'NONE', #5413, #8320 ) ;
#17932=VERTEX_POINT ( 'NONE', #8692 ) ;
#17938=CARTESIAN_POINT ( 'NONE',  ( -3.756430356250002323, -26.45312499938548356, 11.16877607737301226 ) ) ;
#17941=( BOUNDED_CURVE ( )  B_SPLINE_CURVE ( 2, ( #16324, #504, #14484, #629, #14999 ),
 .UNSPECIFIED., .F., .F. ) 
 B_SPLINE_CURVE_WITH_KNOTS ( ( 3, 2, 3 ),
 ( 0.9749999999999999778, 0.9833333333333332815, 1.000000000000000000 ),
 .UNSPECIFIED. ) 
 CURVE ( )  GEOMETRIC_REPRESENTATION_ITEM ( )  RATIONAL_B_SPLINE_CURVE ( ( 0.9330127018922194093, 0.9330127018922194093, 1.000000000000000000, 0.8660254037844387076, 1.000000000000000000 ) ) 
 REPRESENTATION_ITEM ( '' )  );
#17947=CARTESIAN_POINT ( 'NONE',  ( 1.071796769724492338, 29.80134618820330417, 12.99999999999999467 ) ) ;
#17948=CARTESIAN_POINT ( 'NONE',  ( -3.756430356249996105, 27.24062499938548498, 6.831223922626973533 ) ) ;
#17952=CARTESIAN_POINT ( 'NONE',  ( 16.87099832581089132, 22.18339308172956237, 8.999999999999992895 ) ) ;
#17954=CYLINDRICAL_SURFACE ( 'NONE', #461, 4.000000000000000000 ) ;
#17958=CARTESIAN_POINT ( 'NONE',  ( -1.999999999999995781, 28.30000000000000071, 5.535898384862237620 ) ) ;
#17960=DIRECTION ( 'NONE',  ( 0.000000000000000000, 0.000000000000000000, -1.000000000000000000 ) ) ;
#17961=CARTESIAN_POINT ( 'NONE',  ( 18.19682354053567153, 23.50921829645434258, 6.831223922626973533 ) ) ;
#17967=CARTESIAN_POINT ( 'NONE',  ( 4.000000000000001776, 26.31250000000000000, 11.30940107675849760 ) ) ;
#17968=CARTESIAN_POINT ( 'NONE',  ( 4.000000000000003553, 29.89374999877096784, 8.999999999999992895 ) ) ;
#17971=CARTESIAN_POINT ( 'NONE',  ( 19.28502432982091008, 17.76927480196879472, 12.99999999999999112 ) ) ;
#17976=PRODUCT_DEFINITION ( 'UNKNOWN', '', #4788, #6797 ) ;
#17984=ADVANCED_FACE ( 'NONE', ( #20814 ), #2898, .F. ) ;
#17987=EDGE_CURVE ( 'NONE', #16614, #15499, #5945, .T. ) ;
#17988=CARTESIAN_POINT ( 'NONE',  ( 1.878215178125004048, 25.66562499938548569, 5.746835883940462963 ) ) ;
#17992=CARTESIAN_POINT ( 'NONE',  ( 15.61822102945791002, 21.27507527895022221, 6.690598923241487306 ) ) ;
#17995=CARTESIAN_POINT ( 'NONE',  ( -3.469446951953614189E-15, -30.00000000000000355, 8.999999999999992895 ) ) ;
#17996=CARTESIAN_POINT ( 'NONE',  ( -1.071796769724493448, 29.12634618820329990, 4.999999999999995559 ) ) ;
#17998=CARTESIAN_POINT ( 'NONE',  ( -3.735045420075836212E-15, -26.15312499938548285, 4.662447845253954171 ) ) ;
#17999=CARTESIAN_POINT ( 'NONE',  ( 19.41885621233737069, 22.07505359029666536, 5.746835883940462963 ) ) ;
#18000=EDGE_LOOP ( 'NONE', ( #3644, #7059, #7949, #25690 ) ) ;
#18002=CARTESIAN_POINT ( 'NONE',  ( 1.999999999999995781, -27.40000000000000213, 5.535898384862237620 ) ) ;
#18010=CARTESIAN_POINT ( 'NONE',  ( -1.878215178125000939, -29.56562499938548427, 12.25316411605952283 ) ) ;
#18015=ADVANCED_FACE ( 'NONE', ( #16911 ), #4994, .F. ) ;
#18017=( BOUNDED_SURFACE ( )  B_SPLINE_SURFACE ( 1, 2, ( 
 ( #24387, #594, #712, #8561, #6586, #12611, #201, #20587, #22023, #2675, #19010, #14958, #22687, #1362, #8816, #4772, #3061, #13252, #1092, #14710, #13134, #6854, #11030, #9068, #17051, #21221, #12744, #16807, #22934, #3305, #2793, #12861, #5019, #24773, #21103, #25022, #7244, #5275, #8957, #3181, #13002, #17190, #1221, #15224, #25162, #20982, #7110, #15096, #14838, #23190, #11278, #24629, #23073, #5158, #11147, #19128, #22812, #19262, #20839, #20713, #16663, #2929, #9200, #18889, #6716, #10758, #18748, #837, #4887, #10890, #976, #16930, #24900, #6978, #1749, #15859, #21876, #21609, #13522, #17703, #3687, #21492, #25671, #23829, #15613, #9455, #7489, #7366, #17821, #25542, #13763, #19780, #21742, #11418, #25786, #11541, #1877, #23449, #7871, #9719, #15478, #5538, #3958, #7751, #17321, #17436, #11667, #13904, #9580, #19507, #3826, #19893, #25402, #5398, #3568, #9839, #1607, #5918, #11924, #13387, #17566 ),
 ( #7626, #23579, #5660, #13640, #19643, #11805, #15734, #23696, #9337, #25284, #5777, #15343, #23312, #21365, #3445, #19391, #1484, #22514, #21997, #4595, #22380, #173, #22122, #22261, #8264, #14421, #16245, #2508, #4073, #8534, #14154, #18214, #14031, #16122, #24216, #6554, #12046, #24084, #295, #10092, #6434, #10335, #18475, #16515, #20160, #4463, #6303, #10474, #12438, #563, #24477, #14296, #4342, #12316, #2127, #14536, #12574, #9961, #430, #20284, #2381, #20406, #8144, #1992, #6166, #15999, #17952, #4208, #18332, #12187, #38, #8399, #16388, #20024, #8014, #23966, #6047, #24354, #18092, #2260, #10216, #1183, #7212, #3033, #15064, #6683, #23039, #5244, #4742, #22901, #18857, #684, #20554, #12715, #8650, #6950, #17153, #4987, #18597, #17023, #10726, #14928, #12967, #20949, #25124, #16629, #20682, #22781, #1066, #2765, #2645, #18982, #9163, #947, #15194, #18712, #8782, #14807, #10607, #9040, #5127 ) ),
 .UNSPECIFIED., .F., .F., .F. ) 
 B_SPLINE_SURFACE_WITH_KNOTS ( ( 2, 2 ),
 ( 3, 2, 2, 2, 2, 2, 2, 2, 2, 2, 2, 2, 2, 2, 2, 2, 2, 2, 2, 2, 2, 2, 2, 2, 2, 2, 2, 2, 2, 2, 2, 2, 2, 2, 2, 2, 2, 2, 2, 2, 2, 2, 2, 2, 2, 2, 2, 2, 2, 2, 2, 2, 2, 2, 2, 2, 2, 2, 2, 2, 3 ),
 ( 0.000000000000000000, 1.000000000000000000 ),
 ( 0.000000000000000000, 0.01666666666666666644, 0.03333333333333333287, 0.05000000000000000278, 0.06666666666666666574, 0.08333333333333332871, 0.1000000000000000056, 0.1166666666666666685, 0.1333333333333333315, 0.1499999999999999944, 0.1666666666666666574, 0.1833333333333333204, 0.2000000000000000111, 0.2166666666666666741, 0.2333333333333333370, 0.2500000000000000000, 0.2666666666666666630, 0.2833333333333333259, 0.2999999999999999889, 0.3166666666666666519, 0.3333333333333333148, 0.3499999999999999778, 0.3666666666666666408, 0.3833333333333333592, 0.4000000000000000222, 0.4166666666666666852, 0.4333333333333333481, 0.4500000000000000111, 0.4666666666666666741, 0.4833333333333333370, 0.5000000000000000000, 0.5166666666666667185, 0.5333333333333333259, 0.5500000000000000444, 0.5666666666666666519, 0.5833333333333333703, 0.5999999999999999778, 0.6166666666666666963, 0.6333333333333333037, 0.6500000000000000222, 0.6666666666666666297, 0.6833333333333333481, 0.6999999999999999556, 0.7166666666666666741, 0.7333333333333332815, 0.7500000000000000000, 0.7666666666666667185, 0.7833333333333333259, 0.8000000000000000444, 0.8166666666666666519, 0.8333333333333333703, 0.8499999999999999778, 0.8666666666666666963, 0.8833333333333333037, 0.9000000000000000222, 0.9166666666666666297, 0.9333333333333333481, 0.9499999999999999556, 0.9666666666666666741, 0.9833333333333332815, 1.000000000000000000 ),
 .UNSPECIFIED. ) 
 GEOMETRIC_REPRESENTATION_ITEM ( )  RATIONAL_B_SPLINE_SURFACE ( (
 ( 1.000000000000000000, 0.8660254037844387076, 1.000000000000000000, 0.8660254037844387076, 1.000000000000000000, 0.8660254037844387076, 1.000000000000000000, 0.8660254037844387076, 1.000000000000000000, 0.8660254037844387076, 1.000000000000000000, 0.8660254037844387076, 1.000000000000000000, 0.8660254037844387076, 1.000000000000000000, 0.8660254037844387076, 1.000000000000000000, 0.8660254037844387076, 1.000000000000000000, 0.8660254037844387076, 1.000000000000000000, 0.8660254037844387076, 1.000000000000000000, 0.8660254037844387076, 1.000000000000000000, 0.8660254037844387076, 1.000000000000000000, 0.8660254037844387076, 1.000000000000000000, 0.8660254037844387076, 1.000000000000000000, 0.8660254037844387076, 1.000000000000000000, 0.8660254037844387076, 1.000000000000000000, 0.8660254037844387076, 1.000000000000000000, 0.8660254037844387076, 1.000000000000000000, 0.8660254037844387076, 1.000000000000000000, 0.8660254037844387076, 1.000000000000000000, 0.8660254037844387076, 1.000000000000000000, 0.8660254037844387076, 1.000000000000000000, 0.8660254037844387076, 1.000000000000000000, 0.8660254037844387076, 1.000000000000000000, 0.8660254037844387076, 1.000000000000000000, 0.8660254037844387076, 1.000000000000000000, 0.8660254037844387076, 1.000000000000000000, 0.8660254037844387076, 1.000000000000000000, 0.8660254037844387076, 1.000000000000000000, 0.8660254037844387076, 1.000000000000000000, 0.8660254037844387076, 1.000000000000000000, 0.8660254037844387076, 1.000000000000000000, 0.8660254037844387076, 1.000000000000000000, 0.8660254037844387076, 1.000000000000000000, 0.8660254037844387076, 1.000000000000000000, 0.8660254037844387076, 1.000000000000000000, 0.8660254037844387076, 1.000000000000000000, 0.8660254037844387076, 1.000000000000000000, 0.8660254037844387076, 1.000000000000000000, 0.8660254037844387076, 1.000000000000000000, 0.8660254037844387076, 1.000000000000000000, 0.8660254037844387076, 1.000000000000000000, 0.8660254037844387076, 1.000000000000000000, 0.8660254037844387076, 1.000000000000000000, 0.8660254037844387076, 1.000000000000000000, 0.8660254037844387076, 1.000000000000000000, 0.8660254037844387076, 1.000000000000000000, 0.8660254037844387076, 1.000000000000000000, 0.8660254037844387076, 1.000000000000000000, 0.8660254037844387076, 1.000000000000000000, 0.8660254037844387076, 1.000000000000000000, 0.8660254037844387076, 1.000000000000000000, 0.8660254037844387076, 1.000000000000000000, 0.8660254037844387076, 1.000000000000000000, 0.8660254037844387076, 1.000000000000000000, 0.8660254037844387076, 1.000000000000000000, 0.8660254037844387076, 1.000000000000000000, 0.8660254037844387076, 1.000000000000000000, 0.8660254037844387076, 1.000000000000000000),
 ( 1.000000000000000000, 0.8660254037844387076, 1.000000000000000000, 0.8660254037844387076, 1.000000000000000000, 0.8660254037844387076, 1.000000000000000000, 0.8660254037844387076, 1.000000000000000000, 0.8660254037844387076, 1.000000000000000000, 0.8660254037844387076, 1.000000000000000000, 0.8660254037844387076, 1.000000000000000000, 0.8660254037844387076, 1.000000000000000000, 0.8660254037844387076, 1.000000000000000000, 0.8660254037844387076, 1.000000000000000000, 0.8660254037844387076, 1.000000000000000000, 0.8660254037844387076, 1.000000000000000000, 0.8660254037844387076, 1.000000000000000000, 0.8660254037844387076, 1.000000000000000000, 0.8660254037844387076, 1.000000000000000000, 0.8660254037844387076, 1.000000000000000000, 0.8660254037844387076, 1.000000000000000000, 0.8660254037844387076, 1.000000000000000000, 0.8660254037844387076, 1.000000000000000000, 0.8660254037844387076, 1.000000000000000000, 0.8660254037844387076, 1.000000000000000000, 0.8660254037844387076, 1.000000000000000000, 0.8660254037844387076, 1.000000000000000000, 0.8660254037844387076, 1.000000000000000000, 0.8660254037844387076, 1.000000000000000000, 0.8660254037844387076, 1.000000000000000000, 0.8660254037844387076, 1.000000000000000000, 0.8660254037844387076, 1.000000000000000000, 0.8660254037844387076, 1.000000000000000000, 0.8660254037844387076, 1.000000000000000000, 0.8660254037844387076, 1.000000000000000000, 0.8660254037844387076, 1.000000000000000000, 0.8660254037844387076, 1.000000000000000000, 0.8660254037844387076, 1.000000000000000000, 0.8660254037844387076, 1.000000000000000000, 0.8660254037844387076, 1.000000000000000000, 0.8660254037844387076, 1.000000000000000000, 0.8660254037844387076, 1.000000000000000000, 0.8660254037844387076, 1.000000000000000000, 0.8660254037844387076, 1.000000000000000000, 0.8660254037844387076, 1.000000000000000000, 0.8660254037844387076, 1.000000000000000000, 0.8660254037844387076, 1.000000000000000000, 0.8660254037844387076, 1.000000000000000000, 0.8660254037844387076, 1.000000000000000000, 0.8660254037844387076, 1.000000000000000000, 0.8660254037844387076, 1.000000000000000000, 0.8660254037844387076, 1.000000000000000000, 0.8660254037844387076, 1.000000000000000000, 0.8660254037844387076, 1.000000000000000000, 0.8660254037844387076, 1.000000000000000000, 0.8660254037844387076, 1.000000000000000000, 0.8660254037844387076, 1.000000000000000000, 0.8660254037844387076, 1.000000000000000000, 0.8660254037844387076, 1.000000000000000000, 0.8660254037844387076, 1.000000000000000000, 0.8660254037844387076, 1.000000000000000000, 0.8660254037844387076, 1.000000000000000000, 0.8660254037844387076, 1.000000000000000000, 0.8660254037844387076, 1.000000000000000000) ) ) 
 REPRESENTATION_ITEM ( '' )  SURFACE ( )  );
#18018=VECTOR ( 'NONE', #12842, 1000.000000000000000 ) ;
#18029=CARTESIAN_POINT ( 'NONE',  ( 16.66113976570983368, 19.31733714366914256, 12.25316411605951927 ) ) ;
#18030=CARTESIAN_POINT ( 'NONE',  ( 20.74032577480890183, 20.74032577480882722, 13.61880215351699874 ) ) ;
#18035=CARTESIAN_POINT ( 'NONE',  ( -3.471149744654747238, 29.79887180468049479, 6.994934987683496530 ) ) ;
#18044=CARTESIAN_POINT ( 'NONE',  ( 15.67125403804690187, 21.32810828753921228, 11.30940107675849404 ) ) ;
#18046=AXIS2_PLACEMENT_3D ( 'NONE', #24119, #3726, #15900 ) ;
#18047=AXIS2_PLACEMENT_3D ( 'NONE', #20165, #6308, #18340 ) ;
#18056=( BOUNDED_CURVE ( )  B_SPLINE_CURVE ( 2, ( #19278, #24912, #852 ),
 .UNSPECIFIED., .F., .F. ) 
 B_SPLINE_CURVE_WITH_KNOTS ( ( 3, 3 ),
 ( 0.9889400238386636399, 1.000000000000000000 ),
 .UNSPECIFIED. ) 
 CURVE ( )  GEOMETRIC_REPRESENTATION_ITEM ( )  RATIONAL_B_SPLINE_CURVE ( ( 0.9401842259098239785, 0.9110946495778740051, 1.000000000000000000 ) ) 
 REPRESENTATION_ITEM ( '' )  );
#18060=CARTESIAN_POINT ( 'NONE',  ( 3.756430356250004099, 26.52812499938548285, 6.831223922626973533 ) ) ;
#18069=CARTESIAN_POINT ( 'NONE',  ( -2.620986760973688460E-15, -28.88124999877096855, 13.61880215351699874 ) ) ;
#18071=CARTESIAN_POINT ( 'NONE',  ( -1.878215178124995832, 28.55312499938548498, 5.746835883940462963 ) ) ;
#18078=DIRECTION ( 'NONE',  ( 0.000000000000000000, 0.000000000000000000, -1.000000000000000000 ) ) ;
#18087=VERTEX_POINT ( 'NONE', #5250 ) ;
#18089=CARTESIAN_POINT ( 'NONE',  ( 3.735045420075836212E-15, 25.81562499938548783, 4.662447845253954171 ) ) ;
#18092=CARTESIAN_POINT ( 'NONE',  ( 17.18919637734483885, 22.50159113326351346, 8.999999999999992895 ) ) ;
#18093=DIRECTION ( 'NONE',  ( 1.000000000000000000, -0.000000000000000000, 0.000000000000000000 ) ) ;
#18095=ADVANCED_FACE ( 'NONE', ( #3543 ), #3414, .F. ) ;
#18099=CARTESIAN_POINT ( 'NONE',  ( 4.000000000000001776, 27.66249999999999787, 11.30940107675849760 ) ) ;
#18104=CARTESIAN_POINT ( 'NONE',  ( 17.90514199329621903, 23.21753674921489008, 8.999999999999992895 ) ) ;
#18105=CARTESIAN_POINT ( 'NONE',  ( 0.000000000000000000, 0.000000000000000000, 0.000000000000000000 ) ) ;
#18109=( BOUNDED_CURVE ( )  B_SPLINE_CURVE ( 2, ( #11613, #23530, #5613, #25622, #1440, #25741, #9412, #1306, #19588 ),
 .UNSPECIFIED., .F., .F. ) 
 B_SPLINE_CURVE_WITH_KNOTS ( ( 3, 2, 2, 2, 3 ),
 ( 0.3250000000000000111, 0.3333333333333333148, 0.3499999999999999778, 0.3666666666666666408, 0.3750000000000000000 ),
 .UNSPECIFIED. ) 
 CURVE ( )  GEOMETRIC_REPRESENTATION_ITEM ( )  RATIONAL_B_SPLINE_CURVE ( ( 0.9330127018922194093, 0.9330127018922196314, 1.000000000000000000, 0.8660254037844387076, 1.000000000000000000, 0.8660254037844387076, 1.000000000000000000, 0.9330127018922194093, 0.9330127018922194093 ) ) 
 REPRESENTATION_ITEM ( '' )  );
#18113=CARTESIAN_POINT ( 'NONE',  ( 3.756430356250002323, 26.11562499938548498, 11.16877607737301226 ) ) ;
#18118=CIRCLE ( 'NONE', #16868, 4.000000000000000000 ) ;
#18119=DIRECTION ( 'NONE',  ( 0.000000000000000000, 0.000000000000000000, -1.000000000000000000 ) ) ;
#18121=FACE_OUTER_BOUND ( 'NONE', #24943, .T. ) ;
#18125=CARTESIAN_POINT ( 'NONE',  ( 4.000000000000003553, 29.48124999877097352, 6.690598923241489970 ) ) ;
#18129=CARTESIAN_POINT ( 'NONE',  ( 3.756430356250003655, 29.64062499938548356, 8.999999999999992895 ) ) ;
#18132=CARTESIAN_POINT ( 'NONE',  ( 17.26224429571663066, 22.91909854520893930, 11.30940107675849404 ) ) ;
#18135=CARTESIAN_POINT ( 'NONE',  ( -1.626862140677534194E-14, -28.43124999877096570, 12.99999999999999289 ) ) ;
#18136=CARTESIAN_POINT ( 'NONE',  ( 1.071796769724494336, 25.09240381056766367, 4.999999999999992895 ) ) ;
#18137=CARTESIAN_POINT ( 'NONE',  ( 1.878215178124995832, -25.74062499938548498, 5.746835883940462963 ) ) ;
#18141=CARTESIAN_POINT ( 'NONE',  ( -4.000000000000001776, -29.46250000000000568, 11.30940107675849760 ) ) ;
#18142=EDGE_CURVE ( 'NONE', #23031, #7614, #15071, .T. ) ;
#18144=ORIENTED_EDGE ( 'NONE', *, *, #9173, .F. ) ;
#18157=CARTESIAN_POINT ( 'NONE',  ( 22.09708691207964293, 16.44023266258718863, 8.999999999999992895 ) ) ;
#18160=CARTESIAN_POINT ( 'NONE',  ( 22.05731215476884088, 16.40045790527639369, 8.999999999999992895 ) ) ;
#18162=LINE ( 'NONE', #17889, #2576 ) ;
#18164=AXIS2_PLACEMENT_3D ( 'NONE', #1648, #3484, #11841 ) ;
#18166=CARTESIAN_POINT ( 'NONE',  ( -2.004590926901224535, 29.93374515888019971, 5.528701699505815803 ) ) ;
#18170=CARTESIAN_POINT ( 'NONE',  ( 4.000000000000003553, 27.19374999877096855, 8.999999999999992895 ) ) ;
#18172=CARTESIAN_POINT ( 'NONE',  ( 1.878215178124995832, -26.64062499938548711, 5.746835883940462963 ) ) ;
#18174=CARTESIAN_POINT ( 'NONE',  ( 17.64995053351269405, 19.16570006136466731, 4.999999999999992006 ) ) ;
#18184=CARTESIAN_POINT ( 'NONE',  ( -1.878215178124995832, 26.64062499938548711, 5.746835883940462963 ) ) ;
#18189=CARTESIAN_POINT ( 'NONE',  ( 3.999999999999997335, -25.65624999877097068, 11.30940107675849404 ) ) ;
#18191=CARTESIAN_POINT ( 'NONE',  ( -2.672651547586948120E-15, -25.59062499938548640, 13.33755215474602984 ) ) ;
#18195=DIRECTION ( 'NONE',  ( 0.000000000000000000, 0.000000000000000000, 1.000000000000000000 ) ) ;
#18196=ORIENTED_EDGE ( 'NONE', *, *, #12772, .T. ) ;
#18199=ORIENTED_EDGE ( 'NONE', *, *, #1096, .F. ) ;
#18200=ADVANCED_FACE ( 'NONE', ( #19756 ), #5891, .T. ) ;
#18201=EDGE_CURVE ( 'NONE', #5606, #17829, #25656, .T. ) ;
#18202=ORIENTED_EDGE ( 'NONE', *, *, #8703, .T. ) ;
#18210=CARTESIAN_POINT ( 'NONE',  ( 1.878215178125004048, 27.12812499938548783, 5.746835883940462963 ) ) ;
#18214=CARTESIAN_POINT ( 'NONE',  ( 15.94292067550354730, 21.25531543142222901, 11.16877607737301226 ) ) ;
#18219=CARTESIAN_POINT ( 'NONE',  ( -3.756430356249997438, 28.55312499938548498, 11.16877607737301048 ) ) ;
#18229=CARTESIAN_POINT ( 'NONE',  ( 21.39439954740644723, 15.73754529791400181, 11.30940107675849760 ) ) ;
#18231=CYLINDRICAL_SURFACE ( 'NONE', #14025, 4.000000000000000000 ) ;
#18237=AXIS2_PLACEMENT_3D ( 'NONE', #9489, #17472, #19544 ) ;
#18240=CARTESIAN_POINT ( 'NONE',  ( 3.579383266608310077, 29.78592973091716800, 10.80044967790457378 ) ) ;
#18241=CARTESIAN_POINT ( 'NONE',  ( 3.756430356250002323, 26.45312499938548356, 11.16877607737301226 ) ) ;
#18242=( BOUNDED_CURVE ( )  B_SPLINE_CURVE ( 2, ( #3287, #11259, #6151, #21, #17930, #23812, #1730, #21860, #282 ),
 .UNSPECIFIED., .F., .F. ) 
 B_SPLINE_CURVE_WITH_KNOTS ( ( 3, 2, 2, 2, 3 ),
 ( 0.8750000000000000000, 0.8833333333333333037, 0.9000000000000000222, 0.9166666666666666297, 0.9250000000000000444 ),
 .UNSPECIFIED. ) 
 CURVE ( )  GEOMETRIC_REPRESENTATION_ITEM ( )  RATIONAL_B_SPLINE_CURVE ( ( 0.9330127018922194093, 0.9330127018922194093, 1.000000000000000000, 0.8660254037844387076, 1.000000000000000000, 0.8660254037844387076, 1.000000000000000000, 0.9330127018922189652, 0.9330127018922194093 ) ) 
 REPRESENTATION_ITEM ( '' )  );
#18244=CARTESIAN_POINT ( 'NONE',  ( 21.90263254725334363, 19.07420542250708451, 12.46410161513774817 ) ) ;
#18246=CARTESIAN_POINT ( 'NONE',  ( -2.000000000000000888, -28.46874999877097068, 12.46410161513774817 ) ) ;
#18247=CARTESIAN_POINT ( 'NONE',  ( -1.626862140677534194E-14, -27.98124999877096997, 12.99999999999999289 ) ) ;
#18261=CARTESIAN_POINT ( 'NONE',  ( -3.735045420075836212E-15, -27.16562499938547859, 4.662447845253954171 ) ) ;
#18263=CARTESIAN_POINT ( 'NONE',  ( 3.834746474454188013E-15, 28.20624999877096428, 4.999999999999992006 ) ) ;
#18264=EDGE_CURVE ( 'NONE', #12515, #130, #13432, .T. ) ;
#18271=DIRECTION ( 'NONE',  ( -0.7071067811865487940, -0.7071067811865463515, 0.000000000000000000 ) ) ;
#18273=CARTESIAN_POINT ( 'NONE',  ( 17.87212389449003425, 23.52897814398233933, 8.999999999999992895 ) ) ;
#18274=CARTESIAN_POINT ( 'NONE',  ( 18.49305203628493288, 18.49305203628486183, 4.662447845253954171 ) ) ;
#18275=CARTESIAN_POINT ( 'NONE',  ( 20.26302869750799118, 20.26302869750790947, 4.381197846482986158 ) ) ;
#18276=EDGE_LOOP ( 'NONE', ( #5548, #24439, #11677, #24437 ) ) ;
#18277=CARTESIAN_POINT ( 'NONE',  ( 1.071796769724490117, -26.93259618943234202, 4.999999999999992895 ) ) ;
#18280=CARTESIAN_POINT ( 'NONE',  ( -2.440392720584789288, 29.90136469312441037, 12.17998752022640296 ) ) ;
#18282=CARTESIAN_POINT ( 'NONE',  ( 15.25349156384666216, 20.56588631976533676, 6.831223922626973533 ) ) ;
#18284=VERTEX_POINT ( 'NONE', #9693 ) ;
#18285=DIRECTION ( 'NONE',  ( 0.000000000000000000, -0.000000000000000000, -1.000000000000000000 ) ) ;
#18287=CARTESIAN_POINT ( 'NONE',  ( 3.756430356249997882, -26.30312499938548498, 11.16877607737301226 ) ) ;
#18288=CARTESIAN_POINT ( 'NONE',  ( 18.39361514561510091, 18.39361514561503341, 4.999999999999992006 ) ) ;
#18301=CARTESIAN_POINT ( 'NONE',  ( 3.756430356250003655, 29.75312499938548783, 8.999999999999992895 ) ) ;
#18302=EDGE_CURVE ( 'NONE', #8728, #19338, #23276, .T. ) ;
#18303=CARTESIAN_POINT ( 'NONE',  ( 3.469446951953614189E-15, 30.00000000000000355, 4.999999999999992006 ) ) ;
#18306=CARTESIAN_POINT ( 'NONE',  ( 21.21320343559646915, 21.21320343559638744, 12.99999999999999289 ) ) ;
#18308=CARTESIAN_POINT ( 'NONE',  ( 3.999999999999997335, -29.70624999877097139, 11.30940107675849404 ) ) ;
#18310=DIRECTION ( 'NONE',  ( -0.000000000000000000, -0.000000000000000000, 1.000000000000000000 ) ) ;
#18314=DIRECTION ( 'NONE',  ( -0.000000000000000000, -0.000000000000000000, 1.000000000000000000 ) ) ;
#18324=CARTESIAN_POINT ( 'NONE',  ( 19.82550637751787548, 19.82550637751778666, 12.99999999999999289 ) ) ;
#18326=CARTESIAN_POINT ( 'NONE',  ( 3.063240906311874401, 29.84319947910909931, 11.57226653943512851 ) ) ;
#18327=CARTESIAN_POINT ( 'NONE',  ( 3.756430356250003655, 27.50312499938548427, 8.999999999999992895 ) ) ;
#18332=CARTESIAN_POINT ( 'NONE',  ( 18.25213002337956780, 20.90832740133887313, 12.25316411605951927 ) ) ;
#18335=EDGE_CURVE ( 'NONE', #17313, #1348, #10917, .T. ) ;
#18336=CARTESIAN_POINT ( 'NONE',  ( -4.000000000000003553, -29.69687499938548569, 8.999999999999992895 ) ) ;
#18340=DIRECTION ( 'NONE',  ( 1.000000000000000000, 0.000000000000000000, 0.000000000000000000 ) ) ;
#18349=CIRCLE ( 'NONE', #7070, 24.00000000000000355 ) ;
#18353=VERTEX_POINT ( 'NONE', #12689 ) ;
#18354=AXIS2_PLACEMENT_3D ( 'NONE', #6433, #24215, #1991 ) ;
#18366=CARTESIAN_POINT ( 'NONE',  ( 1.878215178125000939, 28.66562499938548569, 12.25316411605952283 ) ) ;
#18372=CARTESIAN_POINT ( 'NONE',  ( 1.999999999999998224, -27.94374999877096855, 12.46410161513774639 ) ) ;
#18373=CARTESIAN_POINT ( 'NONE',  ( 1.878215178124998497, -25.44062499938548427, 12.25316411605951927 ) ) ;
#18378=CARTESIAN_POINT ( 'NONE',  ( 1.999999999999998224, -28.00000000000000000, 12.46410161513774639 ) ) ;
#18380=ORIENTED_EDGE ( 'NONE', *, *, #9920, .F. ) ;
#18384=CIRCLE ( 'NONE', #8359, 4.000000000000000000 ) ;
#18389=CARTESIAN_POINT ( 'NONE',  ( 3.756430356249997438, -26.41562499938548569, 11.16877607737301048 ) ) ;
#18391=CARTESIAN_POINT ( 'NONE',  ( -27.10000000000000497, 0.6000000000000000888, 19.00000000000000000 ) ) ;
#18394=CARTESIAN_POINT ( 'NONE',  ( 20.58122674904192451, 20.58122674904186411, 4.999999999999992006 ) ) ;
#18396=CARTESIAN_POINT ( 'NONE',  ( 3.959305671612554781E-15, 25.00000000000000000, 12.99999999999999289 ) ) ;
#18398=AXIS2_PLACEMENT_3D ( 'NONE', #3688, #5920, #18093 ) ;
#18401=CARTESIAN_POINT ( 'NONE',  ( 24.00000000000000355, 0.000000000000000000, 17.00000000000000000 ) ) ;
#18403=CARTESIAN_POINT ( 'NONE',  ( 19.76584424242071947, 19.76584424242064486, 4.662447845253954171 ) ) ;
#18404=CARTESIAN_POINT ( 'NONE',  ( 17.83234913717923220, 23.48920338667153729, 8.999999999999992895 ) ) ;
#18405=CARTESIAN_POINT ( 'NONE',  ( -3.999999999999996447, 28.37500000000000000, 8.999999999999992895 ) ) ;
#18409=CARTESIAN_POINT ( 'NONE',  ( -3.999903055931597784, 29.73215053696358368, 8.737301635141733414 ) ) ;
#18413=CARTESIAN_POINT ( 'NONE',  ( 3.999999999999997335, -27.96250000000000213, 11.30940107675849404 ) ) ;
#18415=DIRECTION ( 'NONE',  ( 1.000000000000000000, 0.000000000000000000, 0.000000000000000000 ) ) ;
#18417=CARTESIAN_POINT ( 'NONE',  ( -1.878215178125004048, -27.01562499938548711, 5.746835883940462963 ) ) ;
#18418=CARTESIAN_POINT ( 'NONE',  ( 18.55271417138208179, 18.55271417138200363, 12.99999999999999112 ) ) ;
#18421=DIRECTION ( 'NONE',  ( 0.000000000000000000, 0.000000000000000000, -1.000000000000000000 ) ) ;
#18423=CARTESIAN_POINT ( 'NONE',  ( 3.756430356249996994, -29.52812499938548640, 8.999999999999992895 ) ) ;
#18427=ORIENTED_EDGE ( 'NONE', *, *, #6840, .F. ) ;
#18432=CARTESIAN_POINT ( 'NONE',  ( -25.99307600111999150, -0.5999999999999996447, 19.59999999999999787 ) ) ;
#18435=DIRECTION ( 'NONE',  ( -0.7071067811865487940, -0.7071067811865463515, 0.000000000000000000 ) ) ;
#18436=CARTESIAN_POINT ( 'NONE',  ( 2.672651547586948120E-15, 29.64062499938548356, 13.33755215474602984 ) ) ;
#18443=CARTESIAN_POINT ( 'NONE',  ( -8.831537335106614961E-15, -26.23749999999999716, 12.99999999999999112 ) ) ;
#18444=CARTESIAN_POINT ( 'NONE',  ( 1.999999999999998224, -28.84374999877096712, 12.46410161513774639 ) ) ;
#18446=CARTESIAN_POINT ( 'NONE',  ( -1.878215178124995832, 29.45312499938548356, 5.746835883940462963 ) ) ;
#18447=VECTOR ( 'NONE', #10221, 1000.000000000000000 ) ;
#18450=CARTESIAN_POINT ( 'NONE',  ( 1.071796769724487230, -25.31740381056767220, 12.99999999999999467 ) ) ;
#18463=EDGE_LOOP ( 'NONE', ( #15718, #8257, #25008, #7025, #20700 ) ) ;
#18470=CARTESIAN_POINT ( 'NONE',  ( 1.878215178125004048, 26.22812499938548569, 5.746835883940462963 ) ) ;
#18475=CARTESIAN_POINT ( 'NONE',  ( 16.23460222274299980, 21.54699697866167440, 8.999999999999992895 ) ) ;
#18476=( BOUNDED_CURVE ( )  B_SPLINE_CURVE ( 2, ( #4274, #20611, #16447, #16054, #16172, #10391, #12639, #8319, #18263 ),
 .UNSPECIFIED., .F., .F. ) 
 B_SPLINE_CURVE_WITH_KNOTS ( ( 3, 2, 2, 2, 3 ),
 ( 0.5750000000000000666, 0.5833333333333333703, 0.5999999999999999778, 0.6166666666666666963, 0.6250000000000000000 ),
 .UNSPECIFIED. ) 
 CURVE ( )  GEOMETRIC_REPRESENTATION_ITEM ( )  RATIONAL_B_SPLINE_CURVE ( ( 0.9330127018922194093, 0.9330127018922198534, 1.000000000000000000, 0.8660254037844387076, 1.000000000000000000, 0.8660254037844387076, 1.000000000000000000, 0.9330127018922194093, 0.9330127018922194093 ) ) 
 REPRESENTATION_ITEM ( '' )  );
#18477=CARTESIAN_POINT ( 'NONE',  ( 20.30280345481879323, 20.30280345481869730, 4.999999999999992006 ) ) ;
#18483=CARTESIAN_POINT ( 'NONE',  ( 2.672651547586948120E-15, 28.17812499938548143, 13.33755215474603162 ) ) ;
#18486=DIRECTION ( 'NONE',  ( -0.7071067811865487940, -0.7071067811865463515, 0.000000000000000000 ) ) ;
#18488=ORIENTED_EDGE ( 'NONE', *, *, #12668, .T. ) ;
#18489=ORIENTED_EDGE ( 'NONE', *, *, #23797, .F. ) ;
#18510=CARTESIAN_POINT ( 'NONE',  ( -1.878215178124995832, 27.54062499938548214, 5.746835883940462963 ) ) ;
#18511=CARTESIAN_POINT ( 'NONE',  ( 15.35955758102464408, 20.67195233694332401, 8.999999999999992895 ) ) ;
#18513=CARTESIAN_POINT ( 'NONE',  ( 17.55392584295608316, 23.21078009244839180, 8.999999999999992895 ) ) ;
#18515=CARTESIAN_POINT ( 'NONE',  ( -1.071796769724488563, 29.31115380933863790, 12.99999999999999289 ) ) ;
#18516=CARTESIAN_POINT ( 'NONE',  ( -1.878215178125000939, -26.86562499938548498, 12.25316411605952283 ) ) ;
#18519=VERTEX_POINT ( 'NONE', #7426 ) ;
#18521=CARTESIAN_POINT ( 'NONE',  ( -4.000000000000001776, -29.01249999999999929, 11.30940107675849760 ) ) ;
#18523=ORIENTED_EDGE ( 'NONE', *, *, #1740, .F. ) ;
#18526=CARTESIAN_POINT ( 'NONE',  ( 3.999999999999995559, -29.18124999877096926, 6.690598923241487306 ) ) ;
#18529=ORIENTED_EDGE ( 'NONE', *, *, #12060, .F. ) ;
#18530=CARTESIAN_POINT ( 'NONE',  ( 1.878215178124998497, -26.00312499938548783, 12.25316411605951927 ) ) ;
#18538=AXIS2_PLACEMENT_3D ( 'NONE', #16086, #18567, #24951 ) ;
#18540=CARTESIAN_POINT ( 'NONE',  ( 1.999999999999995781, -28.30000000000000071, 5.535898384862237620 ) ) ;
#18541=CARTESIAN_POINT ( 'NONE',  ( 21.21320343559646915, 21.21320343559638744, 4.999999999999992006 ) ) ;
#18543=CARTESIAN_POINT ( 'NONE',  ( 4.000000000000003553, 25.48750000000000071, 6.690598923241489970 ) ) ;
#18544=CARTESIAN_POINT ( 'NONE',  ( 19.44764619088677549, 19.44764619088670088, 4.662447845253954171 ) ) ;
#18545=CARTESIAN_POINT ( 'NONE',  ( 18.66319960507342302, 21.49162672981954003, 12.46410161513774639 ) ) ;
#18549=DIRECTION ( 'NONE',  ( 0.000000000000000000, 0.000000000000000000, -1.000000000000000000 ) ) ;
#18553=CARTESIAN_POINT ( 'NONE',  ( 19.03001124868299243, 19.03001124868293559, 4.999999999999991118 ) ) ;
#18554=VERTEX_POINT ( 'NONE', #1156 ) ;
#18556=CARTESIAN_POINT ( 'NONE',  ( 2.000000000000003997, 26.81874999877096855, 5.535898384862238508 ) ) ;
#18557=CARTESIAN_POINT ( 'NONE',  ( -1.878215178125004048, -25.66562499938548569, 5.746835883940462963 ) ) ;
#18561=CARTESIAN_POINT ( 'NONE',  ( 1.878215178124998497, -26.79062499938548214, 12.25316411605951927 ) ) ;
#18567=DIRECTION ( 'NONE',  ( -0.000000000000000000, -0.000000000000000000, 1.000000000000000000 ) ) ;
#18568=EDGE_CURVE ( 'NONE', #25106, #7772, #17381, .T. ) ;
#18572=CARTESIAN_POINT ( 'NONE',  ( 1.878215178125000939, 29.67812499938548498, 12.25316411605952283 ) ) ;
#18573=CARTESIAN_POINT ( 'NONE',  ( 19.82550637751787548, 19.82550637751778666, 12.99999999999999289 ) ) ;
#18577=CARTESIAN_POINT ( 'NONE',  ( 3.756430356249997882, -26.86562499938548498, 11.16877607737301226 ) ) ;
#18581=CARTESIAN_POINT ( 'NONE',  ( 4.000096396247766251, -29.73212452601126188, 9.259737768674039415 ) ) ;
#18590=ORIENTED_EDGE ( 'NONE', *, *, #16159, .F. ) ;
#18593=CARTESIAN_POINT ( 'NONE',  ( 1.878215178125004048, 28.47812499938548569, 5.746835883940462963 ) ) ;
#18597=CARTESIAN_POINT ( 'NONE',  ( 21.70382253017380592, 19.04762515221435493, 5.746835883940462963 ) ) ;
#18599=CARTESIAN_POINT ( 'NONE',  ( 19.02117241391816904, 21.84959953866428606, 12.46410161513774639 ) ) ;
#18606=CARTESIAN_POINT ( 'NONE',  ( 4.000000000000003553, 29.50000000000000355, 8.999999999999992895 ) ) ;
#18624=CARTESIAN_POINT ( 'NONE',  ( 3.469446951953614189E-15, 30.00000000000000355, 8.999999999999992895 ) ) ;
#18625=CARTESIAN_POINT ( 'NONE',  ( 4.000000000000003553, 26.80000000000000071, 8.999999999999992895 ) ) ;
#18626=CARTESIAN_POINT ( 'NONE',  ( 15.98945208958084407, 21.64630633907315982, 11.30940107675849404 ) ) ;
#18628=( BOUNDED_CURVE ( )  B_SPLINE_CURVE ( 2, ( #7009, #22845, #744, #22723, #8713, #22588, #24671, #20879, #18925 ),
 .UNSPECIFIED., .F., .F. ) 
 B_SPLINE_CURVE_WITH_KNOTS ( ( 3, 2, 2, 2, 3 ),
 ( 0.6250000000000000000, 0.6333333333333333037, 0.6500000000000000222, 0.6666666666666666297, 0.6750000000000000444 ),
 .UNSPECIFIED. ) 
 CURVE ( )  GEOMETRIC_REPRESENTATION_ITEM ( )  RATIONAL_B_SPLINE_CURVE ( ( 0.9330127018922194093, 0.9330127018922194093, 1.000000000000000000, 0.8660254037844387076, 1.000000000000000000, 0.8660254037844387076, 1.000000000000000000, 0.9330127018922189652, 0.9330127018922194093 ) ) 
 REPRESENTATION_ITEM ( '' )  );
#18630=CARTESIAN_POINT ( 'NONE',  ( 3.756430356250003655, 27.84062499938548640, 8.999999999999992895 ) ) ;
#18631=EDGE_CURVE ( 'NONE', #5488, #20241, #24145, .T. ) ;
#18637=CARTESIAN_POINT ( 'NONE',  ( 1.878215178124995832, -27.54062499938548214, 5.746835883940462963 ) ) ;
#18641=CARTESIAN_POINT ( 'NONE',  ( 22.40202671059728345, 16.74517246110483271, 6.690598923241489970 ) ) ;
#18645=CARTESIAN_POINT ( 'NONE',  ( 3.469446951953614189E-15, 30.00000000000000355, 4.999999999999992006 ) ) ;
#18648=CARTESIAN_POINT ( 'NONE',  ( -3.735045420075836212E-15, -26.26562499938548356, 4.662447845253954171 ) ) ;
#18652=CARTESIAN_POINT ( 'NONE',  ( 23.33010436090463102, 17.67325011141217317, 8.999999999999992895 ) ) ;
#18655=LINE ( 'NONE', #10542, #12170 ) ;
#18656=CARTESIAN_POINT ( 'NONE',  ( 3.756430356250002323, 25.55312499938548498, 11.16877607737301403 ) ) ;
#18658=CARTESIAN_POINT ( 'NONE',  ( 18.57032807491351178, 21.22652545287281356, 12.25316411605951927 ) ) ;
#18659=CARTESIAN_POINT ( 'NONE',  ( 16.63462326141533865, 19.29082063937464397, 5.746835883940462963 ) ) ;
#18660=CARTESIAN_POINT ( 'NONE',  ( 20.50609665440990526, 14.84924240491746339, 8.999999999999992895 ) ) ;
#18666=CARTESIAN_POINT ( 'NONE',  ( 20.31164228958361306, 17.48321516483735394, 12.46410161513774817 ) ) ;
#18669=CARTESIAN_POINT ( 'NONE',  ( 3.752267015613588906E-15, 26.85624999877096641, 4.381197846482986158 ) ) ;
#18670=CARTESIAN_POINT ( 'NONE',  ( 1.878215178124998497, -27.69062499938548427, 12.25316411605951927 ) ) ;
#18672=ORIENTED_EDGE ( 'NONE', *, *, #19464, .T. ) ;
#18674=EDGE_CURVE ( 'NONE', #20151, #18519, #358, .T. ) ;
#18675=ORIENTED_EDGE ( 'NONE', *, *, #22775, .F. ) ;
#18676=CARTESIAN_POINT ( 'NONE',  ( 1.878215178124995832, -25.29062499938548569, 5.746835883940462963 ) ) ;
#18680=CARTESIAN_POINT ( 'NONE',  ( 21.21320343559646915, 21.21320343559638744, 8.999999999999992895 ) ) ;
#18681=CARTESIAN_POINT ( 'NONE',  ( 4.000000000000001776, 27.66249999999999787, 11.30940107675849760 ) ) ;
#18684=CARTESIAN_POINT ( 'NONE',  ( -1.878215178124995832, 28.89062499938548356, 5.746835883940462963 ) ) ;
#18691=CARTESIAN_POINT ( 'NONE',  ( -3.735045420075836212E-15, -25.81562499938548783, 4.662447845253954171 ) ) ;
#18692=( BOUNDED_CURVE ( )  B_SPLINE_CURVE ( 2, ( #8925, #16905, #24869, #21329, #15579 ),
 .UNSPECIFIED., .F., .F. ) 
 B_SPLINE_CURVE_WITH_KNOTS ( ( 3, 2, 3 ),
 ( 0.000000000000000000, 0.01666666666666666644, 0.02500000000000000486 ),
 .UNSPECIFIED. ) 
 CURVE ( )  GEOMETRIC_REPRESENTATION_ITEM ( )  RATIONAL_B_SPLINE_CURVE ( ( 1.000000000000000000, 0.8660254037844387076, 1.000000000000000000, 0.9330127018922194093, 0.9330127018922194093 ) ) 
 REPRESENTATION_ITEM ( '' )  );
#18696=CARTESIAN_POINT ( 'NONE',  ( -1.071796769724481901, 28.01740381056766438, 12.99999999999999645 ) ) ;
#18702=AXIS2_PLACEMENT_3D ( 'NONE', #1098, #6982, #14963 ) ;
#18703=EDGE_LOOP ( 'NONE', ( #16536, #19472, #8797 ) ) ;
#18706=DIRECTION ( 'NONE',  ( 0.000000000000000000, 0.000000000000000000, -1.000000000000000000 ) ) ;
#18709=CARTESIAN_POINT ( 'NONE',  ( -3.756430356249997438, 27.76562499938549067, 11.16877607737301048 ) ) ;
#18711=CARTESIAN_POINT ( 'NONE',  ( 19.34820930021694352, 19.34820930021687246, 4.999999999999992006 ) ) ;
#18712=CARTESIAN_POINT ( 'NONE',  ( 18.17030703624117294, 23.48270179215984754, 11.16877607737301226 ) ) ;
#18713=CARTESIAN_POINT ( 'NONE',  ( -1.878215178124995832, 26.30312499938548498, 5.746835883940462963 ) ) ;
#18719=CARTESIAN_POINT ( 'NONE',  ( 1.626862140677534194E-14, 27.98124999877096997, 12.99999999999999289 ) ) ;
#18720=DIRECTION ( 'NONE',  ( 1.000000000000000000, 0.000000000000000000, 0.000000000000000000 ) ) ;
#18726=DIRECTION ( 'NONE',  ( -0.7071067811865487940, -0.7071067811865463515, 0.000000000000000000 ) ) ;
#18727=VERTEX_POINT ( 'NONE', #15675 ) ;
#18728=ORIENTED_EDGE ( 'NONE', *, *, #2288, .T. ) ;
#18730=EDGE_CURVE ( 'NONE', #7828, #21834, #15795, .T. ) ;
#18736=ORIENTED_EDGE ( 'NONE', *, *, #1321, .F. ) ;
#18740=VECTOR ( 'NONE', #21907, 1000.000000000000000 ) ;
#18746=CIRCLE ( 'NONE', #9125, 0.5000000000000001110 ) ;
#18747=LINE ( 'NONE', #16805, #11749 ) ;
#18748=CARTESIAN_POINT ( 'NONE',  ( 16.95054783869437642, 22.26294259461305103, 8.999999999999992895 ) ) ;
#18749=CARTESIAN_POINT ( 'NONE',  ( 3.756430356250002323, 29.15312499938548640, 11.16877607737301226 ) ) ;
#18750=CARTESIAN_POINT ( 'NONE',  ( 18.25440349763447756, 18.25440349763440651, 4.662447845253954171 ) ) ;
#18754=CARTESIAN_POINT ( 'NONE',  ( -4.000000000000003553, -25.03750000000000142, 6.690598923241489970 ) ) ;
#18758=CARTESIAN_POINT ( 'NONE',  ( -3.756430356250003211, -28.32812499938548356, 6.831223922626973533 ) ) ;
#18762=CARTESIAN_POINT ( 'NONE',  ( -3.469446951953614189E-15, -30.00000000000000355, 8.999999999999992895 ) ) ;
#18766=( BOUNDED_CURVE ( )  B_SPLINE_CURVE ( 2, ( #3011, #784, #664, #24851, #14653, #4444, #8375, #18450, #10708 ),
 .UNSPECIFIED., .F., .F. ) 
 B_SPLINE_CURVE_WITH_KNOTS ( ( 3, 2, 2, 2, 3 ),
 ( 0.02500000000000000139, 0.03333333333333333287, 0.05000000000000000278, 0.06666666666666666574, 0.07500000000000001110 ),
 .UNSPECIFIED. ) 
 CURVE ( )  GEOMETRIC_REPRESENTATION_ITEM ( )  RATIONAL_B_SPLINE_CURVE ( ( 0.9330127018922194093, 0.9330127018922194093, 1.000000000000000000, 0.8660254037844387076, 1.000000000000000000, 0.8660254037844387076, 1.000000000000000000, 0.9330127018922191873, 0.9330127018922192983 ) ) 
 REPRESENTATION_ITEM ( '' )  );
#18767=CARTESIAN_POINT ( 'NONE',  ( 1.999999999999995781, -29.14374999877096784, 5.535898384862237620 ) ) ;
#18770=ADVANCED_FACE ( 'NONE', ( #10031 ), #16947, .F. ) ;
#18771=CARTESIAN_POINT ( 'NONE',  ( -1.878215178125004048, -27.12812499938548783, 5.746835883940462963 ) ) ;
#18773=( BOUNDED_CURVE ( )  B_SPLINE_CURVE ( 2, ( #23745, #5833, #13821, #3880, #19822, #12457, #1530, #9501, #1923 ),
 .UNSPECIFIED., .F., .F. ) 
 B_SPLINE_CURVE_WITH_KNOTS ( ( 3, 2, 2, 2, 3 ),
 ( 0.9250000000000000444, 0.9333333333333333481, 0.9499999999999999556, 0.9666666666666666741, 0.9749999999999999778 ),
 .UNSPECIFIED. ) 
 CURVE ( )  GEOMETRIC_REPRESENTATION_ITEM ( )  RATIONAL_B_SPLINE_CURVE ( ( 0.9330127018922194093, 0.9330127018922198534, 1.000000000000000000, 0.8660254037844387076, 1.000000000000000000, 0.8660254037844387076, 1.000000000000000000, 0.9330127018922194093, 0.9330127018922194093 ) ) 
 REPRESENTATION_ITEM ( '' )  );
#18781=VECTOR ( 'NONE', #11293, 1000.000000000000000 ) ;
#18786=CARTESIAN_POINT ( 'NONE',  ( 2.672651547586948120E-15, 25.47812499938548569, 13.33755215474603162 ) ) ;
#18789=CARTESIAN_POINT ( 'NONE',  ( 23.58876780933789519, 18.27637305341907492, 11.16877607737301226 ) ) ;
#18790=CARTESIAN_POINT ( 'NONE',  ( 17.05888733012726632, 19.71508470808657520, 12.25316411605951927 ) ) ;
#18791=FACE_OUTER_BOUND ( 'NONE', #3746, .T. ) ;
#18794=CIRCLE ( 'NONE', #15054, 4.000000000000000000 ) ;
#18795=DIRECTION ( 'NONE',  ( 0.000000000000000000, 1.000000000000000000, 0.000000000000000000 ) ) ;
#18796=LINE ( 'NONE', #20757, #4975 ) ;
#18800=CARTESIAN_POINT ( 'NONE',  ( 2.000000000000003997, 29.06874999877096855, 5.535898384862238508 ) ) ;
#18801=CARTESIAN_POINT ( 'NONE',  ( 1.878215178124995832, -28.89062499938548356, 5.746835883940462963 ) ) ;
#18802=CARTESIAN_POINT ( 'NONE',  ( -3.999999999999996447, 25.61874999877096926, 8.999999999999992895 ) ) ;
#18803=ORIENTED_EDGE ( 'NONE', *, *, #2666, .T. ) ;
#18808=CARTESIAN_POINT ( 'NONE',  ( 3.756430356249996994, -26.71562499938548285, 8.999999999999992895 ) ) ;
#18820=CARTESIAN_POINT ( 'NONE',  ( -1.878215178124998497, 28.14062499938548356, 12.25316411605951927 ) ) ;
#18822=CARTESIAN_POINT ( 'NONE',  ( 21.36466611845514052, 19.84891659060301805, 4.999999999999988454 ) ) ;
#18827=CARTESIAN_POINT ( 'NONE',  ( 22.01336592481439780, 20.38367064973063236, 12.84165680230635864 ) ) ;
#18829=CARTESIAN_POINT ( 'NONE',  ( 15.26024822061316577, 20.91710247010547619, 6.690598923241487306 ) ) ;
#18830=CARTESIAN_POINT ( 'NONE',  ( -3.756430356250002323, -27.91562499938548569, 11.16877607737301226 ) ) ;
#18832=DIRECTION ( 'NONE',  ( -0.000000000000000000, -0.000000000000000000, 1.000000000000000000 ) ) ;
#18833=AXIS2_PLACEMENT_3D ( 'NONE', #9639, #14077, #19943 ) ;
#18835=CARTESIAN_POINT ( 'NONE',  ( 23.02516456238698339, 17.36831031289453264, 11.30940107675849760 ) ) ;
#18843=ORIENTED_EDGE ( 'NONE', *, *, #8568, .F. ) ;
#18845=ORIENTED_EDGE ( 'NONE', *, *, #9124, .F. ) ;
#18851=CARTESIAN_POINT ( 'NONE',  ( 1.878215178125004048, 28.92812499938548854, 5.746835883940462963 ) ) ;
#18857=CARTESIAN_POINT ( 'NONE',  ( 17.50739442887878639, 22.81978918479745744, 8.999999999999992895 ) ) ;
#18859=CARTESIAN_POINT ( 'NONE',  ( 3.756430356250004099, 26.64062499938549067, 6.831223922626973533 ) ) ;
#18867=CARTESIAN_POINT ( 'NONE',  ( 3.469446951953614189E-15, 30.00000000000000355, 4.999999999999992006 ) ) ;
#18870=CARTESIAN_POINT ( 'NONE',  ( 23.69483382651587888, 18.38243907059705151, 8.999999999999992895 ) ) ;
#18877=CARTESIAN_POINT ( 'NONE',  ( 1.878215178124995832, -26.75312499938548783, 5.746835883940462963 ) ) ;
#18885=FACE_OUTER_BOUND ( 'NONE', #10777, .T. ) ;
#18888=CARTESIAN_POINT ( 'NONE',  ( 18.71181319714904490, 18.71181319714897384, 4.999999999999991118 ) ) ;
#18889=CARTESIAN_POINT ( 'NONE',  ( 19.52719570377026415, 19.52719570377018599, 4.662447845253954171 ) ) ;
#18893=CARTESIAN_POINT ( 'NONE',  ( 3.735045420075836212E-15, 27.95312499938548001, 4.662447845253954171 ) ) ;
#18896=CARTESIAN_POINT ( 'NONE',  ( 18.22561351908507277, 20.88181089704437454, 5.746835883940462963 ) ) ;
#18899=EDGE_CURVE ( 'NONE', #11588, #24788, #67, .T. ) ;
#18901=CARTESIAN_POINT ( 'NONE',  ( 3.756430356249996105, -27.57812499938548356, 6.831223922626973533 ) ) ;
#18904=CARTESIAN_POINT ( 'NONE',  ( 1.152368580279349075, 29.97923206407486774, 12.84165680230635509 ) ) ;
#18906=ORIENTED_EDGE ( 'NONE', *, *, #17987, .T. ) ;
#18912=CARTESIAN_POINT ( 'NONE',  ( 1.878215178124998497, -29.60312499938548569, 12.25316411605951927 ) ) ;
#18913=CARTESIAN_POINT ( 'NONE',  ( -3.469446951953614189E-15, -30.00000000000000355, 8.999999999999992895 ) ) ;
#18914=VECTOR ( 'NONE', #18314, 1000.000000000000000 ) ;
#18915=CARTESIAN_POINT ( 'NONE',  ( 19.50730832598392084, 19.50730832598383913, 12.99999999999999289 ) ) ;
#18920=EDGE_CURVE ( 'NONE', #16889, #14283, #17419, .T. ) ;
#18924=CARTESIAN_POINT ( 'NONE',  ( -3.756430356249997438, 26.30312499938548854, 11.16877607737301048 ) ) ;
#18925=CARTESIAN_POINT ( 'NONE',  ( -1.626862140677534194E-14, -28.43124999877096570, 12.99999999999999289 ) ) ;
#18926=CARTESIAN_POINT ( 'NONE',  ( 16.36952198446861217, 19.19794910921473630, 5.535898384862237620 ) ) ;
#18927=CARTESIAN_POINT ( 'NONE',  ( 18.89079960070236908, 18.89079960070229802, 4.662447845253954171 ) ) ;
#18932=CARTESIAN_POINT ( 'NONE',  ( 23.85222316637486273, 18.19536891688240843, 8.999999999999992895 ) ) ;
#18933=CARTESIAN_POINT ( 'NONE',  ( 19.60674521665374215, 19.60674521665367465, 13.33755215474603162 ) ) ;
#18937=CARTESIAN_POINT ( 'NONE',  ( -3.999999999999997335, 27.45624999877096784, 11.30940107675849404 ) ) ;
#18938=CARTESIAN_POINT ( 'NONE',  ( -1.878215178125000939, -29.11562499938548498, 12.25316411605952283 ) ) ;
#18944=CARTESIAN_POINT ( 'NONE',  ( -3.735045420075836212E-15, -27.05312499938548498, 4.662447845253954171 ) ) ;
#18952=CARTESIAN_POINT ( 'NONE',  ( 1.878215178125004048, 27.46562499938548640, 5.746835883940462963 ) ) ;
#18954=CARTESIAN_POINT ( 'NONE',  ( 3.999999999999995559, -28.78750000000000142, 6.690598923241487306 ) ) ;
#18957=LINE ( 'NONE', #5342, #10108 ) ;
#18960=CARTESIAN_POINT ( 'NONE',  ( -1.878215178125004048, -28.02812499938548640, 5.746835883940462963 ) ) ;
#18961=CARTESIAN_POINT ( 'NONE',  ( 17.16943652981684210, 22.82629077930915074, 6.690598923241487306 ) ) ;
#18962=EDGE_CURVE ( 'NONE', #8071, #19049, #18746, .T. ) ;
#18966=CARTESIAN_POINT ( 'NONE',  ( 2.642157743709451889, -29.88401080970086099, 12.01472878375391140 ) ) ;
#18967=VERTEX_POINT ( 'NONE', #4894 ) ;
#18968=LINE ( 'NONE', #10985, #3325 ) ;
#18970=ORIENTED_EDGE ( 'NONE', *, *, #2052, .F. ) ;
#18976=CYLINDRICAL_SURFACE ( 'NONE', #16809, 4.000000000000000000 ) ;
#18977=VERTEX_POINT ( 'NONE', #9809 ) ;
#18979=CARTESIAN_POINT ( 'NONE',  ( 3.756430356250002323, 28.81562499938548427, 11.16877607737301403 ) ) ;
#18981=CARTESIAN_POINT ( 'NONE',  ( 8.831537335106614961E-15, 27.13750000000000284, 12.99999999999999112 ) ) ;
#18982=CARTESIAN_POINT ( 'NONE',  ( 20.72043839702256207, 20.72043839702248036, 4.662447845253954171 ) ) ;
#18983=CARTESIAN_POINT ( 'NONE',  ( -3.756430356249997882, 26.86562499938548498, 11.16877607737301226 ) ) ;
#18984=DIRECTION ( 'NONE',  ( 0.000000000000000000, 1.000000000000000000, 0.000000000000000000 ) ) ;
#18990=CARTESIAN_POINT ( 'NONE',  ( 21.21320343559646915, 21.21320343559638744, 4.999999999999992006 ) ) ;
#18994=CARTESIAN_POINT ( 'NONE',  ( -2.000000000000003997, -25.52500000000000213, 5.535898384862238508 ) ) ;
#18999=ORIENTED_EDGE ( 'NONE', *, *, #1740, .T. ) ;
#19000=CARTESIAN_POINT ( 'NONE',  ( -3.756430356250002323, -26.56562499938548427, 11.16877607737301226 ) ) ;
#19002=DIRECTION ( 'NONE',  ( 1.000000000000000000, 0.000000000000000000, 0.000000000000000000 ) ) ;
#19009=CARTESIAN_POINT ( 'NONE',  ( 17.67766952966372429, 17.67766952966365679, 8.999999999999992895 ) ) ;
#19010=CARTESIAN_POINT ( 'NONE',  ( 19.44991966514168169, 16.79372228718224491, 12.25316411605952283 ) ) ;
#19012=CARTESIAN_POINT ( 'NONE',  ( 1.878215178125004048, 29.26562499938548356, 5.746835883940462963 ) ) ;
#19013=CARTESIAN_POINT ( 'NONE',  ( 17.24222938593383248, 22.55462414185250353, 6.831223922626973533 ) ) ;
#19017=CARTESIAN_POINT ( 'NONE',  ( -2.672651547586948120E-15, -27.27812499938548640, 13.33755215474603162 ) ) ;
#19022=CARTESIAN_POINT ( 'NONE',  ( 3.469446951953614189E-15, 30.00000000000000355, 4.999999999999992006 ) ) ;
#19026=CARTESIAN_POINT ( 'NONE',  ( 3.469446951953614189E-15, 30.00000000000000355, 8.999999999999992895 ) ) ;
#19029=CARTESIAN_POINT ( 'NONE',  ( 1.878215178124995832, -28.55312499938548498, 5.746835883940462963 ) ) ;
#19030=EDGE_CURVE ( 'NONE', #12924, #6983, #17683, .T. ) ;
#19034=CARTESIAN_POINT ( 'NONE',  ( 20.27939324173355473, 18.76364371388142516, 12.99999999999998757 ) ) ;
#19039=CARTESIAN_POINT ( 'NONE',  ( -27.10000000000000497, 0.6000000000000000888, 19.59999999999999787 ) ) ;
#19040=CARTESIAN_POINT ( 'NONE',  ( -1.878215178124998497, 26.34062499938548285, 12.25316411605951927 ) ) ;
#19042=CARTESIAN_POINT ( 'NONE',  ( 19.14491610062580662, 16.31648897587954750, 5.535898384862238508 ) ) ;
#19043=CARTESIAN_POINT ( 'NONE',  ( 18.17706369300767832, 23.83391794249997986, 11.30940107675849404 ) ) ;
#19044=FACE_OUTER_BOUND ( 'NONE', #3020, .T. ) ;
#19047=CARTESIAN_POINT ( 'NONE',  ( 17.50966790313369259, 20.16586528109299437, 5.746835883940462963 ) ) ;
#19049=VERTEX_POINT ( 'NONE', #17926 ) ;
#19051=CARTESIAN_POINT ( 'NONE',  ( -3.999999999999996447, 26.96874999877096712, 8.999999999999992895 ) ) ;
#19052=CARTESIAN_POINT ( 'NONE',  ( -3.756430356250002323, -28.70312499938548356, 11.16877607737301226 ) ) ;
#19058=CARTESIAN_POINT ( 'NONE',  ( -3.756430356250002323, -27.35312499938547859, 11.16877607737301226 ) ) ;
#19059=ORIENTED_EDGE ( 'NONE', *, *, #19094, .T. ) ;
#19061=EDGE_LOOP ( 'NONE', ( #10292, #12000, #1769, #2395, #5618, #13177 ) ) ;
#19062=EDGE_CURVE ( 'NONE', #21186, #7772, #22429, .T. ) ;
#19063=CARTESIAN_POINT ( 'NONE',  ( 19.92282844591920110, 22.43077534314094379, 12.59496732558994125 ) ) ;
#19069=CYLINDRICAL_SURFACE ( 'NONE', #17644, 4.000000000000000000 ) ;
#19070=CARTESIAN_POINT ( 'NONE',  ( -3.756430356249995661, 29.37812499938548427, 6.831223922626973533 ) ) ;
#19078=CARTESIAN_POINT ( 'NONE',  ( -1.878215178125004048, -27.57812499938548711, 5.746835883940462963 ) ) ;
#19081=CYLINDRICAL_SURFACE ( 'NONE', #15398, 4.000000000000000000 ) ;
#19088=ORIENTED_EDGE ( 'NONE', *, *, #3092, .T. ) ;
#19094=EDGE_CURVE ( 'NONE', #24890, #20539, #20836, .T. ) ;
#19095=CARTESIAN_POINT ( 'NONE',  ( 2.672651547586948120E-15, 27.84062499938548640, 13.33755215474603162 ) ) ;
#19099=CARTESIAN_POINT ( 'NONE',  ( 4.000000000000003553, 29.50000000000000355, 8.999999999999992895 ) ) ;
#19100=CARTESIAN_POINT ( 'NONE',  ( 3.756430356250003655, 27.05312499938548498, 8.999999999999992895 ) ) ;
#19101=CARTESIAN_POINT ( 'NONE',  ( 26.00000000000000355, 1.592040838891558898E-15, 20.00000599999999906 ) ) ;
#19107=DIRECTION ( 'NONE',  ( -0.7071067811865487940, -0.7071067811865463515, 0.000000000000000000 ) ) ;
#19110=CARTESIAN_POINT ( 'NONE',  ( -4.000000000000003553, -25.48750000000000071, 6.690598923241489970 ) ) ;
#19116=CARTESIAN_POINT ( 'NONE',  ( -1.878215178125000939, -26.52812499938548285, 12.25316411605952283 ) ) ;
#19117=ORIENTED_EDGE ( 'NONE', *, *, #12094, .F. ) ;
#19118=CARTESIAN_POINT ( 'NONE',  ( -1.999999999999998224, 28.90000000000000213, 12.46410161513774639 ) ) ;
#19121=CARTESIAN_POINT ( 'NONE',  ( 18.03564233677035489, 18.03564233677029094, 4.999999999999992006 ) ) ;
#19123=CARTESIAN_POINT ( 'NONE',  ( 18.41702535870033941, 19.93277488655231267, 12.99999999999999467 ) ) ;
#19128=CARTESIAN_POINT ( 'NONE',  ( 16.65886629145492748, 21.97126104737360919, 11.16877607737301226 ) ) ;
#19130=AXIS2_PLACEMENT_3D ( 'NONE', #24995, #7462, #9171 ) ;
#19131=CARTESIAN_POINT ( 'NONE',  ( -3.999999999999996003, 26.53750000000000142, 6.690598923241487306 ) ) ;
#19133=CARTESIAN_POINT ( 'NONE',  ( 21.12273290994980712, 15.81033815403099574, 11.16877607737301403 ) ) ;
#19146=CARTESIAN_POINT ( 'NONE',  ( -27.10000000000000497, 0.6000000000000000888, 19.59999999999999787 ) ) ;
#19151=CARTESIAN_POINT ( 'NONE',  ( 1.878215178124995832, -29.00312499938548427, 5.746835883940462963 ) ) ;
#19154=CARTESIAN_POINT ( 'NONE',  ( -4.000000000000003553, -26.29374999877096997, 8.999999999999992895 ) ) ;
#19159=VECTOR ( 'NONE', #13774, 1000.000000000000000 ) ;
#19163=CARTESIAN_POINT ( 'NONE',  ( 1.878215178125004048, 26.11562499938548498, 5.746835883940462963 ) ) ;
#19164=CARTESIAN_POINT ( 'NONE',  ( -3.974064950101062088, -29.73565934716929959, 8.475804415688518390 ) ) ;
#19165=CARTESIAN_POINT ( 'NONE',  ( 21.11597625318330174, 15.45912200369085632, 11.30940107675849760 ) ) ;
#19166=CARTESIAN_POINT ( 'NONE',  ( 15.35955758102464408, 20.67195233694332401, 8.999999999999992895 ) ) ;
#19170=CARTESIAN_POINT ( 'NONE',  ( 18.97034911358585418, 18.97034911358578668, 13.33755215474603162 ) ) ;
#19171=ORIENTED_EDGE ( 'NONE', *, *, #15059, .T. ) ;
#19172=CARTESIAN_POINT ( 'NONE',  ( 3.756430356250004099, 26.19062499938548783, 6.831223922626973533 ) ) ;
#19173=CARTESIAN_POINT ( 'NONE',  ( 3.756430356249996994, -29.41562499938548569, 8.999999999999992895 ) ) ;
#19179=CARTESIAN_POINT ( 'NONE',  ( -1.878215178125000939, -28.21562499938548640, 12.25316411605952283 ) ) ;
#19180=ORIENTED_EDGE ( 'NONE', *, *, #20774, .F. ) ;
#19187=ADVANCED_FACE ( 'NONE', ( #11906 ), #25770, .F. ) ;
#19190=CARTESIAN_POINT ( 'NONE',  ( -8.831537335106614961E-15, -27.13750000000000284, 12.99999999999999112 ) ) ;
#19193=CYLINDRICAL_SURFACE ( 'NONE', #10466, 4.000000000000000000 ) ;
#19196=CARTESIAN_POINT ( 'NONE',  ( 2.000000000000003997, 28.67500000000000426, 5.535898384862238508 ) ) ;
#19199=CARTESIAN_POINT ( 'NONE',  ( -0.5000000000000001110, 10.00000000000000000, 13.00000000000000178 ) ) ;
#19202=CARTESIAN_POINT ( 'NONE',  ( -1.878215178125004048, -28.92812499938548854, 5.746835883940462963 ) ) ;
#19203=CARTESIAN_POINT ( 'NONE',  ( 17.19595303411133713, 22.85280728360364577, 8.999999999999992895 ) ) ;
#19206=CARTESIAN_POINT ( 'NONE',  ( 2.007411586324088226, -29.93355017142139118, 12.46960170373642640 ) ) ;
#19210=DIRECTION ( 'NONE',  ( -0.7071067811865487940, -0.7071067811865463515, 0.000000000000000000 ) ) ;
#19216=ORIENTED_EDGE ( 'NONE', *, *, #7271, .F. ) ;
#19221=LINE ( 'NONE', #1180, #2643 ) ;
#19226=CARTESIAN_POINT ( 'NONE',  ( 1.878215178125004048, 25.32812499938548356, 5.746835883940462963 ) ) ;
#19228=CARTESIAN_POINT ( 'NONE',  ( 2.000000000000003997, 28.61874999877096926, 5.535898384862238508 ) ) ;
#19231=CARTESIAN_POINT ( 'NONE',  ( -2.000000000000000888, -25.76874999877096784, 12.46410161513774817 ) ) ;
#19235=CARTESIAN_POINT ( 'NONE',  ( -4.000000000000003553, -27.19374999877096855, 8.999999999999992895 ) ) ;
#19237=FACE_OUTER_BOUND ( 'NONE', #21482, .T. ) ;
#19242=ORIENTED_EDGE ( 'NONE', *, *, #17010, .T. ) ;
#19243=EDGE_CURVE ( 'NONE', #24788, #4092, #18766, .T. ) ;
#19245=EDGE_LOOP ( 'NONE', ( #22794, #14317, #12796, #3522 ) ) ;
#19250=VERTEX_POINT ( 'NONE', #10981 ) ;
#19251=CARTESIAN_POINT ( 'NONE',  ( -3.756430356250003655, -28.85312499938548569, 8.999999999999992895 ) ) ;
#19253=CARTESIAN_POINT ( 'NONE',  ( 3.756430356250003655, 25.14062499938548356, 8.999999999999992895 ) ) ;
#19257=DIRECTION ( 'NONE',  ( -0.000000000000000000, -0.000000000000000000, 1.000000000000000000 ) ) ;
#19260=DIRECTION ( 'NONE',  ( 0.000000000000000000, -1.000000000000000000, 0.000000000000000000 ) ) ;
#19262=CARTESIAN_POINT ( 'NONE',  ( 19.36809667800328683, 19.36809667800321932, 13.33755215474602984 ) ) ;
#19264=CARTESIAN_POINT ( 'NONE',  ( -3.999999999999996447, 25.22500000000000142, 8.999999999999992895 ) ) ;
#19265=CARTESIAN_POINT ( 'NONE',  ( 18.41350252340144422, 18.41350252340138383, 13.33755215474603162 ) ) ;
#19272=CARTESIAN_POINT ( 'NONE',  ( 1.878215178124995832, -28.89062499938548356, 5.746835883940462963 ) ) ;
#19278=CARTESIAN_POINT ( 'NONE',  ( 3.063240906311874401, 29.84319947910909931, 11.57226653943512851 ) ) ;
#19280=VERTEX_POINT ( 'NONE', #8515 ) ;
#19285=CARTESIAN_POINT ( 'NONE',  ( 3.756430356249996994, -28.62812499938548427, 8.999999999999992895 ) ) ;
#19286=DIRECTION ( 'NONE',  ( 1.000000000000000000, 0.000000000000000000, 0.000000000000000000 ) ) ;
#19294=SHAPE_DEFINITION_REPRESENTATION ( #1534, #16033 ) ;
#19295=LINE ( 'NONE', #23342, #25454 ) ;
#19298=CARTESIAN_POINT ( 'NONE',  ( -3.756430356249996994, 26.71562499938548285, 8.999999999999992895 ) ) ;
#19300=CARTESIAN_POINT ( 'NONE',  ( 22.68720666332504621, 17.37481190740622239, 6.831223922626973533 ) ) ;
#19301=CARTESIAN_POINT ( 'NONE',  ( 17.26874589022832751, 22.58114064614699856, 8.999999999999992895 ) ) ;
#19304=( BOUNDED_CURVE ( )  B_SPLINE_CURVE ( 2, ( #695, #8274, #16256, #8411, #20417, #24368, #14546, #10737, #4222 ),
 .UNSPECIFIED., .F., .F. ) 
 B_SPLINE_CURVE_WITH_KNOTS ( ( 3, 2, 2, 2, 3 ),
 ( 0.6750000000000000444, 0.6833333333333333481, 0.6999999999999999556, 0.7166666666666666741, 0.7249999999999999778 ),
 .UNSPECIFIED. ) 
 CURVE ( )  GEOMETRIC_REPRESENTATION_ITEM ( )  RATIONAL_B_SPLINE_CURVE ( ( 0.9330127018922194093, 0.9330127018922198534, 1.000000000000000000, 0.8660254037844387076, 1.000000000000000000, 0.8660254037844387076, 1.000000000000000000, 0.9330127018922194093, 0.9330127018922194093 ) ) 
 REPRESENTATION_ITEM ( '' )  );
#19309=CARTESIAN_POINT ( 'NONE',  ( 16.23460222274299980, 21.54699697866167440, 8.999999999999992895 ) ) ;
#19313=CARTESIAN_POINT ( 'NONE',  ( 3.735045420075836212E-15, 25.36562499938548498, 4.662447845253954171 ) ) ;
#19314=CARTESIAN_POINT ( 'NONE',  ( -2.000000000000003997, -25.07499999999999929, 5.535898384862238508 ) ) ;
#19321=CARTESIAN_POINT ( 'NONE',  ( -2.672651547586948120E-15, -27.27812499938548285, 13.33755215474602984 ) ) ;
#19333=CYLINDRICAL_SURFACE ( 'NONE', #23446, 4.000000000000000000 ) ;
#19338=VERTEX_POINT ( 'NONE', #10586 ) ;
#19339=DIRECTION ( 'NONE',  ( 1.000000000000000000, 0.000000000000000000, 0.000000000000000000 ) ) ;
#19348=ORIENTED_EDGE ( 'NONE', *, *, #15056, .F. ) ;
#19349=VECTOR ( 'NONE', #4097, 1000.000000000000000 ) ;
#19351=ORIENTED_EDGE ( 'NONE', *, *, #19062, .T. ) ;
#19356=CARTESIAN_POINT ( 'NONE',  ( 23.85222316637486273, 18.19536891688240843, 8.999999999999992895 ) ) ;
#19357=MECHANICAL_DESIGN_GEOMETRIC_PRESENTATION_REPRESENTATION('',(#12686),#22713);
#19360=SURFACE_STYLE_FILL_AREA ( #17791 ) ;
#19361=CARTESIAN_POINT ( 'NONE',  ( 3.756430356250002323, 28.81562499938548427, 11.16877607737301226 ) ) ;
#19369=CARTESIAN_POINT ( 'NONE',  ( -4.000000000000003553, -25.88124999877096499, 6.690598923241489970 ) ) ;
#19381=CARTESIAN_POINT ( 'NONE',  ( -3.735045420075836212E-15, -28.51562499938549067, 4.662447845253954171 ) ) ;
#19391=CARTESIAN_POINT ( 'NONE',  ( 18.17485398475098535, 18.17485398475091785, 4.662447845253954171 ) ) ;
#19395=CARTESIAN_POINT ( 'NONE',  ( 4.000000000000003553, 26.80000000000000071, 8.999999999999992895 ) ) ;
#19396=CIRCLE ( 'NONE', #18237, 8.000000000000000000 ) ;
#19397=CARTESIAN_POINT ( 'NONE',  ( 21.04090992281141581, 18.38471254485196837, 12.25316411605952283 ) ) ;
#19398=DIRECTION ( 'NONE',  ( 0.000000000000000000, -1.000000000000000000, 0.000000000000000000 ) ) ;
#19399=ADVANCED_FACE ( 'NONE', ( #17273 ), #7316, .T. ) ;
#19401=ORIENTED_EDGE ( 'NONE', *, *, #12668, .F. ) ;
#19403=CARTESIAN_POINT ( 'NONE',  ( -3.756430356250003655, -29.19062499938548072, 8.999999999999992895 ) ) ;
#19408=VERTEX_POINT ( 'NONE', #13330 ) ;
#19409=ORIENTED_EDGE ( 'NONE', *, *, #11449, .F. ) ;
#19410=DIRECTION ( 'NONE',  ( 0.000000000000000000, 0.000000000000000000, 1.000000000000000000 ) ) ;
#19412=CARTESIAN_POINT ( 'NONE',  ( -3.735045420075836212E-15, -28.06562499938548427, 4.662447845253954171 ) ) ;
#19422=CARTESIAN_POINT ( 'NONE',  ( -3.756430356249996994, 26.26562499938548711, 8.999999999999992895 ) ) ;
#19426=CARTESIAN_POINT ( 'NONE',  ( 18.71181319714904845, 18.71181319714898095, 4.381197846482986158 ) ) ;
#19427=CARTESIAN_POINT ( 'NONE',  ( 20.72271187127746828, 18.06651449331802439, 12.25316411605952283 ) ) ;
#19432=CARTESIAN_POINT ( 'NONE',  ( 16.26111872703749128, 21.57351348295617299, 11.16877607737301048 ) ) ;
#19435=CARTESIAN_POINT ( 'NONE',  ( 3.999999999999997335, -25.71250000000000213, 11.30940107675849404 ) ) ;
#19440=CARTESIAN_POINT ( 'NONE',  ( 3.756430356249996994, -28.96562499938548285, 8.999999999999992895 ) ) ;
#19443=CARTESIAN_POINT ( 'NONE',  ( 21.02609847369771501, 21.40030839749514868, 4.999999999999992895 ) ) ;
#19450=B_SPLINE_CURVE_WITH_KNOTS ( 'NONE', 3,
 ( #23665, #5240, #15310, #13220, #21189, #1708, #15575, #19356 ),
 .UNSPECIFIED., .F., .F.,
 ( 4, 2, 2, 4 ),
 ( 0.01599790909976502723, 0.01669365098321972177, 0.01738939286667441977, 0.01878087663358380885 ),
 .UNSPECIFIED. ) ;
#19452=CARTESIAN_POINT ( 'NONE',  ( 27.09999999999999787, 0.6000000000000000888, 19.59999999999999787 ) ) ;
#19453=( BOUNDED_CURVE ( )  B_SPLINE_CURVE ( 2, ( #4803, #20622, #16574, #24930, #16963, #1009, #12650, #13040, #21019 ),
 .UNSPECIFIED., .F., .F. ) 
 B_SPLINE_CURVE_WITH_KNOTS ( ( 3, 2, 2, 2, 3 ),
 ( 0.2750000000000000222, 0.2833333333333333259, 0.2999999999999999889, 0.3166666666666666519, 0.3250000000000000111 ),
 .UNSPECIFIED. ) 
 CURVE ( )  GEOMETRIC_REPRESENTATION_ITEM ( )  RATIONAL_B_SPLINE_CURVE ( ( 0.9330127018922194093, 0.9330127018922196314, 1.000000000000000000, 0.8660254037844387076, 1.000000000000000000, 0.8660254037844387076, 1.000000000000000000, 0.9330127018922191873, 0.9330127018922194093 ) ) 
 REPRESENTATION_ITEM ( '' )  );
#19457=CARTESIAN_POINT ( 'NONE',  ( -3.137519842735244810E-15, 26.85624999877096641, 4.999999999999991118 ) ) ;
#19460=CARTESIAN_POINT ( 'NONE',  ( -2.000000000000000888, -29.81874999877096855, 12.46410161513774817 ) ) ;
#19464=EDGE_CURVE ( 'NONE', #22072, #14822, #15117, .T. ) ;
#19465=CARTESIAN_POINT ( 'NONE',  ( 1.071796769724494558, 27.34240381056766722, 4.999999999999992895 ) ) ;
#19469=CARTESIAN_POINT ( 'NONE',  ( -1.071796769724495668, -26.25759618943233065, 12.99999999999999112 ) ) ;
#19470=ORIENTED_EDGE ( 'NONE', *, *, #21818, .F. ) ;
#19472=ORIENTED_EDGE ( 'NONE', *, *, #18335, .T. ) ;
#19475=DIRECTION ( 'NONE',  ( 0.000000000000000000, 0.000000000000000000, -1.000000000000000000 ) ) ;
#19480=CARTESIAN_POINT ( 'NONE',  ( -3.756430356249996994, 28.62812499938548427, 8.999999999999992895 ) ) ;
#19485=DIRECTION ( 'NONE',  ( 0.000000000000000000, 0.000000000000000000, -1.000000000000000000 ) ) ;
#19488=CARTESIAN_POINT ( 'NONE',  ( 1.999999999999998224, -26.59374999877096712, 12.46410161513774639 ) ) ;
#19489=CARTESIAN_POINT ( 'NONE',  ( 1.878215178125000939, 29.22812499938548569, 12.25316411605952283 ) ) ;
#19494=PLANE ( 'NONE',  #3730 ) ;
#19497=FACE_OUTER_BOUND ( 'NONE', #16400, .T. ) ;
#19499=CARTESIAN_POINT ( 'NONE',  ( -3.756430356250004099, -28.89062499938548356, 6.831223922626973533 ) ) ;
#19507=CARTESIAN_POINT ( 'NONE',  ( 23.40315227927642283, 18.09075752335759901, 6.831223922626973533 ) ) ;
#19508=DIRECTION ( 'NONE',  ( 0.000000000000000000, 0.000000000000000000, -1.000000000000000000 ) ) ;
#19509=EDGE_CURVE ( 'NONE', #19338, #11048, #25116, .T. ) ;
#19510=CARTESIAN_POINT ( 'NONE',  ( 4.000000000000001776, 28.11250000000000426, 11.30940107675849760 ) ) ;
#19513=CARTESIAN_POINT ( 'NONE',  ( -4.000000000000003553, -29.44374999877096855, 8.999999999999992895 ) ) ;
#19519=CARTESIAN_POINT ( 'NONE',  ( 1.071796769724491227, 26.44240381056766509, 4.999999999999989342 ) ) ;
#19534=CARTESIAN_POINT ( 'NONE',  ( 2.672651547586948120E-15, 27.72812499938548569, 13.33755215474602984 ) ) ;
#19539=CARTESIAN_POINT ( 'NONE',  ( 3.735045420075836212E-15, 28.85312499938548569, 4.662447845253954171 ) ) ;
#19541=CARTESIAN_POINT ( 'NONE',  ( 22.70696651085303941, 17.05011226136058866, 11.30940107675849760 ) ) ;
#19542=CARTESIAN_POINT ( 'NONE',  ( 18.33167953626305646, 20.98787691422236179, 12.25316411605951927 ) ) ;
#19544=DIRECTION ( 'NONE',  ( 1.000000000000000000, 0.000000000000000000, 0.000000000000000000 ) ) ;
#19549=AXIS2_PLACEMENT_3D ( 'NONE', #12024, #13882, #2242 ) ;
#19552=CARTESIAN_POINT ( 'NONE',  ( -4.000000000000001776, -27.21250000000000213, 11.30940107675849760 ) ) ;
#19555=ORIENTED_EDGE ( 'NONE', *, *, #9570, .T. ) ;
#19558=CARTESIAN_POINT ( 'NONE',  ( 3.469446951953614189E-15, 30.00000000000000355, 4.999999999999992006 ) ) ;
#19572=CARTESIAN_POINT ( 'NONE',  ( -1.071796769724494558, -27.34240381056766722, 4.999999999999992895 ) ) ;
#19577=CARTESIAN_POINT ( 'NONE',  ( 15.25349156384666216, 20.56588631976534387, 6.831223922626973533 ) ) ;
#19578=CARTESIAN_POINT ( 'NONE',  ( 21.76563060752939549, 16.10877635803694119, 6.690598923241489970 ) ) ;
#19581=CARTESIAN_POINT ( 'NONE',  ( 4.000000000000002665, 29.73213749463701205, 8.735714247490120599 ) ) ;
#19585=CARTESIAN_POINT ( 'NONE',  ( -4.000000000000003553, -25.39374999877096784, 8.999999999999992895 ) ) ;
#19587=ORIENTED_EDGE ( 'NONE', *, *, #12188, .F. ) ;
#19588=CARTESIAN_POINT ( 'NONE',  ( -1.859271017917182139E-15, -27.08124999877096784, 12.99999999999999289 ) ) ;
#19609=CARTESIAN_POINT ( 'NONE',  ( -3.756430356249995661, 29.04062499938548569, 6.831223922626973533 ) ) ;
#19610=VECTOR ( 'NONE', #8324, 999.9999999999998863 ) ;
#19612=CARTESIAN_POINT ( 'NONE',  ( 4.000000000000003553, 28.54374999877096997, 8.999999999999992895 ) ) ;
#19617=CARTESIAN_POINT ( 'NONE',  ( -2.000000000000000888, -27.56874999877096855, 12.46410161513774817 ) ) ;
#19618=CARTESIAN_POINT ( 'NONE',  ( -3.756430356249997882, 28.66562499938548569, 11.16877607737301226 ) ) ;
#19627=AXIS2_PLACEMENT_3D ( 'NONE', #10804, #4927, #24937 ) ;
#19628=VERTEX_POINT ( 'NONE', #19585 ) ;
#19630=VERTEX_POINT ( 'NONE', #11877 ) ;
#19631=CARTESIAN_POINT ( 'NONE',  ( -3.735045420075836212E-15, -27.61562499938548498, 4.662447845253954171 ) ) ;
#19635=ADVANCED_FACE ( 'NONE', ( #17769 ), #6248, .F. ) ;
#19639=EDGE_CURVE ( 'NONE', #8528, #16342, #22286, .T. ) ;
#19643=CARTESIAN_POINT ( 'NONE',  ( 16.55507374853184999, 19.21127112649115531, 5.746835883940462963 ) ) ;
#19648=CARTESIAN_POINT ( 'NONE',  ( 2.620986760973688460E-15, 28.03750000000000142, 13.61880215351699874 ) ) ;
#19651=CARTESIAN_POINT ( 'NONE',  ( 18.24985654912466515, 23.56225130504333620, 11.16877607737301048 ) ) ;
#19674=CARTESIAN_POINT ( 'NONE',  ( -1.071796769724491227, -26.89240381056766793, 4.999999999999989342 ) ) ;
#19684=CARTESIAN_POINT ( 'NONE',  ( 18.27871029367229383, 21.10713741841841085, 5.535898384862237620 ) ) ;
#19685=CARTESIAN_POINT ( 'NONE',  ( 23.37663577498192780, 18.06424101906310753, 8.999999999999992895 ) ) ;
#19686=CARTESIAN_POINT ( 'NONE',  ( -3.347751660414011177, -29.81285215011482137, 11.20140010723572388 ) ) ;
#19690=FACE_BOUND ( 'NONE', #23682, .T. ) ;
#19693=CARTESIAN_POINT ( 'NONE',  ( 18.55271417138208179, 18.55271417138200363, 12.99999999999999112 ) ) ;
#19695=CARTESIAN_POINT ( 'NONE',  ( 3.999999999999996003, -26.98750000000000426, 6.690598923241487306 ) ) ;
#19703=VERTEX_POINT ( 'NONE', #12785 ) ;
#19707=EDGE_CURVE ( 'NONE', #24890, #1173, #18796, .T. ) ;
#19712=EDGE_CURVE ( 'NONE', #7736, #2329, #21453, .T. ) ;
#19715=CARTESIAN_POINT ( 'NONE',  ( 3.469446951953614189E-15, 30.00000000000000355, 8.999999999999992895 ) ) ;
#19718=( BOUNDED_CURVE ( )  B_SPLINE_CURVE ( 2, ( #21928, #4008, #11974, #24135, #13573, #6097, #14080, #4129, #20084, #21539, #12108, #14733, #12492, #16445, #2815, #10654, #6743, #6485, #22185, #14591, #18530, #617, #10778, #20737, #24523, #12243, #4271, #18648, #2427, #12766, #8317, #18389, #10389, #8700, #12637, #14351, #20212, #20335, #14471, #2312, #731, #16305, #347, #16686, #10267, #6605, #24657, #22710, #4791, #22575, #18771, #18261, #862, #8842, #8583, #24273, #6360, #16829, #22313, #4391, #12371, #6220, #487, #16563, #8458, #24410, #14212, #22436, #4514, #2565, #20468, #10533, #20608, #4655, #2695, #19412, #1505, #9476, #23211, #11168, #23096, #13412, #17342, #15122, #11049, #25046, #15246, #5295, #19029, #3199, #19285, #23335, #15363, #3327, #1384, #22957, #9226, #24793, #2954, #13274, #19151, #1242, #10918, #7135, #3083, #12885, #17215, #4907, #7268, #21247, #16951, #1112, #6875, #14858, #5180, #9087, #18912, #11306, #22833, #25185, #9359 ),
 .UNSPECIFIED., .F., .F. ) 
 B_SPLINE_CURVE_WITH_KNOTS ( ( 3, 2, 2, 2, 2, 2, 2, 2, 2, 2, 2, 2, 2, 2, 2, 2, 2, 2, 2, 2, 2, 2, 2, 2, 2, 2, 2, 2, 2, 2, 2, 2, 2, 2, 2, 2, 2, 2, 2, 2, 2, 2, 2, 2, 2, 2, 2, 2, 2, 2, 2, 2, 2, 2, 2, 2, 2, 2, 2, 2, 3 ),
 ( 0.000000000000000000, 0.01666666666666666644, 0.03333333333333333287, 0.05000000000000000278, 0.06666666666666666574, 0.08333333333333332871, 0.1000000000000000056, 0.1166666666666666685, 0.1333333333333333315, 0.1499999999999999944, 0.1666666666666666574, 0.1833333333333333204, 0.2000000000000000111, 0.2166666666666666741, 0.2333333333333333370, 0.2500000000000000000, 0.2666666666666666630, 0.2833333333333333259, 0.2999999999999999889, 0.3166666666666666519, 0.3333333333333333148, 0.3499999999999999778, 0.3666666666666666408, 0.3833333333333333592, 0.4000000000000000222, 0.4166666666666666852, 0.4333333333333333481, 0.4500000000000000111, 0.4666666666666666741, 0.4833333333333333370, 0.5000000000000000000, 0.5166666666666667185, 0.5333333333333333259, 0.5500000000000000444, 0.5666666666666666519, 0.5833333333333333703, 0.5999999999999999778, 0.6166666666666666963, 0.6333333333333333037, 0.6500000000000000222, 0.6666666666666666297, 0.6833333333333333481, 0.6999999999999999556, 0.7166666666666666741, 0.7333333333333332815, 0.7500000000000000000, 0.7666666666666667185, 0.7833333333333333259, 0.8000000000000000444, 0.8166666666666666519, 0.8333333333333333703, 0.8499999999999999778, 0.8666666666666666963, 0.8833333333333333037, 0.9000000000000000222, 0.9166666666666666297, 0.9333333333333333481, 0.9499999999999999556, 0.9666666666666666741, 0.9833333333333332815, 1.000000000000000000 ),
 .UNSPECIFIED. ) 
 CURVE ( )  GEOMETRIC_REPRESENTATION_ITEM ( )  RATIONAL_B_SPLINE_CURVE ( ( 1.000000000000000000, 0.8660254037844387076, 1.000000000000000000, 0.8660254037844387076, 1.000000000000000000, 0.8660254037844387076, 1.000000000000000000, 0.8660254037844387076, 1.000000000000000000, 0.8660254037844387076, 1.000000000000000000, 0.8660254037844387076, 1.000000000000000000, 0.8660254037844387076, 1.000000000000000000, 0.8660254037844387076, 1.000000000000000000, 0.8660254037844387076, 1.000000000000000000, 0.8660254037844387076, 1.000000000000000000, 0.8660254037844387076, 1.000000000000000000, 0.8660254037844387076, 1.000000000000000000, 0.8660254037844387076, 1.000000000000000000, 0.8660254037844387076, 1.000000000000000000, 0.8660254037844387076, 1.000000000000000000, 0.8660254037844387076, 1.000000000000000000, 0.8660254037844387076, 1.000000000000000000, 0.8660254037844387076, 1.000000000000000000, 0.8660254037844387076, 1.000000000000000000, 0.8660254037844387076, 1.000000000000000000, 0.8660254037844387076, 1.000000000000000000, 0.8660254037844387076, 1.000000000000000000, 0.8660254037844387076, 1.000000000000000000, 0.8660254037844387076, 1.000000000000000000, 0.8660254037844387076, 1.000000000000000000, 0.8660254037844387076, 1.000000000000000000, 0.8660254037844387076, 1.000000000000000000, 0.8660254037844387076, 1.000000000000000000, 0.8660254037844387076, 1.000000000000000000, 0.8660254037844387076, 1.000000000000000000, 0.8660254037844387076, 1.000000000000000000, 0.8660254037844387076, 1.000000000000000000, 0.8660254037844387076, 1.000000000000000000, 0.8660254037844387076, 1.000000000000000000, 0.8660254037844387076, 1.000000000000000000, 0.8660254037844387076, 1.000000000000000000, 0.8660254037844387076, 1.000000000000000000, 0.8660254037844387076, 1.000000000000000000, 0.8660254037844387076, 1.000000000000000000, 0.8660254037844387076, 1.000000000000000000, 0.8660254037844387076, 1.000000000000000000, 0.8660254037844387076, 1.000000000000000000, 0.8660254037844387076, 1.000000000000000000, 0.8660254037844387076, 1.000000000000000000, 0.8660254037844387076, 1.000000000000000000, 0.8660254037844387076, 1.000000000000000000, 0.8660254037844387076, 1.000000000000000000, 0.8660254037844387076, 1.000000000000000000, 0.8660254037844387076, 1.000000000000000000, 0.8660254037844387076, 1.000000000000000000, 0.8660254037844387076, 1.000000000000000000, 0.8660254037844387076, 1.000000000000000000, 0.8660254037844387076, 1.000000000000000000, 0.8660254037844387076, 1.000000000000000000, 0.8660254037844387076, 1.000000000000000000, 0.8660254037844387076, 1.000000000000000000, 0.8660254037844387076, 1.000000000000000000, 0.8660254037844387076, 1.000000000000000000, 0.8660254037844387076, 1.000000000000000000, 0.8660254037844387076, 1.000000000000000000 ) ) 
 REPRESENTATION_ITEM ( '' )  );
#19719=CARTESIAN_POINT ( 'NONE',  ( -3.999999999999997335, 27.00624999877096855, 11.30940107675849404 ) ) ;
#19721=CARTESIAN_POINT ( 'NONE',  ( 19.42333939484895211, 16.59491227010269299, 5.535898384862238508 ) ) ;
#19722=ORIENTED_EDGE ( 'NONE', *, *, #14474, .F. ) ;
#19740=CYLINDRICAL_SURFACE ( 'NONE', #23927, 4.000000000000000000 ) ;
#19750=CARTESIAN_POINT ( 'NONE',  ( -1.878215178124995832, 28.10312499938548569, 5.746835883940462963 ) ) ;
#19756=FACE_OUTER_BOUND ( 'NONE', #20540, .T. ) ;
#19757=CARTESIAN_POINT ( 'NONE',  ( 20.43330379829292198, 15.12090904237410527, 8.999999999999992895 ) ) ;
#19758=CARTESIAN_POINT ( 'NONE',  ( -2.000000000000003997, -27.71874999877097068, 5.535898384862238508 ) ) ;
#19759=ADVANCED_FACE ( 'NONE', ( #19690, #212, #23492 ), #21789, .T. ) ;
#19760=CARTESIAN_POINT ( 'NONE',  ( 3.756430356250004099, 27.09062499938548285, 6.831223922626973533 ) ) ;
#19771=CARTESIAN_POINT ( 'NONE',  ( -1.878215178125000939, -28.77812499938548640, 12.25316411605952283 ) ) ;
#19774=( BOUNDED_CURVE ( )  B_SPLINE_CURVE ( 2, ( #15180, #1438, #6928, #18835, #23148, #5228, #4966, #13207, #13331 ),
 .UNSPECIFIED., .F., .F. ) 
 B_SPLINE_CURVE_WITH_KNOTS ( ( 3, 2, 2, 2, 3 ),
 ( 0.7750000000000000222, 0.7833333333333333259, 0.8000000000000000444, 0.8166666666666666519, 0.8249999999999999556 ),
 .UNSPECIFIED. ) 
 CURVE ( )  GEOMETRIC_REPRESENTATION_ITEM ( )  RATIONAL_B_SPLINE_CURVE ( ( 0.9330127018922194093, 0.9330127018922194093, 1.000000000000000000, 0.8660254037844387076, 1.000000000000000000, 0.8660254037844387076, 1.000000000000000000, 0.9330127018922198534, 0.9330127018922194093 ) ) 
 REPRESENTATION_ITEM ( '' )  );
#19780=CARTESIAN_POINT ( 'NONE',  ( 17.61346044605677008, 22.92585520197544469, 11.16877607737301226 ) ) ;
#19784=CARTESIAN_POINT ( 'NONE',  ( 2.000000000000003997, 29.12500000000000000, 5.535898384862238508 ) ) ;
#19793=CARTESIAN_POINT ( 'NONE',  ( -3.756430356249995661, 26.79062499938548925, 6.831223922626973533 ) ) ;
#19804=CARTESIAN_POINT ( 'NONE',  ( -1.878215178124998497, 26.34062499938548285, 12.25316411605951927 ) ) ;
#19809=CARTESIAN_POINT ( 'NONE',  ( 15.93641908099185933, 21.59327333048416975, 6.690598923241487306 ) ) ;
#19810=CARTESIAN_POINT ( 'NONE',  ( 20.48178985837210320, 20.48178985837202859, 4.662447845253954171 ) ) ;
#19811=CARTESIAN_POINT ( 'NONE',  ( -3.063240906311874401, -29.84319947910909931, 11.57226653943513028 ) ) ;
#19816=ORIENTED_EDGE ( 'NONE', *, *, #1933, .T. ) ;
#19818=CARTESIAN_POINT ( 'NONE',  ( 3.999999999999997335, -26.61250000000000071, 11.30940107675849404 ) ) ;
#19822=CARTESIAN_POINT ( 'NONE',  ( 3.999999999999996447, -29.66874999877096997, 8.999999999999992895 ) ) ;
#19823=EDGE_LOOP ( 'NONE', ( #13528, #24643, #16899, #24425 ) ) ;
#19825=ORIENTED_EDGE ( 'NONE', *, *, #21823, .F. ) ;
#19836=CARTESIAN_POINT ( 'NONE',  ( 19.33937046545212013, 22.16779759019823359, 12.46410161513774639 ) ) ;
#19837=CARTESIAN_POINT ( 'NONE',  ( 15.59820611967510295, 20.91060087559377934, 8.999999999999992895 ) ) ;
#19838=CARTESIAN_POINT ( 'NONE',  ( 15.28676472490765548, 20.94361897439997122, 8.999999999999992895 ) ) ;
#19845=CARTESIAN_POINT ( 'NONE',  ( -3.469446951953614189E-15, -30.00000000000000355, 8.999999999999992895 ) ) ;
#19847=ORIENTED_EDGE ( 'NONE', *, *, #12060, .T. ) ;
#19850=CARTESIAN_POINT ( 'NONE',  ( -4.000000000000001776, -26.31250000000000000, 11.30940107675849760 ) ) ;
#19851=ORIENTED_EDGE ( 'NONE', *, *, #25005, .F. ) ;
#19853=ORIENTED_EDGE ( 'NONE', *, *, #13998, .F. ) ;
#19856=ORIENTED_EDGE ( 'NONE', *, *, #8461, .F. ) ;
#19858=CARTESIAN_POINT ( 'NONE',  ( 18.87091222291601866, 18.87091222291595827, 12.99999999999999289 ) ) ;
#19864=CARTESIAN_POINT ( 'NONE',  ( 1.878215178125004048, 27.12812499938548783, 5.746835883940462963 ) ) ;
#19871=CARTESIAN_POINT ( 'NONE',  ( -2.620986760973688460E-15, -29.78124999877096712, 13.61880215351699874 ) ) ;
#19872=CARTESIAN_POINT ( 'NONE',  ( -3.756430356249996994, 28.17812499938548498, 8.999999999999992895 ) ) ;
#19874=CARTESIAN_POINT ( 'NONE',  ( -1.071796769724488563, 29.76115380933863364, 12.99999999999999289 ) ) ;
#19876=VERTEX_POINT ( 'NONE', #24259 ) ;
#19878=CARTESIAN_POINT ( 'NONE',  ( -1.878215178125000939, -29.11562499938548498, 12.25316411605952283 ) ) ;
#19883=CARTESIAN_POINT ( 'NONE',  ( -3.756430356250002323, -29.26562499938548356, 11.16877607737301226 ) ) ;
#19887=EDGE_CURVE ( 'NONE', #4092, #23536, #6594, .T. ) ;
#19890=CARTESIAN_POINT ( 'NONE',  ( 3.756430356250003655, 27.05312499938548498, 8.999999999999992895 ) ) ;
#19893=CARTESIAN_POINT ( 'NONE',  ( 20.79998790990604718, 20.79998790990596902, 4.662447845253954171 ) ) ;
#19897=CARTESIAN_POINT ( 'NONE',  ( -1.999999999999998224, 29.35000000000000142, 12.46410161513774639 ) ) ;
#19899=CARTESIAN_POINT ( 'NONE',  ( 19.60447174239884305, 22.26066912035814127, 12.25316411605951927 ) ) ;
#19900=CARTESIAN_POINT ( 'NONE',  ( 27.09999999999999787, 0.6000000000000000888, 19.00000000000000000 ) ) ;
#19904=( BOUNDED_CURVE ( )  B_SPLINE_CURVE ( 2, ( #17808, #12167, #7735, #25773, #7854 ),
 .UNSPECIFIED., .F., .F. ) 
 B_SPLINE_CURVE_WITH_KNOTS ( ( 3, 2, 3 ),
 ( 0.000000000000000000, 0.01666666666666666644, 0.02500000000000000486 ),
 .UNSPECIFIED. ) 
 CURVE ( )  GEOMETRIC_REPRESENTATION_ITEM ( )  RATIONAL_B_SPLINE_CURVE ( ( 1.000000000000000000, 0.8660254037844387076, 1.000000000000000000, 0.9330127018922194093, 0.9330127018922194093 ) ) 
 REPRESENTATION_ITEM ( '' )  );
#19905=ORIENTED_EDGE ( 'NONE', *, *, #16510, .F. ) ;
#19906=CARTESIAN_POINT ( 'NONE',  ( -3.469446951953614189E-15, -30.00000000000000355, 8.999999999999992895 ) ) ;
#19907=EDGE_CURVE ( 'NONE', #22503, #4122, #12478, .T. ) ;
#19908=CARTESIAN_POINT ( 'NONE',  ( -3.999999999999996003, 29.63124999877096499, 6.690598923241487306 ) ) ;
#19910=CARTESIAN_POINT ( 'NONE',  ( 17.75721904254721295, 17.75721904254714545, 4.999999999999992006 ) ) ;
#19919=CARTESIAN_POINT ( 'NONE',  ( 1.071796769724487675, 29.53615380933863221, 4.999999999999988454 ) ) ;
#19922=CARTESIAN_POINT ( 'NONE',  ( -3.756430356249996994, 26.71562499938548285, 8.999999999999992895 ) ) ;
#19924=DIRECTION ( 'NONE',  ( 0.000000000000000000, 1.000000000000000000, 0.000000000000000000 ) ) ;
#19926=CARTESIAN_POINT ( 'NONE',  ( 17.20921128712764414, 22.86606553661995278, 6.690598923241487306 ) ) ;
#19928=CYLINDRICAL_SURFACE ( 'NONE', #13423, 4.000000000000000000 ) ;
#19929=CARTESIAN_POINT ( 'NONE',  ( 3.999999999999997335, -27.90624999877097068, 11.30940107675849404 ) ) ;
#19930=CARTESIAN_POINT ( 'NONE',  ( -3.735045420075836212E-15, -25.70312499938548001, 4.662447845253954171 ) ) ;
#19932=B_SPLINE_CURVE_WITH_KNOTS ( 'NONE', 3,
 ( #19811, #17734, #19686, #7913, #21643, #6204, #10000, #9754 ),
 .UNSPECIFIED., .F., .F.,
 ( 4, 2, 2, 4 ),
 ( 0.01599790909976502723, 0.01669365098321972177, 0.01738939286667441630, 0.01878087663358380885 ),
 .UNSPECIFIED. ) ;
#19934=ORIENTED_EDGE ( 'NONE', *, *, #22393, .F. ) ;
#19936=CARTESIAN_POINT ( 'NONE',  ( -4.000000000000003553, -27.70000000000000284, 8.999999999999992895 ) ) ;
#19943=DIRECTION ( 'NONE',  ( -1.000000000000000000, 0.000000000000000000, -0.000000000000000000 ) ) ;
#19945=ORIENTED_EDGE ( 'NONE', *, *, #20774, .T. ) ;
#19959=CARTESIAN_POINT ( 'NONE',  ( 19.37037015225818948, 16.71417277429875625, 12.25316411605952283 ) ) ;
#19960=CARTESIAN_POINT ( 'NONE',  ( 17.16943652981684210, 22.82629077930915074, 6.690598923241487306 ) ) ;
#19961=ORIENTED_EDGE ( 'NONE', *, *, #19712, .T. ) ;
#19965=CARTESIAN_POINT ( 'NONE',  ( -3.015186248472646824, 29.84868090056883716, 11.64163568064553544 ) ) ;
#19969=CARTESIAN_POINT ( 'NONE',  ( 2.000000000000003997, 27.26874999877097139, 5.535898384862238508 ) ) ;
#19970=CARTESIAN_POINT ( 'NONE',  ( -1.999999999999995781, 25.54374999877096997, 5.535898384862237620 ) ) ;
#19988=CARTESIAN_POINT ( 'NONE',  ( 1.878215178125000939, 25.96562499938548285, 12.25316411605952283 ) ) ;
#19990=VECTOR ( 'NONE', #16752, 1000.000000000000000 ) ;
#19998=CARTESIAN_POINT ( 'NONE',  ( 3.999999999999997335, -28.80624999877096926, 11.30940107675849404 ) ) ;
#19999=CARTESIAN_POINT ( 'NONE',  ( -3.756430356249996994, 27.72812499938548569, 8.999999999999992895 ) ) ;
#20004=CARTESIAN_POINT ( 'NONE',  ( 1.071796769724487230, -25.97634618820330132, 4.999999999999992006 ) ) ;
#20007=FACE_OUTER_BOUND ( 'NONE', #11687, .T. ) ;
#20009=ORIENTED_EDGE ( 'NONE', *, *, #14381, .T. ) ;
#20010=DIRECTION ( 'NONE',  ( 0.000000000000000000, -1.000000000000000000, 0.000000000000000000 ) ) ;
#20014=VERTEX_POINT ( 'NONE', #5416 ) ;
#20020=CARTESIAN_POINT ( 'NONE',  ( 3.756430356250003211, 25.29062499938548569, 6.831223922626973533 ) ) ;
#20024=CARTESIAN_POINT ( 'NONE',  ( 22.36900861179109867, 17.05661385587227841, 6.831223922626973533 ) ) ;
#20027=DIRECTION ( 'NONE',  ( 0.000000000000000000, -1.000000000000000000, 0.000000000000000000 ) ) ;
#20031=CARTESIAN_POINT ( 'NONE',  ( 4.000000000000003553, 27.70000000000000284, 8.999999999999992895 ) ) ;
#20032=CARTESIAN_POINT ( 'NONE',  ( -3.756430356249996105, 29.37812499938548427, 6.831223922626973533 ) ) ;
#20034=EDGE_CURVE ( 'NONE', #2494, #1926, #13760, .T. ) ;
#20036=CARTESIAN_POINT ( 'NONE',  ( 19.18020767368691182, 21.83640505164621004, 5.746835883940462963 ) ) ;
#20043=CARTESIAN_POINT ( 'NONE',  ( 1.878215178125000939, 26.07812499938548356, 12.25316411605952283 ) ) ;
#20051=CARTESIAN_POINT ( 'NONE',  ( 4.000000000000001776, 29.01249999999999929, 11.30940107675849760 ) ) ;
#20053=CIRCLE ( 'NONE', #14223, 8.000000000000000000 ) ;
#20058=CARTESIAN_POINT ( 'NONE',  ( -3.756430356249995661, 25.77812499938548640, 6.831223922626973533 ) ) ;
#20068=FACE_OUTER_BOUND ( 'NONE', #23053, .T. ) ;
#20070=CARTESIAN_POINT ( 'NONE',  ( -1.878215178125000939, -25.51562499938548356, 12.25316411605952283 ) ) ;
#20080=LINE ( 'NONE', #219, #8817 ) ;
#20084=CARTESIAN_POINT ( 'NONE',  ( 1.878215178124998497, -25.55312499938548854, 12.25316411605951927 ) ) ;
#20086=CARTESIAN_POINT ( 'NONE',  ( 22.08382865906333947, 16.42697440957088872, 6.690598923241489970 ) ) ;
#20094=EDGE_CURVE ( 'NONE', #2304, #12209, #24910, .T. ) ;
#20100=CARTESIAN_POINT ( 'NONE',  ( 17.19595303411133713, 22.85280728360364577, 8.999999999999992895 ) ) ;
#20111=CARTESIAN_POINT ( 'NONE',  ( 2.000000000000003997, 26.36874999877096926, 5.535898384862238508 ) ) ;
#20112=CARTESIAN_POINT ( 'NONE',  ( 1.878215178124995832, -25.29062499938548569, 5.746835883940462963 ) ) ;
#20117=ORIENTED_EDGE ( 'NONE', *, *, #24489, .F. ) ;
#20119=ORIENTED_EDGE ( 'NONE', *, *, #16370, .F. ) ;
#20128=CARTESIAN_POINT ( 'NONE',  ( -3.756430356249995661, 29.49062499938548498, 6.831223922626973533 ) ) ;
#20133=DIRECTION ( 'NONE',  ( 0.000000000000000000, 0.000000000000000000, -1.000000000000000000 ) ) ;
#20136=CARTESIAN_POINT ( 'NONE',  ( 3.756430356249996994, -25.47812499938548569, 8.999999999999992895 ) ) ;
#20141=CARTESIAN_POINT ( 'NONE',  ( 3.999999999999995559, -26.03124999877097068, 6.690598923241487306 ) ) ;
#20142=EDGE_CURVE ( 'NONE', #22705, #21476, #6230, .T. ) ;
#20147=( BOUNDED_CURVE ( )  B_SPLINE_CURVE ( 2, ( #23807, #1973, #15, #10197, #663, #10072, #24065, #20263, #8632 ),
 .UNSPECIFIED., .F., .F. ) 
 B_SPLINE_CURVE_WITH_KNOTS ( ( 3, 2, 2, 2, 3 ),
 ( 0.2250000000000000056, 0.2333333333333333370, 0.2500000000000000000, 0.2666666666666666630, 0.2750000000000000222 ),
 .UNSPECIFIED. ) 
 CURVE ( )  GEOMETRIC_REPRESENTATION_ITEM ( )  RATIONAL_B_SPLINE_CURVE ( ( 0.9330127018922194093, 0.9330127018922194093, 1.000000000000000000, 0.8660254037844387076, 1.000000000000000000, 0.8660254037844387076, 1.000000000000000000, 0.9330127018922191873, 0.9330127018922194093 ) ) 
 REPRESENTATION_ITEM ( '' )  );
#20149=VERTEX_POINT ( 'NONE', #5934 ) ;
#20151=VERTEX_POINT ( 'NONE', #3581 ) ;
#20152=ORIENTED_EDGE ( 'NONE', *, *, #3035, .T. ) ;
#20153=AXIS2_PLACEMENT_3D ( 'NONE', #9177, #11257, #1342 ) ;
#20156=CARTESIAN_POINT ( 'NONE',  ( 2.672651547586948120E-15, 26.49062499938548498, 13.33755215474603162 ) ) ;
#20160=CARTESIAN_POINT ( 'NONE',  ( 17.61573392031167273, 20.27193129827097806, 12.25316411605951927 ) ) ;
#20165=CARTESIAN_POINT ( 'NONE',  ( 0.000000000000000000, 0.000000000000000000, 17.00000000000000000 ) ) ;
#20166=CARTESIAN_POINT ( 'NONE',  ( -3.756430356249996994, 28.51562499938548356, 8.999999999999992895 ) ) ;
#20170=VERTEX_POINT ( 'NONE', #1619 ) ;
#20177=ADVANCED_FACE ( 'NONE', ( #5672 ), #21618, .F. ) ;
#20183=DIRECTION ( 'NONE',  ( 0.000000000000000000, 0.000000000000000000, -1.000000000000000000 ) ) ;
#20190=CARTESIAN_POINT ( 'NONE',  ( 1.878215178125000939, 25.51562499938548356, 12.25316411605952283 ) ) ;
#20194=CARTESIAN_POINT ( 'NONE',  ( 19.66640735175089105, 19.66640735175081289, 4.999999999999992006 ) ) ;
#20195=PLANE ( 'NONE',  #18046 ) ;
#20196=CARTESIAN_POINT ( 'NONE',  ( 3.369928719974892281E-15, 25.11250000000000426, 4.999999999999992006 ) ) ;
#20197=CARTESIAN_POINT ( 'NONE',  ( -3.756430356250003655, -26.04062499938548569, 8.999999999999992895 ) ) ;
#20212=CARTESIAN_POINT ( 'NONE',  ( -3.756430356250003655, -26.60312499938548569, 8.999999999999992895 ) ) ;
#20214=CARTESIAN_POINT ( 'NONE',  ( 19.14933551713917126, 19.14933551713910376, 12.99999999999999289 ) ) ;
#20218=CARTESIAN_POINT ( 'NONE',  ( 3.469446951953614189E-15, 30.00000000000000355, 8.999999999999992895 ) ) ;
#20224=CARTESIAN_POINT ( 'NONE',  ( 8.831537335106614961E-15, 26.63124999877096855, 12.99999999999999112 ) ) ;
#20226=CARTESIAN_POINT ( 'NONE',  ( 16.20808571844850121, 21.52048047436717937, 6.831223922626973533 ) ) ;
#20227=CARTESIAN_POINT ( 'NONE',  ( 22.69370825783673951, 17.03685400834428521, 8.999999999999992895 ) ) ;
#20229=CARTESIAN_POINT ( 'NONE',  ( 1.999999999999995781, -26.95000000000000284, 5.535898384862237620 ) ) ;
#20232=CARTESIAN_POINT ( 'NONE',  ( -3.974007292349814424, 29.73566758725665338, 9.525109153848150711 ) ) ;
#20234=CARTESIAN_POINT ( 'NONE',  ( 19.47643616943617317, 16.82023879147673284, 5.746835883940462963 ) ) ;
#20235=CARTESIAN_POINT ( 'NONE',  ( 1.071796769724487230, -27.83259618943233704, 4.999999999999992006 ) ) ;
#20237=CARTESIAN_POINT ( 'NONE',  ( -1.999999999999998224, 25.69374999877097210, 12.46410161513774639 ) ) ;
#20238=CARTESIAN_POINT ( 'NONE',  ( -2.672651547586948120E-15, -25.47812499938548569, 13.33755215474602984 ) ) ;
#20241=VERTEX_POINT ( 'NONE', #8030 ) ;
#20253=CARTESIAN_POINT ( 'NONE',  ( 3.735045420075836212E-15, 27.05312499938548498, 4.662447845253954171 ) ) ;
#20260=CARTESIAN_POINT ( 'NONE',  ( 16.68772003600256326, 19.51614716074868028, 5.535898384862237620 ) ) ;
#20261=CARTESIAN_POINT ( 'NONE',  ( 3.999999999999996003, -28.73124999877096641, 6.690598923241487306 ) ) ;
#20263=CARTESIAN_POINT ( 'NONE',  ( 1.071796769724485454, -26.21740381056766367, 12.99999999999999467 ) ) ;
#20265=CARTESIAN_POINT ( 'NONE',  ( 1.626862140677534194E-14, 28.03750000000000497, 12.99999999999999289 ) ) ;
#20278=AXIS2_PLACEMENT_3D ( 'NONE', #4484, #315, #14050 ) ;
#20279=CARTESIAN_POINT ( 'NONE',  ( 23.26836714124207361, 18.93629030671969460, 11.57226653943513028 ) ) ;
#20280=CARTESIAN_POINT ( 'NONE',  ( 1.878215178125000939, 25.62812499938548783, 12.25316411605952283 ) ) ;
#20284=CARTESIAN_POINT ( 'NONE',  ( 21.99777755166815751, 16.68538279574934435, 11.16877607737301226 ) ) ;
#20285=( BOUNDED_CURVE ( )  B_SPLINE_CURVE ( 2, ( #4221, #24225, #6312, #14307, #7566, #13704, #3244, #13325, #15417 ),
 .UNSPECIFIED., .F., .F. ) 
 B_SPLINE_CURVE_WITH_KNOTS ( ( 3, 2, 2, 2, 3 ),
 ( 0.5250000000000000222, 0.5333333333333333259, 0.5500000000000000444, 0.5666666666666666519, 0.5750000000000000666 ),
 .UNSPECIFIED. ) 
 CURVE ( )  GEOMETRIC_REPRESENTATION_ITEM ( )  RATIONAL_B_SPLINE_CURVE ( ( 0.9330127018922194093, 0.9330127018922194093, 1.000000000000000000, 0.8660254037844387076, 1.000000000000000000, 0.8660254037844387076, 1.000000000000000000, 0.9330127018922189652, 0.9330127018922194093 ) ) 
 REPRESENTATION_ITEM ( '' )  );
#20286=CARTESIAN_POINT ( 'NONE',  ( 18.91510639674018890, 21.74353352148630236, 5.535898384862237620 ) ) ;
#20287=LINE ( 'NONE', #18336, #14215 ) ;
#20291=CARTESIAN_POINT ( 'NONE',  ( 2.672651547586948120E-15, 29.52812499938548285, 13.33755215474603162 ) ) ;
#20297=ORIENTED_EDGE ( 'NONE', *, *, #13413, .T. ) ;
#20303=ORIENTED_EDGE ( 'NONE', *, *, #17433, .F. ) ;
#20311=CARTESIAN_POINT ( 'NONE',  ( 1.859271017917182139E-15, 29.33124999877096428, 12.99999999999999289 ) ) ;
#20314=CARTESIAN_POINT ( 'NONE',  ( 3.756430356250003655, 27.39062499938548356, 8.999999999999992895 ) ) ;
#20317=CARTESIAN_POINT ( 'NONE',  ( 21.69050051289738690, 18.86207338815112067, 5.535898384862238508 ) ) ;
#20319=CARTESIAN_POINT ( 'NONE',  ( -3.999999999999996447, 29.27500000000000213, 8.999999999999992895 ) ) ;
#20335=CARTESIAN_POINT ( 'NONE',  ( -3.756430356250003211, -26.64062499938548356, 6.831223922626973533 ) ) ;
#20337=CARTESIAN_POINT ( 'NONE',  ( 1.057460391440397258E-14, -29.10624999877096641, 4.999999999999992006 ) ) ;
#20344=CARTESIAN_POINT ( 'NONE',  ( 16.53304042674895058, 22.18989467624125922, 6.690598923241487306 ) ) ;
#20346=CARTESIAN_POINT ( 'NONE',  ( 22.36900861179109867, 17.05661385587227841, 6.831223922626973533 ) ) ;
#20347=CARTESIAN_POINT ( 'NONE',  ( 20.42212772327495784, 20.42212772327488324, 13.61880215351699874 ) ) ;
#20353=CARTESIAN_POINT ( 'NONE',  ( -3.013274039476890653, 29.84885987243285399, 6.356496494711869616 ) ) ;
#20355=CARTESIAN_POINT ( 'NONE',  ( 16.97933781724378122, 19.63553519520309010, 12.25316411605951927 ) ) ;
#20357=VERTEX_POINT ( 'NONE', #6571 ) ;
#20358=CYLINDRICAL_SURFACE ( 'NONE', #16772, 4.000000000000000000 ) ;
#20359=CARTESIAN_POINT ( 'NONE',  ( 4.000000000000003553, 25.39374999877096784, 8.999999999999992895 ) ) ;
#20360=CARTESIAN_POINT ( 'NONE',  ( -1.878215178125004048, -26.56562499938548427, 5.746835883940462963 ) ) ;
#20361=CARTESIAN_POINT ( 'NONE',  ( -1.999999999999995781, 25.15000000000000213, 5.535898384862237620 ) ) ;
#20364=CARTESIAN_POINT ( 'NONE',  ( -3.756430356250002323, -26.90312499938548640, 11.16877607737301226 ) ) ;
#20371=VECTOR ( 'NONE', #3736, 1000.000000000000227 ) ;
#20373=CARTESIAN_POINT ( 'NONE',  ( -1.878215178124998497, 25.89062499938548356, 12.25316411605951927 ) ) ;
#20381=CARTESIAN_POINT ( 'NONE',  ( 1.999999999999995781, -28.69374999877096855, 5.535898384862237620 ) ) ;
#20382=CARTESIAN_POINT ( 'NONE',  ( 0.5000000000000001110, 10.00000000000000000, 13.00000000000000178 ) ) ;
#20387=CARTESIAN_POINT ( 'NONE',  ( 0.5247320085691752345, -29.99650235037416834, 5.025996973432255821 ) ) ;
#20394=ORIENTED_EDGE ( 'NONE', *, *, #12094, .T. ) ;
#20401=CARTESIAN_POINT ( 'NONE',  ( 1.878215178125000939, 26.07812499938548356, 12.25316411605952283 ) ) ;
#20402=AXIS2_PLACEMENT_3D ( 'NONE', #410, #2751, #20670 ) ;
#20406=CARTESIAN_POINT ( 'NONE',  ( 22.05081056025715114, 16.73841580433833442, 6.831223922626973533 ) ) ;
#20416=CARTESIAN_POINT ( 'NONE',  ( -8.831537335106614961E-15, -26.63124999877096855, 12.99999999999999112 ) ) ;
#20417=CARTESIAN_POINT ( 'NONE',  ( -4.000000000000003553, -28.15000000000000213, 8.999999999999992895 ) ) ;
#20421=EDGE_CURVE ( 'NONE', #22705, #11048, #4614, .T. ) ;
#20427=ORIENTED_EDGE ( 'NONE', *, *, #6643, .T. ) ;
#20428=DIRECTION ( 'NONE',  ( 0.000000000000000000, 0.000000000000000000, -1.000000000000000000 ) ) ;
#20433=ORIENTED_EDGE ( 'NONE', *, *, #14305, .T. ) ;
#20442=( BOUNDED_CURVE ( )  B_SPLINE_CURVE ( 2, ( #16749, #2625, #16496, #14654, #2747, #4323, #10709, #18696, #20265 ),
 .UNSPECIFIED., .F., .F. ) 
 B_SPLINE_CURVE_WITH_KNOTS ( ( 3, 2, 2, 2, 3 ),
 ( 0.6250000000000000000, 0.6333333333333333037, 0.6500000000000000222, 0.6666666666666666297, 0.6750000000000000444 ),
 .UNSPECIFIED. ) 
 CURVE ( )  GEOMETRIC_REPRESENTATION_ITEM ( )  RATIONAL_B_SPLINE_CURVE ( ( 0.9330127018922194093, 0.9330127018922194093, 1.000000000000000000, 0.8660254037844387076, 1.000000000000000000, 0.8660254037844387076, 1.000000000000000000, 0.9330127018922189652, 0.9330127018922194093 ) ) 
 REPRESENTATION_ITEM ( '' )  );
#20445=CARTESIAN_POINT ( 'NONE',  ( -3.756430356249995661, 27.57812499938548356, 6.831223922626973533 ) ) ;
#20448=CARTESIAN_POINT ( 'NONE',  ( 17.89864039878453283, 23.55549464827683437, 11.30940107675849404 ) ) ;
#20449=DIRECTION ( 'NONE',  ( 0.000000000000000000, -1.000000000000000000, 0.000000000000000000 ) ) ;
#20450=CARTESIAN_POINT ( 'NONE',  ( 1.878215178124998497, -28.59062499938548285, 12.25316411605951927 ) ) ;
#20456=CARTESIAN_POINT ( 'NONE',  ( -2.000000000000003997, -29.12500000000000000, 5.535898384862238508 ) ) ;
#20465=EDGE_CURVE ( 'NONE', #2390, #17829, #4875, .T. ) ;
#20468=CARTESIAN_POINT ( 'NONE',  ( -1.878215178125000939, -27.87812499938548427, 12.25316411605952283 ) ) ;
#20470=CARTESIAN_POINT ( 'NONE',  ( 19.30843454290614147, 19.30843454290607752, 4.999999999999991118 ) ) ;
#20477=CARTESIAN_POINT ( 'NONE',  ( 3.999999999999997335, -28.41250000000000142, 11.30940107675849404 ) ) ;
#20483=CARTESIAN_POINT ( 'NONE',  ( 21.41441445718925962, 16.10201970127043936, 6.831223922626973533 ) ) ;
#20485=CARTESIAN_POINT ( 'NONE',  ( 21.86285778994254514, 19.03443066519628601, 12.46410161513774817 ) ) ;
#20487=LINE ( 'NONE', #24536, #1771 ) ;
#20491=CARTESIAN_POINT ( 'NONE',  ( -3.470226642398214878, 29.79897209676519765, 11.00633161724385900 ) ) ;
#20493=CARTESIAN_POINT ( 'NONE',  ( 15.28000806814115720, 20.59240282405983535, 8.999999999999992895 ) ) ;
#20495=ORIENTED_EDGE ( 'NONE', *, *, #20465, .T. ) ;
#20498=CARTESIAN_POINT ( 'NONE',  ( 3.756430356249996994, -25.81562499938548427, 8.999999999999992895 ) ) ;
#20501=CARTESIAN_POINT ( 'NONE',  ( 17.92837382773583954, 19.44412335558781280, 4.999999999999992006 ) ) ;
#20505=CARTESIAN_POINT ( 'NONE',  ( -1.878215178125004048, -26.56562499938548427, 5.746835883940462963 ) ) ;
#20519=CARTESIAN_POINT ( 'NONE',  ( 2.672651547586948120E-15, 25.92812499938548498, 13.33755215474602984 ) ) ;
#20520=CARTESIAN_POINT ( 'NONE',  ( 23.36987911821542951, 17.71302486872297166, 8.999999999999992895 ) ) ;
#20527=CARTESIAN_POINT ( 'NONE',  ( 3.756430356249997882, -25.96562499938548640, 11.16877607737301226 ) ) ;
#20533=CARTESIAN_POINT ( 'NONE',  ( 3.871674220476135631, -29.74916513505594295, 7.961019890438434388 ) ) ;
#20534=ORIENTED_EDGE ( 'NONE', *, *, #925, .T. ) ;
#20535=FACE_OUTER_BOUND ( 'NONE', #9450, .T. ) ;
#20536=CARTESIAN_POINT ( 'NONE',  ( -3.469446951953614189E-15, -30.00000000000000355, 8.999999999999992895 ) ) ;
#20539=VERTEX_POINT ( 'NONE', #25144 ) ;
#20540=EDGE_LOOP ( 'NONE', ( #6638, #16859, #17449 ) ) ;
#20544=LINE ( 'NONE', #10465, #20985 ) ;
#20546=VERTEX_POINT ( 'NONE', #24886 ) ;
#20549=CARTESIAN_POINT ( 'NONE',  ( -3.756430356249997438, 28.21562499938548640, 11.16877607737301048 ) ) ;
#20554=CARTESIAN_POINT ( 'NONE',  ( 18.88852612644745932, 21.54472350440676109, 12.25316411605951927 ) ) ;
#20555=ADVANCED_FACE ( 'NONE', ( #15213 ), #5005, .F. ) ;
#20557=DIRECTION ( 'NONE',  ( -0.000000000000000000, -0.000000000000000000, 1.000000000000000000 ) ) ;
#20558=ADVANCED_FACE ( 'NONE', ( #23300, #12730 ), #13241, .T. ) ;
#20562=CARTESIAN_POINT ( 'NONE',  ( 3.469446951953614189E-15, 30.00000000000000355, 8.999999999999992895 ) ) ;
#20569=ORIENTED_EDGE ( 'NONE', *, *, #9173, .T. ) ;
#20574=ORIENTED_EDGE ( 'NONE', *, *, #15919, .T. ) ;
#20582=CARTESIAN_POINT ( 'NONE',  ( 16.30765014111479161, 21.96450439060710025, 11.30940107675849404 ) ) ;
#20585=CYLINDRICAL_SURFACE ( 'NONE', #21355, 4.000000000000000000 ) ;
#20586=CARTESIAN_POINT ( 'NONE',  ( 17.96814858504663448, 19.48389811289862195, 4.999999999999992895 ) ) ;
#20587=CARTESIAN_POINT ( 'NONE',  ( 15.38607408531914089, 20.69846884123782260, 11.16877607737301226 ) ) ;
#20589=CARTESIAN_POINT ( 'NONE',  ( -1.878215178124995832, 28.89062499938548356, 5.746835883940462963 ) ) ;
#20593=CARTESIAN_POINT ( 'NONE',  ( 23.34336261392093448, 17.68650836442847663, 11.30940107675849760 ) ) ;
#20596=CARTESIAN_POINT ( 'NONE',  ( -3.756430356250002323, -26.45312499938548356, 11.16877607737301403 ) ) ;
#20600=CARTESIAN_POINT ( 'NONE',  ( 21.01432965251868978, 18.18590252777242711, 5.535898384862238508 ) ) ;
#20608=CARTESIAN_POINT ( 'NONE',  ( -3.756430356250003655, -27.95312499938548711, 8.999999999999992895 ) ) ;
#20610=( BOUNDED_CURVE ( )  B_SPLINE_CURVE ( 2, ( #23111, #3213, #7152, #25064, #25441, #1127, #13556, #11322, #5193 ),
 .UNSPECIFIED., .F., .F. ) 
 B_SPLINE_CURVE_WITH_KNOTS ( ( 3, 2, 2, 2, 3 ),
 ( 0.7249999999999999778, 0.7333333333333332815, 0.7500000000000000000, 0.7666666666666667185, 0.7750000000000000222 ),
 .UNSPECIFIED. ) 
 CURVE ( )  GEOMETRIC_REPRESENTATION_ITEM ( )  RATIONAL_B_SPLINE_CURVE ( ( 0.9330127018922194093, 0.9330127018922194093, 1.000000000000000000, 0.8660254037844387076, 1.000000000000000000, 0.8660254037844387076, 1.000000000000000000, 0.9330127018922194093, 0.9330127018922194093 ) ) 
 REPRESENTATION_ITEM ( '' )  );
#20611=CARTESIAN_POINT ( 'NONE',  ( 1.071796769724498999, 28.00134618820329635, 12.99999999999998757 ) ) ;
#20616=ADVANCED_FACE ( 'NONE', ( #7476 ), #3432, .F. ) ;
#20622=CARTESIAN_POINT ( 'NONE',  ( 19.60322238135485762, 18.08747285350274581, 12.99999999999999112 ) ) ;
#20623=CARTESIAN_POINT ( 'NONE',  ( 18.46426205773553164, 21.12045943569482986, 5.746835883940462963 ) ) ;
#20624=CARTESIAN_POINT ( 'NONE',  ( 16.34066823992098350, 21.65306299583965455, 11.16877607737301226 ) ) ;
#20628=DIRECTION ( 'NONE',  ( 0.000000000000000000, -1.000000000000000000, 0.000000000000000000 ) ) ;
#20631=CARTESIAN_POINT ( 'NONE',  ( 20.75150184982686596, 15.43910709390805280, 8.999999999999992895 ) ) ;
#20635=CARTESIAN_POINT ( 'NONE',  ( 2.000000000000000888, 27.11874999877096926, 12.46410161513774817 ) ) ;
#20636=CARTESIAN_POINT ( 'NONE',  ( -3.756430356250004099, -26.97812499938548569, 6.831223922626973533 ) ) ;
#20637=CYLINDRICAL_SURFACE ( 'NONE', #20865, 4.000000000000000000 ) ;
#20638=ORIENTED_EDGE ( 'NONE', *, *, #7993, .F. ) ;
#20641=CARTESIAN_POINT ( 'NONE',  ( 1.878215178124998497, -29.60312499938548569, 12.25316411605951927 ) ) ;
#20651=CARTESIAN_POINT ( 'NONE',  ( -1.071796769724492338, -27.10134618820329777, 12.99999999999999467 ) ) ;
#20652=CARTESIAN_POINT ( 'NONE',  ( 3.756430356250002323, 29.15312499938548640, 11.16877607737301226 ) ) ;
#20653=ADVANCED_FACE ( 'NONE', ( #19497 ), #9445, .F. ) ;
#20655=CARTESIAN_POINT ( 'NONE',  ( 1.999999999999995781, -28.75000000000000000, 5.535898384862237620 ) ) ;
#20662=CARTESIAN_POINT ( 'NONE',  ( -3.756430356250003655, -26.60312499938548569, 8.999999999999992895 ) ) ;
#20670=DIRECTION ( 'NONE',  ( 0.000000000000000000, 0.000000000000000000, -1.000000000000000000 ) ) ;
#20672=ORIENTED_EDGE ( 'NONE', *, *, #22411, .F. ) ;
#20679=CARTESIAN_POINT ( 'NONE',  ( -3.756430356249996105, 28.59062499938548640, 6.831223922626973533 ) ) ;
#20682=CARTESIAN_POINT ( 'NONE',  ( 21.91595456452976975, 19.25975718657032232, 12.25316411605952283 ) ) ;
#20683=CARTESIAN_POINT ( 'NONE',  ( 0.000000000000000000, 0.000000000000000000, 15.00000000000000178 ) ) ;
#20689=CARTESIAN_POINT ( 'NONE',  ( -3.999999999999995559, 27.83124999877096784, 6.690598923241487306 ) ) ;
#20690=DIRECTION ( 'NONE',  ( 0.000000000000000000, 0.000000000000000000, 1.000000000000000000 ) ) ;
#20695=ORIENTED_EDGE ( 'NONE', *, *, #5845, .F. ) ;
#20697=ORIENTED_EDGE ( 'NONE', *, *, #9037, .F. ) ;
#20700=ORIENTED_EDGE ( 'NONE', *, *, #202, .T. ) ;
#20702=EDGE_LOOP ( 'NONE', ( #19470, #15952, #22892, #4007 ) ) ;
#20706=CARTESIAN_POINT ( 'NONE',  ( 23.96650046397252609, 18.30964621448006824, 8.999999999999992895 ) ) ;
#20713=CARTESIAN_POINT ( 'NONE',  ( 22.07732706455164617, 16.76493230863282591, 11.16877607737301226 ) ) ;
#20714=( BOUNDED_CURVE ( )  B_SPLINE_CURVE ( 2, ( #19910, #25685, #1768, #11823, #7766, #11553, #5937, #11434, #3975 ),
 .UNSPECIFIED., .F., .F. ) 
 B_SPLINE_CURVE_WITH_KNOTS ( ( 3, 2, 2, 2, 3 ),
 ( 0.02500000000000000486, 0.03333333333333333287, 0.05000000000000000278, 0.06666666666666666574, 0.07500000000000001110 ),
 .UNSPECIFIED. ) 
 CURVE ( )  GEOMETRIC_REPRESENTATION_ITEM ( )  RATIONAL_B_SPLINE_CURVE ( ( 0.9330127018922194093, 0.9330127018922194093, 1.000000000000000000, 0.8660254037844387076, 1.000000000000000000, 0.8660254037844387076, 1.000000000000000000, 0.9330127018922191873, 0.9330127018922192983 ) ) 
 REPRESENTATION_ITEM ( '' )  );
#20716=CARTESIAN_POINT ( 'NONE',  ( -1.878215178124998497, 29.04062499938548569, 12.25316411605951927 ) ) ;
#20717=CARTESIAN_POINT ( 'NONE',  ( 15.33304107673014904, 20.64543583264882898, 6.831223922626973533 ) ) ;
#20725=CARTESIAN_POINT ( 'NONE',  ( -3.756430356250002323, -27.80312499938548143, 11.16877607737301403 ) ) ;
#20729=DIRECTION ( 'NONE',  ( 0.000000000000000000, -1.000000000000000000, 0.000000000000000000 ) ) ;
#20732=VERTEX_POINT ( 'NONE', #7613 ) ;
#20737=CARTESIAN_POINT ( 'NONE',  ( -3.756430356250002323, -26.11562499938548498, 11.16877607737301403 ) ) ;
#20738=DIRECTION ( 'NONE',  ( 0.000000000000000000, 0.000000000000000000, -1.000000000000000000 ) ) ;
#20740=ADVANCED_FACE ( 'NONE', ( #8001 ), #13511, .F. ) ;
#20744=DIRECTION ( 'NONE',  ( 0.000000000000000000, 0.000000000000000000, -1.000000000000000000 ) ) ;
#20748=CARTESIAN_POINT ( 'NONE',  ( 19.30843454290614147, 19.30843454290607752, 4.999999999999991118 ) ) ;
#20750=CARTESIAN_POINT ( 'NONE',  ( 22.63417365473605614, 17.32177889881723587, 11.16877607737301226 ) ) ;
#20751=CARTESIAN_POINT ( 'NONE',  ( 15.65123912826409480, 20.96363388418277296, 6.831223922626973533 ) ) ;
#20757=CARTESIAN_POINT ( 'NONE',  ( 20.64530830152148155, 14.98845405202903613, 8.999999999999992895 ) ) ;
#20758=LINE ( 'NONE', #14754, #16300 ) ;
#20761=CARTESIAN_POINT ( 'NONE',  ( 2.000000000000003997, 27.71874999877097068, 5.535898384862238508 ) ) ;
#20762=CARTESIAN_POINT ( 'NONE',  ( 3.756430356249995661, -28.02812499938548640, 6.831223922626973533 ) ) ;
#20763=CARTESIAN_POINT ( 'NONE',  ( -1.071796769724487230, 25.71115380933864003, 12.99999999999999467 ) ) ;
#20769=CARTESIAN_POINT ( 'NONE',  ( -3.735045420075836212E-15, -29.41562499938548569, 4.662447845253954171 ) ) ;
#20774=EDGE_CURVE ( 'NONE', #1602, #17557, #9826, .T. ) ;
#20777=CARTESIAN_POINT ( 'NONE',  ( -4.000000000000003553, -27.23124999877096641, 6.690598923241489970 ) ) ;
#20778=CARTESIAN_POINT ( 'NONE',  ( 2.672651547586948120E-15, 27.27812499938548285, 13.33755215474602984 ) ) ;
#20779=CARTESIAN_POINT ( 'NONE',  ( 16.89101323559370016, 22.54786748508600525, 6.690598923241487306 ) ) ;
#20783=CARTESIAN_POINT ( 'NONE',  ( 21.61951122846571138, 20.80093850620003337, 12.96878440844335678 ) ) ;
#20785=CARTESIAN_POINT ( 'NONE',  ( 3.756430356249996994, -25.92812499938548498, 8.999999999999992895 ) ) ;
#20788=CARTESIAN_POINT ( 'NONE',  ( -4.000000000000003553, -28.63749999999999929, 6.690598923241489970 ) ) ;
#20795=ORIENTED_EDGE ( 'NONE', *, *, #14808, .F. ) ;
#20800=DIRECTION ( 'NONE',  ( 0.000000000000000000, -1.000000000000000000, 0.000000000000000000 ) ) ;
#20805=CARTESIAN_POINT ( 'NONE',  ( -3.756430356249997438, 29.56562499938549493, 11.16877607737301048 ) ) ;
#20807=CARTESIAN_POINT ( 'NONE',  ( 2.000000000000000888, 29.42500000000000071, 12.46410161513774817 ) ) ;
#20808=EDGE_CURVE ( 'NONE', #4579, #9527, #8765, .T. ) ;
#20809=CARTESIAN_POINT ( 'NONE',  ( 1.878215178125004048, 26.22812499938548569, 5.746835883940462963 ) ) ;
#20810=CARTESIAN_POINT ( 'NONE',  ( -15.85973458909327150, -20.67279826512042362, 20.00001200000000168 ) ) ;
#20813=DIRECTION ( 'NONE',  ( -0.7071067811865487940, -0.7071067811865463515, 0.000000000000000000 ) ) ;
#20814=FACE_OUTER_BOUND ( 'NONE', #13239, .T. ) ;
#20818=CARTESIAN_POINT ( 'NONE',  ( -27.10000000000000497, -0.5999999999999998668, 19.59999999999999787 ) ) ;
#20819=CARTESIAN_POINT ( 'NONE',  ( 21.21320343559646915, 21.21320343559638744, 8.999999999999992895 ) ) ;
#20822=ORIENTED_EDGE ( 'NONE', *, *, #11699, .T. ) ;
#20824=DIRECTION ( 'NONE',  ( 1.000000000000000000, 0.000000000000000000, -0.000000000000000000 ) ) ;
#20825=ORIENTED_EDGE ( 'NONE', *, *, #4892, .F. ) ;
#20826=CARTESIAN_POINT ( 'NONE',  ( 1.878215178124995832, -26.30312499938548498, 5.746835883940462963 ) ) ;
#20827=ORIENTED_EDGE ( 'NONE', *, *, #17605, .F. ) ;
#20828=CYLINDRICAL_SURFACE ( 'NONE', #3404, 4.000000000000000000 ) ;
#20832=ADVANCED_FACE ( 'NONE', ( #6034 ), #2601, .F. ) ;
#20836=CIRCLE ( 'NONE', #19549, 4.000000000000000000 ) ;
#20838=CARTESIAN_POINT ( 'NONE',  ( -3.999999999999997335, 28.35624999877096997, 11.30940107675849404 ) ) ;
#20839=CARTESIAN_POINT ( 'NONE',  ( 20.72271187127746828, 18.06651449331802439, 12.25316411605952283 ) ) ;
#20841=ADVANCED_FACE ( 'NONE', ( #6512 ), #16473, .T. ) ;
#20842=DIRECTION ( 'NONE',  ( 0.000000000000000000, 0.000000000000000000, -1.000000000000000000 ) ) ;
#20843=CARTESIAN_POINT ( 'NONE',  ( -1.878215178124998497, 27.69062499938548427, 12.25316411605951927 ) ) ;
#20844=CARTESIAN_POINT ( 'NONE',  ( 20.82877788845545552, 18.17258051049600454, 5.746835883940462963 ) ) ;
#20845=CARTESIAN_POINT ( 'NONE',  ( 4.000000000000003553, 26.78124999877097068, 6.690598923241489970 ) ) ;
#20847=ORIENTED_EDGE ( 'NONE', *, *, #24592, .F. ) ;
#20849=CARTESIAN_POINT ( 'NONE',  ( -3.999999999999995559, 29.23750000000000071, 6.690598923241487306 ) ) ;
#20850=CARTESIAN_POINT ( 'NONE',  ( -3.756430356250003655, -26.49062499938548498, 8.999999999999992895 ) ) ;
#20853=CARTESIAN_POINT ( 'NONE',  ( 3.959305739469038251E-15, 30.00000000000000355, 12.99999999999999289 ) ) ;
#20856=ORIENTED_EDGE ( 'NONE', *, *, #5845, .T. ) ;
#20861=CARTESIAN_POINT ( 'NONE',  ( 3.834746474454188013E-15, 25.56250000000000000, 4.999999999999992006 ) ) ;
#20862=CARTESIAN_POINT ( 'NONE',  ( 19.98460540328483859, 19.98460540328476398, 4.999999999999992006 ) ) ;
#20865=AXIS2_PLACEMENT_3D ( 'NONE', #10044, #8101, #24042 ) ;
#20870=EDGE_CURVE ( 'NONE', #10843, #8456, #517, .T. ) ;
#20877=CARTESIAN_POINT ( 'NONE',  ( 3.756430356250003211, 25.62812499938548072, 6.831223922626973533 ) ) ;
#20879=CARTESIAN_POINT ( 'NONE',  ( 1.071796769724481901, -28.41115380933862866, 12.99999999999999645 ) ) ;
#20880=CARTESIAN_POINT ( 'NONE',  ( 21.38562447863985483, 18.72942710068040739, 5.746835883940462963 ) ) ;
#20881=CARTESIAN_POINT ( 'NONE',  ( 21.75912901301770219, 16.44673425709888548, 11.16877607737301226 ) ) ;
#20887=CARTESIAN_POINT ( 'NONE',  ( 20.74922837557196331, 18.09303099761251588, 5.746835883940462963 ) ) ;
#20888=DIRECTION ( 'NONE',  ( -1.000000000000000000, -0.000000000000000000, -0.000000000000000000 ) ) ;
#20891=CARTESIAN_POINT ( 'NONE',  ( 4.000000000000003553, 27.64374999877096784, 8.999999999999992895 ) ) ;
#20892=CARTESIAN_POINT ( 'NONE',  ( 3.756430356249996994, -28.06562499938548427, 8.999999999999992895 ) ) ;
#20893=CARTESIAN_POINT ( 'NONE',  ( 3.369928719974892281E-15, 25.50624999877096855, 4.999999999999992006 ) ) ;
#20894=ORIENTED_EDGE ( 'NONE', *, *, #16662, .T. ) ;
#20895=CARTESIAN_POINT ( 'NONE',  ( -27.10000000000000497, -0.5999999999999998668, 19.59999999999999787 ) ) ;
#20898=CARTESIAN_POINT ( 'NONE',  ( -1.878215178125000939, -29.11562499938548498, 12.25316411605952283 ) ) ;
#20899=VERTEX_POINT ( 'NONE', #22860 ) ;
#20906=EDGE_CURVE ( 'NONE', #15602, #5488, #6777, .T. ) ;
#20911=CARTESIAN_POINT ( 'NONE',  ( 1.878215178125000939, 29.11562499938548498, 12.25316411605952283 ) ) ;
#20913=CARTESIAN_POINT ( 'NONE',  ( 23.39639562250992810, 17.73954137301747380, 6.690598923241489970 ) ) ;
#20920=CARTESIAN_POINT ( 'NONE',  ( 21.21320343559646915, 21.21320343559638744, 4.999999999999992006 ) ) ;
#20922=CARTESIAN_POINT ( 'NONE',  ( -3.756430356250004099, -27.09062499938548285, 6.831223922626973533 ) ) ;
#20923=( BOUNDED_CURVE ( )  B_SPLINE_CURVE ( 2, ( #25416, #5553, #9595, #13537, #17582, #15628, #22013, #2277, #6184 ),
 .UNSPECIFIED., .F., .F. ) 
 B_SPLINE_CURVE_WITH_KNOTS ( ( 3, 2, 2, 2, 3 ),
 ( 0.4250000000000000444, 0.4333333333333333481, 0.4500000000000000111, 0.4666666666666666741, 0.4750000000000000333 ),
 .UNSPECIFIED. ) 
 CURVE ( )  GEOMETRIC_REPRESENTATION_ITEM ( )  RATIONAL_B_SPLINE_CURVE ( ( 0.9330127018922194093, 0.9330127018922196314, 1.000000000000000000, 0.8660254037844387076, 1.000000000000000000, 0.8660254037844387076, 1.000000000000000000, 0.9330127018922191873, 0.9330127018922194093 ) ) 
 REPRESENTATION_ITEM ( '' )  );
#20931=CARTESIAN_POINT ( 'NONE',  ( 21.21320343559646915, 21.21320343559638744, 4.999999999999992006 ) ) ;
#20935=CIRCLE ( 'NONE', #6713, 26.00000000000000355 ) ;
#20937=ORIENTED_EDGE ( 'NONE', *, *, #11521, .T. ) ;
#20944=CARTESIAN_POINT ( 'NONE',  ( 3.756430356250002323, 29.26562499938548356, 11.16877607737301403 ) ) ;
#20949=CARTESIAN_POINT ( 'NONE',  ( 17.85210898470722896, 23.16450374062589646, 11.16877607737301226 ) ) ;
#20953=CARTESIAN_POINT ( 'NONE',  ( 20.67279826512042362, -15.85973458909328571, 20.00001200000000523 ) ) ;
#20963=VERTEX_POINT ( 'NONE', #3495 ) ;
#20968=DIRECTION ( 'NONE',  ( 0.000000000000000000, 1.000000000000000000, 0.000000000000000000 ) ) ;
#20970=CARTESIAN_POINT ( 'NONE',  ( -1.878215178125000939, -26.07812499938548356, 12.25316411605952283 ) ) ;
#20972=CARTESIAN_POINT ( 'NONE',  ( 0.000000000000000000, 10.00000000000000000, 13.00000000000000178 ) ) ;
#20974=VECTOR ( 'NONE', #9746, 1000.000000000000000 ) ;
#20976=CARTESIAN_POINT ( 'NONE',  ( 1.071796769724488563, -29.36740381056767291, 12.99999999999999289 ) ) ;
#20981=CARTESIAN_POINT ( 'NONE',  ( 15.96293558528635081, 21.61978983477866478, 8.999999999999992895 ) ) ;
#20982=CARTESIAN_POINT ( 'NONE',  ( 19.04989862646933929, 19.04989862646927534, 13.33755215474602984 ) ) ;
#20985=VECTOR ( 'NONE', #16507, 1000.000000000000000 ) ;
#20986=CARTESIAN_POINT ( 'NONE',  ( -3.999999999999997335, 26.16250000000000142, 11.30940107675849404 ) ) ;
#20989=CARTESIAN_POINT ( 'NONE',  ( 18.73170057493538820, 18.73170057493532425, 13.33755215474603162 ) ) ;
#20990=CYLINDRICAL_SURFACE ( 'NONE', #18702, 4.000000000000000000 ) ;
#20994=CARTESIAN_POINT ( 'NONE',  ( 3.756430356249996105, -27.12812499938548427, 6.831223922626973533 ) ) ;
#21006=CARTESIAN_POINT ( 'NONE',  ( -1.999999999999995781, 25.60000000000000142, 5.535898384862237620 ) ) ;
#21007=CARTESIAN_POINT ( 'NONE',  ( 2.000000000000000888, 25.82499999999999929, 12.46410161513774817 ) ) ;
#21012=AXIS2_PLACEMENT_3D ( 'NONE', #18624, #8677, #16803 ) ;
#21018=CARTESIAN_POINT ( 'NONE',  ( 1.878215178125004048, 25.66562499938548569, 5.746835883940462963 ) ) ;
#21019=CARTESIAN_POINT ( 'NONE',  ( 18.99023649137219039, 18.99023649137212999, 4.999999999999991118 ) ) ;
#21020=CARTESIAN_POINT ( 'NONE',  ( 21.70382253017380592, 19.04762515221435493, 5.746835883940462963 ) ) ;
#21021=CARTESIAN_POINT ( 'NONE',  ( 17.27101936448323016, 19.92721674244253549, 5.746835883940462963 ) ) ;
#21025=CARTESIAN_POINT ( 'NONE',  ( 22.66069015903055117, 17.34829540311172735, 8.999999999999992895 ) ) ;
#21029=CARTESIAN_POINT ( 'NONE',  ( 2.620986760973688460E-15, 28.43124999877096926, 13.61880215351699874 ) ) ;
#21030=CARTESIAN_POINT ( 'NONE',  ( -3.756430356250004099, -27.87812499938548427, 6.831223922626973533 ) ) ;
#21036=AXIS2_PLACEMENT_3D ( 'NONE', #13353, #15703, #13223 ) ;
#21038=CARTESIAN_POINT ( 'NONE',  ( -3.756430356250004099, -29.22812499938548925, 6.831223922626973533 ) ) ;
#21041=CARTESIAN_POINT ( 'NONE',  ( 21.21320343559646915, 21.21320343559638744, 4.999999999999992006 ) ) ;
#21042=EDGE_CURVE ( 'NONE', #8072, #6479, #24804, .T. ) ;
#21048=CARTESIAN_POINT ( 'NONE',  ( 2.672651547586948120E-15, 29.07812499938548001, 13.33755215474602984 ) ) ;
#21055=CARTESIAN_POINT ( 'NONE',  ( -2.672651547586948120E-15, -27.39062499938548356, 13.33755215474602984 ) ) ;
#21073=CARTESIAN_POINT ( 'NONE',  ( 2.672651547586948120E-15, 28.29062499938548925, 13.33755215474603162 ) ) ;
#21078=CARTESIAN_POINT ( 'NONE',  ( 3.756430356250002323, 27.01562499938548356, 11.16877607737301226 ) ) ;
#21079=CARTESIAN_POINT ( 'NONE',  ( -17.18149551509900519, -19.58805710660146104, 20.00001200000000523 ) ) ;
#21081=FACE_OUTER_BOUND ( 'NONE', #6240, .T. ) ;
#21084=FACE_OUTER_BOUND ( 'NONE', #23743, .T. ) ;
#21086=CARTESIAN_POINT ( 'NONE',  ( 23.82728881686095335, 18.17043456736849549, 8.999999999999992895 ) ) ;
#21090=ORIENTED_EDGE ( 'NONE', *, *, #20870, .T. ) ;
#21092=ORIENTED_EDGE ( 'NONE', *, *, #5496, .F. ) ;
#21093=CARTESIAN_POINT ( 'NONE',  ( -3.756430356250003655, -26.15312499938548640, 8.999999999999992895 ) ) ;
#21101=CARTESIAN_POINT ( 'NONE',  ( 3.469446951953614189E-15, 30.00000000000000355, 4.999999999999992006 ) ) ;
#21103=CARTESIAN_POINT ( 'NONE',  ( 20.08631576820957321, 17.43011839025013288, 12.25316411605952283 ) ) ;
#21105=CARTESIAN_POINT ( 'NONE',  ( 2.000000000000003997, 26.42500000000000071, 5.535898384862238508 ) ) ;
#21106=CARTESIAN_POINT ( 'NONE',  ( 22.13036007314063625, 16.81796531722181598, 6.831223922626973533 ) ) ;
#21111=CARTESIAN_POINT ( 'NONE',  ( 21.21320343559646915, 21.21320343559638744, 4.999999999999992006 ) ) ;
#21114=DIRECTION ( 'NONE',  ( 0.000000000000000000, 0.000000000000000000, -1.000000000000000000 ) ) ;
#21121=CARTESIAN_POINT ( 'NONE',  ( -1.999999999999998224, 25.75000000000000355, 12.46410161513774639 ) ) ;
#21133=( BOUNDED_CURVE ( )  B_SPLINE_CURVE ( 2, ( #22544, #2535, #4237, #20051, #8042, #319, #14182, #592, #2285 ),
 .UNSPECIFIED., .F., .F. ) 
 B_SPLINE_CURVE_WITH_KNOTS ( ( 3, 2, 2, 2, 3 ),
 ( 0.8750000000000000000, 0.8833333333333333037, 0.9000000000000000222, 0.9166666666666666297, 0.9250000000000000444 ),
 .UNSPECIFIED. ) 
 CURVE ( )  GEOMETRIC_REPRESENTATION_ITEM ( )  RATIONAL_B_SPLINE_CURVE ( ( 0.9330127018922194093, 0.9330127018922194093, 1.000000000000000000, 0.8660254037844387076, 1.000000000000000000, 0.8660254037844387076, 1.000000000000000000, 0.9330127018922189652, 0.9330127018922194093 ) ) 
 REPRESENTATION_ITEM ( '' )  );
#21136=CARTESIAN_POINT ( 'NONE',  ( -3.756430356249996994, 27.61562499938548143, 8.999999999999992895 ) ) ;
#21137=CARTESIAN_POINT ( 'NONE',  ( -3.594806220554922049, -29.78401552627944326, 7.226316032987424975 ) ) ;
#21138=CARTESIAN_POINT ( 'NONE',  ( 16.79378605318053985, 19.62221317792666753, 12.46410161513774639 ) ) ;
#21139=CARTESIAN_POINT ( 'NONE',  ( 20.53936981547090568, 15.22697505955208896, 6.831223922626973533 ) ) ;
#21140=CARTESIAN_POINT ( 'NONE',  ( 18.37725060138953737, 19.89300012924151417, 12.99999999999999289 ) ) ;
#21143=LINE ( 'NONE', #883, #11635 ) ;
#21144=CARTESIAN_POINT ( 'NONE',  ( 17.82786595466764012, 20.48406333262694190, 5.746835883940462963 ) ) ;
#21149=CARTESIAN_POINT ( 'NONE',  ( 4.000000000000003553, 27.19374999877096855, 8.999999999999992895 ) ) ;
#21150=CARTESIAN_POINT ( 'NONE',  ( -1.878215178125000939, -28.66562499938548569, 12.25316411605952283 ) ) ;
#21154=EDGE_LOOP ( 'NONE', ( #3453, #969, #5266, #16405 ) ) ;
#21155=CARTESIAN_POINT ( 'NONE',  ( 3.756430356249996994, -27.16562499938548214, 8.999999999999992895 ) ) ;
#21163=EDGE_CURVE ( 'NONE', #5788, #21186, #12633, .T. ) ;
#21169=LINE ( 'NONE', #15794, #10788 ) ;
#21173=CARTESIAN_POINT ( 'NONE',  ( -1.878215178125004048, -28.47812499938548569, 5.746835883940462963 ) ) ;
#21177=CARTESIAN_POINT ( 'NONE',  ( 0.2612076306139402004, -30.00000000000001066, 12.99999999999999467 ) ) ;
#21186=VERTEX_POINT ( 'NONE', #16948 ) ;
#21189=CARTESIAN_POINT ( 'NONE',  ( 23.65388548145850933, 18.45264921795818225, 10.59017455026297228 ) ) ;
#21194=CYLINDRICAL_SURFACE ( 'NONE', #8849, 4.000000000000000000 ) ;
#21195=ADVANCED_FACE ( 'NONE', ( #25042 ), #5422, .F. ) ;
#21197=CARTESIAN_POINT ( 'NONE',  ( 20.15576018847347584, 21.67150971632543133, 4.999999999999987566 ) ) ;
#21202=CARTESIAN_POINT ( 'NONE',  ( 3.999999999999996003, -26.48124999877096641, 6.690598923241487306 ) ) ;
#21212=VERTEX_POINT ( 'NONE', #3463 ) ;
#21213=CARTESIAN_POINT ( 'NONE',  ( -3.756430356250003655, -28.40312499938548640, 8.999999999999992895 ) ) ;
#21218=CYLINDRICAL_SURFACE ( 'NONE', #9330, 0.5000000000000001110 ) ;
#21221=CARTESIAN_POINT ( 'NONE',  ( 21.17576591853879719, 15.86337116261998048, 6.831223922626973533 ) ) ;
#21225=CARTESIAN_POINT ( 'NONE',  ( -3.999999999999996003, 26.08750000000000213, 6.690598923241487306 ) ) ;
#21227=CARTESIAN_POINT ( 'NONE',  ( 16.63234978716043244, 21.94474454307910705, 8.999999999999992895 ) ) ;
#21228=CARTESIAN_POINT ( 'NONE',  ( 1.071796769724491227, 26.83615380933863293, 4.999999999999989342 ) ) ;
#21229=ORIENTED_EDGE ( 'NONE', *, *, #5334, .T. ) ;
#21242=FACE_OUTER_BOUND ( 'NONE', #12486, .T. ) ;
#21247=CARTESIAN_POINT ( 'NONE',  ( -3.756430356250003211, -29.34062499938548640, 6.831223922626973533 ) ) ;
#21250=CARTESIAN_POINT ( 'NONE',  ( -4.000000000000001776, -26.25624999877096855, 11.30940107675849760 ) ) ;
#21261=CARTESIAN_POINT ( 'NONE',  ( -1.878215178124998497, 27.69062499938548427, 12.25316411605951927 ) ) ;
#21262=CARTESIAN_POINT ( 'NONE',  ( -0.2644264925860129734, -30.00000000000001421, 4.999999999999992006 ) ) ;
#21263=CARTESIAN_POINT ( 'NONE',  ( 20.87953742278953229, 20.87953742278945768, 13.33755215474602984 ) ) ;
#21264=CARTESIAN_POINT ( 'NONE',  ( 17.24222938593383248, 22.55462414185250353, 6.831223922626973533 ) ) ;
#21268=CARTESIAN_POINT ( 'NONE',  ( 18.14606400620158411, 20.80226138416088588, 5.746835883940462963 ) ) ;
#21272=CARTESIAN_POINT ( 'NONE',  ( 4.000000000000001776, 29.40624999877096357, 11.30940107675849760 ) ) ;
#21273=CARTESIAN_POINT ( 'NONE',  ( -2.672651547586948120E-15, -28.17812499938548143, 13.33755215474602984 ) ) ;
#21278=CARTESIAN_POINT ( 'NONE',  ( -15.85973458909327860, 20.67279826512041652, 20.00001200000000168 ) ) ;
#21279=CARTESIAN_POINT ( 'NONE',  ( -1.878215178125000939, -27.31562499938548427, 12.25316411605952283 ) ) ;
#21280=ORIENTED_EDGE ( 'NONE', *, *, #8826, .T. ) ;
#21292=CARTESIAN_POINT ( 'NONE',  ( -4.000000000000003553, -27.28749999999999787, 6.690598923241489970 ) ) ;
#21293=( BOUNDED_CURVE ( )  B_SPLINE_CURVE ( 2, ( #15372, #13422, #1119, #9095, #5187, #5305, #25433, #21396, #7518 ),
 .UNSPECIFIED., .F., .T. ) 
 B_SPLINE_CURVE_WITH_KNOTS ( ( 3, 2, 2, 2, 3 ),
 ( 0.4250000000000000444, 0.4333333333333333481, 0.4500000000000000111, 0.4666666666666666741, 0.4750000000000000333 ),
 .UNSPECIFIED. ) 
 CURVE ( )  GEOMETRIC_REPRESENTATION_ITEM ( )  RATIONAL_B_SPLINE_CURVE ( ( 0.9330127018922194093, 0.9330127018922196314, 1.000000000000000000, 0.8660254037844387076, 1.000000000000000000, 0.8660254037844387076, 1.000000000000000000, 0.9330127018922191873, 0.9330127018922194093 ) ) 
 REPRESENTATION_ITEM ( '' )  );
#21302=CARTESIAN_POINT ( 'NONE',  ( -3.735045420075836212E-15, -29.41562499938548569, 4.662447845253954171 ) ) ;
#21309=ORIENTED_EDGE ( 'NONE', *, *, #23210, .F. ) ;
#21319=ADVANCED_FACE ( 'NONE', ( #13269 ), #5038, .T. ) ;
#21329=CARTESIAN_POINT ( 'NONE',  ( -1.071796769724494336, -25.48615380933863150, 4.999999999999992895 ) ) ;
#21335=CARTESIAN_POINT ( 'NONE',  ( 1.057460391440397258E-14, -29.16249999999999787, 4.999999999999992006 ) ) ;
#21336=CARTESIAN_POINT ( 'NONE',  ( 3.999999999999997335, -26.10624999877096997, 11.30940107675849404 ) ) ;
#21341=CARTESIAN_POINT ( 'NONE',  ( 19.78573162020706988, 19.78573162020698462, 12.99999999999999289 ) ) ;
#21347=EDGE_LOOP ( 'NONE', ( #9193, #17521 ) ) ;
#21350=CARTESIAN_POINT ( 'NONE',  ( 3.756430356249997882, -27.31562499938548427, 11.16877607737301226 ) ) ;
#21351=ADVANCED_FACE ( 'NONE', ( #21242 ), #11299, .F. ) ;
#21354=EDGE_CURVE ( 'NONE', #10560, #2304, #7892, .T. ) ;
#21355=AXIS2_PLACEMENT_3D ( 'NONE', #8559, #6583, #8678 ) ;
#21360=VECTOR ( 'NONE', #22727, 1000.000000000000000 ) ;
#21364=CYLINDRICAL_SURFACE ( 'NONE', #23375, 4.000000000000000000 ) ;
#21365=CARTESIAN_POINT ( 'NONE',  ( 20.77801835412135745, 15.46562359820254784, 6.831223922626973533 ) ) ;
#21369=CARTESIAN_POINT ( 'NONE',  ( 4.000000000000003553, 25.48750000000000071, 6.690598923241489970 ) ) ;
#21370=CARTESIAN_POINT ( 'NONE',  ( 22.39552511608559371, 17.08313036016677700, 11.16877607737301403 ) ) ;
#21385=EDGE_CURVE ( 'NONE', #17898, #21186, #739, .T. ) ;
#21396=CARTESIAN_POINT ( 'NONE',  ( -1.071796769724485454, 27.11740381056766580, 12.99999999999999467 ) ) ;
#21399=CARTESIAN_POINT ( 'NONE',  ( -3.756430356249996105, 26.67812499938548498, 6.831223922626973533 ) ) ;
#21400=CARTESIAN_POINT ( 'NONE',  ( -0.5258040994055174222, -29.99650528990839859, 5.025965267902964939 ) ) ;
#21401=CARTESIAN_POINT ( 'NONE',  ( 20.56133937125558830, 20.56133937125551370, 13.33755215474602984 ) ) ;
#21402=CARTESIAN_POINT ( 'NONE',  ( 18.22561351908507277, 20.88181089704437454, 5.746835883940462963 ) ) ;
#21404=CARTESIAN_POINT ( 'NONE',  ( -3.756430356250003655, -29.64062499938548356, 8.999999999999992895 ) ) ;
#21405=CARTESIAN_POINT ( 'NONE',  ( 23.00150435104295354, 19.26045130116930082, 5.988343842124888461 ) ) ;
#21406=CARTESIAN_POINT ( 'NONE',  ( 19.28854716511979461, 19.28854716511973422, 13.33755215474603162 ) ) ;
#21409=CARTESIAN_POINT ( 'NONE',  ( 19.45547780925145531, 17.93972828139933995, 4.999999999999989342 ) ) ;
#21410=CARTESIAN_POINT ( 'NONE',  ( -3.756430356249996994, 26.37812499938548783, 8.999999999999992895 ) ) ;
#21411=CARTESIAN_POINT ( 'NONE',  ( -4.000000000000001776, -26.76249999999999929, 11.30940107675849760 ) ) ;
#21415=AXIS2_PLACEMENT_3D ( 'NONE', #22763, #14519, #2362 ) ;
#21416=CARTESIAN_POINT ( 'NONE',  ( 13.02991752792603108, 22.56362157461194329, 20.00001200000000168 ) ) ;
#21417=CARTESIAN_POINT ( 'NONE',  ( -2.672651547586948120E-15, -27.72812499938548569, 13.33755215474602984 ) ) ;
#21420=CARTESIAN_POINT ( 'NONE',  ( 18.61723445091742235, 23.52487603310535036, 11.00633161724385900 ) ) ;
#21430=CARTESIAN_POINT ( 'NONE',  ( 2.000000000000000888, 28.52500000000000213, 12.46410161513774817 ) ) ;
#21431=CARTESIAN_POINT ( 'NONE',  ( 1.859271017917182139E-15, 27.08124999877096784, 12.99999999999999289 ) ) ;
#21433=CARTESIAN_POINT ( 'NONE',  ( 20.05973549791684718, 17.23130837317058806, 5.535898384862238508 ) ) ;
#21436=CARTESIAN_POINT ( 'NONE',  ( -3.756430356250004099, -29.34062499938548640, 6.831223922626973533 ) ) ;
#21440=CARTESIAN_POINT ( 'NONE',  ( 4.000000000000001776, 27.21250000000000213, 11.30940107675849760 ) ) ;
#21453=( BOUNDED_CURVE ( )  B_SPLINE_CURVE ( 2, ( #6383, #14488, #8600, #370, #14373, #18282, #20493, #2591, #14877, #4681, #12660, #2836, #20631, #8341, #20234, #22332, #2713, #10675, #12388, #2330, #20355, #509, #752, #14753, #22731, #4810, #10803, #16852, #10290, #11458, #7155, #11069, #5444, #23355, #15382, #13175, #1017, #7531, #17094, #17358, #19047, #12910, #19309, #19432, #5314, #19170, #25323, #13436, #7015, #7403, #1131, #13047, #21144, #9249, #3104, #22983, #9104, #21406, #25069, #1522, #9491, #5068, #20887, #17474, #21268, #25444, #16970, #15146, #3216, #18933, #24936, #10942, #23114, #5196, #15526, #23231, #11187, #3487, #1265, #8992, #4926, #2974, #17237, #15002, #21025, #25208, #7287, #15263, #13293, #3351, #11326, #1404, #9379, #24003, #17606, #4116, #25708, #3729, #6084, #16042, #8059, #25583, #88, #15652, #21914, #2036, #10004, #5579, #11962, #12095, #23878, #11844, #17999, #14068, #7667, #22034, #11714, #5696, #13810, #1915, #21647 ),
 .UNSPECIFIED., .F., .F. ) 
 B_SPLINE_CURVE_WITH_KNOTS ( ( 3, 2, 2, 2, 2, 2, 2, 2, 2, 2, 2, 2, 2, 2, 2, 2, 2, 2, 2, 2, 2, 2, 2, 2, 2, 2, 2, 2, 2, 2, 2, 2, 2, 2, 2, 2, 2, 2, 2, 2, 2, 2, 2, 2, 2, 2, 2, 2, 2, 2, 2, 2, 2, 2, 2, 2, 2, 2, 2, 2, 3 ),
 ( 0.000000000000000000, 0.01666666666666666644, 0.03333333333333333287, 0.05000000000000000278, 0.06666666666666666574, 0.08333333333333332871, 0.1000000000000000056, 0.1166666666666666685, 0.1333333333333333315, 0.1499999999999999944, 0.1666666666666666574, 0.1833333333333333204, 0.2000000000000000111, 0.2166666666666666741, 0.2333333333333333370, 0.2500000000000000000, 0.2666666666666666630, 0.2833333333333333259, 0.2999999999999999889, 0.3166666666666666519, 0.3333333333333333148, 0.3499999999999999778, 0.3666666666666666408, 0.3833333333333333592, 0.4000000000000000222, 0.4166666666666666852, 0.4333333333333333481, 0.4500000000000000111, 0.4666666666666666741, 0.4833333333333333370, 0.5000000000000000000, 0.5166666666666667185, 0.5333333333333333259, 0.5500000000000000444, 0.5666666666666666519, 0.5833333333333333703, 0.5999999999999999778, 0.6166666666666666963, 0.6333333333333333037, 0.6500000000000000222, 0.6666666666666666297, 0.6833333333333333481, 0.6999999999999999556, 0.7166666666666666741, 0.7333333333333332815, 0.7500000000000000000, 0.7666666666666667185, 0.7833333333333333259, 0.8000000000000000444, 0.8166666666666666519, 0.8333333333333333703, 0.8499999999999999778, 0.8666666666666666963, 0.8833333333333333037, 0.9000000000000000222, 0.9166666666666666297, 0.9333333333333333481, 0.9499999999999999556, 0.9666666666666666741, 0.9833333333333332815, 1.000000000000000000 ),
 .UNSPECIFIED. ) 
 CURVE ( )  GEOMETRIC_REPRESENTATION_ITEM ( )  RATIONAL_B_SPLINE_CURVE ( ( 1.000000000000000000, 0.8660254037844387076, 1.000000000000000000, 0.8660254037844387076, 1.000000000000000000, 0.8660254037844387076, 1.000000000000000000, 0.8660254037844387076, 1.000000000000000000, 0.8660254037844387076, 1.000000000000000000, 0.8660254037844387076, 1.000000000000000000, 0.8660254037844387076, 1.000000000000000000, 0.8660254037844387076, 1.000000000000000000, 0.8660254037844387076, 1.000000000000000000, 0.8660254037844387076, 1.000000000000000000, 0.8660254037844387076, 1.000000000000000000, 0.8660254037844387076, 1.000000000000000000, 0.8660254037844387076, 1.000000000000000000, 0.8660254037844387076, 1.000000000000000000, 0.8660254037844387076, 1.000000000000000000, 0.8660254037844387076, 1.000000000000000000, 0.8660254037844387076, 1.000000000000000000, 0.8660254037844387076, 1.000000000000000000, 0.8660254037844387076, 1.000000000000000000, 0.8660254037844387076, 1.000000000000000000, 0.8660254037844387076, 1.000000000000000000, 0.8660254037844387076, 1.000000000000000000, 0.8660254037844387076, 1.000000000000000000, 0.8660254037844387076, 1.000000000000000000, 0.8660254037844387076, 1.000000000000000000, 0.8660254037844387076, 1.000000000000000000, 0.8660254037844387076, 1.000000000000000000, 0.8660254037844387076, 1.000000000000000000, 0.8660254037844387076, 1.000000000000000000, 0.8660254037844387076, 1.000000000000000000, 0.8660254037844387076, 1.000000000000000000, 0.8660254037844387076, 1.000000000000000000, 0.8660254037844387076, 1.000000000000000000, 0.8660254037844387076, 1.000000000000000000, 0.8660254037844387076, 1.000000000000000000, 0.8660254037844387076, 1.000000000000000000, 0.8660254037844387076, 1.000000000000000000, 0.8660254037844387076, 1.000000000000000000, 0.8660254037844387076, 1.000000000000000000, 0.8660254037844387076, 1.000000000000000000, 0.8660254037844387076, 1.000000000000000000, 0.8660254037844387076, 1.000000000000000000, 0.8660254037844387076, 1.000000000000000000, 0.8660254037844387076, 1.000000000000000000, 0.8660254037844387076, 1.000000000000000000, 0.8660254037844387076, 1.000000000000000000, 0.8660254037844387076, 1.000000000000000000, 0.8660254037844387076, 1.000000000000000000, 0.8660254037844387076, 1.000000000000000000, 0.8660254037844387076, 1.000000000000000000, 0.8660254037844387076, 1.000000000000000000, 0.8660254037844387076, 1.000000000000000000, 0.8660254037844387076, 1.000000000000000000, 0.8660254037844387076, 1.000000000000000000, 0.8660254037844387076, 1.000000000000000000, 0.8660254037844387076, 1.000000000000000000, 0.8660254037844387076, 1.000000000000000000, 0.8660254037844387076, 1.000000000000000000, 0.8660254037844387076, 1.000000000000000000, 0.8660254037844387076, 1.000000000000000000 ) ) 
 REPRESENTATION_ITEM ( '' )  );
#21462=CARTESIAN_POINT ( 'NONE',  ( -3.756430356249997882, 28.21562499938548285, 11.16877607737301226 ) ) ;
#21465=CARTESIAN_POINT ( 'NONE',  ( 21.21320343559646915, 21.21320343559638744, 12.99999999999999289 ) ) ;
#21467=CARTESIAN_POINT ( 'NONE',  ( -1.071796769724494336, -25.75134618820330346, 12.99999999999999467 ) ) ;
#21471=CARTESIAN_POINT ( 'NONE',  ( -2.620986760973688460E-15, -26.18124999877096926, 13.61880215351699874 ) ) ;
#21476=VERTEX_POINT ( 'NONE', #10126 ) ;
#21482=EDGE_LOOP ( 'NONE', ( #10078, #5619, #15330, #10467 ) ) ;
#21483=CARTESIAN_POINT ( 'NONE',  ( -3.756430356250004099, -28.44062499938548783, 6.831223922626973533 ) ) ;
#21484=ORIENTED_EDGE ( 'NONE', *, *, #19509, .F. ) ;
#21492=CARTESIAN_POINT ( 'NONE',  ( 20.00449278107117834, 20.00449278107111084, 13.33755215474602984 ) ) ;
#21495=CARTESIAN_POINT ( 'NONE',  ( -3.999999999999996003, 25.63749999999999929, 6.690598923241487306 ) ) ;
#21502=CARTESIAN_POINT ( 'NONE',  ( 1.071796769724495668, 26.25759618943233065, 12.99999999999999112 ) ) ;
#21504=CARTESIAN_POINT ( 'NONE',  ( -3.959305671612554781E-15, -30.00000000000000355, 12.99999999999999289 ) ) ;
#21513=CARTESIAN_POINT ( 'NONE',  ( 3.735045420075836212E-15, 28.40312499938548640, 4.662447845253954171 ) ) ;
#21516=LINE ( 'NONE', #5188, #2994 ) ;
#21517=CARTESIAN_POINT ( 'NONE',  ( 3.756430356250003211, 27.42812499938548143, 6.831223922626973533 ) ) ;
#21519=DIRECTION ( 'NONE',  ( 0.000000000000000000, 0.000000000000000000, 1.000000000000000000 ) ) ;
#21520=CARTESIAN_POINT ( 'NONE',  ( 17.43018215624843847, 20.25860928099455904, 12.46410161513774639 ) ) ;
#21521=CARTESIAN_POINT ( 'NONE',  ( 22.07732706455164617, 16.76493230863282591, 11.16877607737301226 ) ) ;
#21527=ORIENTED_EDGE ( 'NONE', *, *, #18201, .T. ) ;
#21529=CARTESIAN_POINT ( 'NONE',  ( -4.000000000000003553, -26.83749999999999503, 6.690598923241489970 ) ) ;
#21534=CARTESIAN_POINT ( 'NONE',  ( -26.00000000000000355, -1.592040838891558504E-15, 20.00000599999999906 ) ) ;
#21535=CARTESIAN_POINT ( 'NONE',  ( 3.756430356249997882, -29.45312499938548356, 11.16877607737301226 ) ) ;
#21537=ORIENTED_EDGE ( 'NONE', *, *, #22909, .F. ) ;
#21539=CARTESIAN_POINT ( 'NONE',  ( -2.672651547586948120E-15, -25.59062499938548640, 13.33755215474603162 ) ) ;
#21544=EDGE_CURVE ( 'NONE', #19408, #961, #15956, .T. ) ;
#21545=CARTESIAN_POINT ( 'NONE',  ( -3.469446951953614189E-15, -30.00000000000000355, 8.999999999999992895 ) ) ;
#21548=( BOUNDED_CURVE ( )  B_SPLINE_CURVE ( 2, ( #8952, #7715, #5013, #25155, #970, #17182, #5625, #20976, #15697 ),
 .UNSPECIFIED., .F., .F. ) 
 B_SPLINE_CURVE_WITH_KNOTS ( ( 3, 2, 2, 2, 3 ),
 ( 0.9250000000000000444, 0.9333333333333333481, 0.9499999999999999556, 0.9666666666666666741, 0.9749999999999999778 ),
 .UNSPECIFIED. ) 
 CURVE ( )  GEOMETRIC_REPRESENTATION_ITEM ( )  RATIONAL_B_SPLINE_CURVE ( ( 0.9330127018922194093, 0.9330127018922198534, 1.000000000000000000, 0.8660254037844387076, 1.000000000000000000, 0.8660254037844387076, 1.000000000000000000, 0.9330127018922194093, 0.9330127018922194093 ) ) 
 REPRESENTATION_ITEM ( '' )  );
#21549=CARTESIAN_POINT ( 'NONE',  ( -3.063240906311874401, -29.84319947910909931, 11.57226653943513028 ) ) ;
#21550=CARTESIAN_POINT ( 'NONE',  ( -3.999999999999996447, 26.96874999877096712, 8.999999999999992895 ) ) ;
#21552=CARTESIAN_POINT ( 'NONE',  ( 21.73911410323489690, 16.08225985374244615, 8.999999999999992895 ) ) ;
#21555=CARTESIAN_POINT ( 'NONE',  ( -3.756430356250003655, -29.75312499938548783, 8.999999999999992895 ) ) ;
#21558=CARTESIAN_POINT ( 'NONE',  ( 21.21320343559646915, 21.21320343559638744, 8.999999999999992895 ) ) ;
#21566=VERTEX_POINT ( 'NONE', #24772 ) ;
#21571=CARTESIAN_POINT ( 'NONE',  ( -4.000000000000001776, -28.05624999877096570, 11.30940107675849760 ) ) ;
#21577=CARTESIAN_POINT ( 'NONE',  ( 1.878215178125004048, 28.92812499938548854, 5.746835883940462963 ) ) ;
#21583=CARTESIAN_POINT ( 'NONE',  ( 3.137519842735244810E-15, -27.30624999877096926, 4.999999999999991118 ) ) ;
#21584=CARTESIAN_POINT ( 'NONE',  ( 1.999999999999998224, -27.49374999877096926, 12.46410161513774639 ) ) ;
#21585=CARTESIAN_POINT ( 'NONE',  ( 1.878215178125004048, 28.02812499938548640, 5.746835883940462963 ) ) ;
#21594=EDGE_CURVE ( 'NONE', #21679, #3647, #905, .T. ) ;
#21599=CARTESIAN_POINT ( 'NONE',  ( -1.878215178125000939, -27.42812499938548498, 12.25316411605952283 ) ) ;
#21600=ORIENTED_EDGE ( 'NONE', *, *, #6718, .F. ) ;
#21602=( BOUNDED_CURVE ( )  B_SPLINE_CURVE ( 2, ( #3423, #17033, #23295, #9439, #15460, #5381, #23051, #17420, #16916 ),
 .UNSPECIFIED., .F., .F. ) 
 B_SPLINE_CURVE_WITH_KNOTS ( ( 3, 2, 2, 2, 3 ),
 ( 0.1749999999999999889, 0.1833333333333333204, 0.2000000000000000111, 0.2166666666666666741, 0.2250000000000000056 ),
 .UNSPECIFIED. ) 
 CURVE ( )  GEOMETRIC_REPRESENTATION_ITEM ( )  RATIONAL_B_SPLINE_CURVE ( ( 0.9330127018922194093, 0.9330127018922194093, 1.000000000000000000, 0.8660254037844387076, 1.000000000000000000, 0.8660254037844387076, 1.000000000000000000, 0.9330127018922194093, 0.9330127018922194093 ) ) 
 REPRESENTATION_ITEM ( '' )  );
#21603=ORIENTED_EDGE ( 'NONE', *, *, #769, .F. ) ;
#21604=EDGE_CURVE ( 'NONE', #20539, #21627, #2892, .T. ) ;
#21609=CARTESIAN_POINT ( 'NONE',  ( 17.24222938593383248, 22.55462414185250353, 6.831223922626973533 ) ) ;
#21611=CARTESIAN_POINT ( 'NONE',  ( -3.999999999999996003, 28.33750000000000213, 6.690598923241487306 ) ) ;
#21614=ORIENTED_EDGE ( 'NONE', *, *, #12648, .F. ) ;
#21618=CYLINDRICAL_SURFACE ( 'NONE', #4573, 4.000000000000000000 ) ;
#21622=VERTEX_POINT ( 'NONE', #23072 ) ;
#21627=VERTEX_POINT ( 'NONE', #8560 ) ;
#21634=CARTESIAN_POINT ( 'NONE',  ( 19.66640735175089105, 19.66640735175081289, 4.999999999999992006 ) ) ;
#21636=CARTESIAN_POINT ( 'NONE',  ( 3.735045420075836212E-15, 25.70312499938548001, 4.662447845253954171 ) ) ;
#21638=FACE_OUTER_BOUND ( 'NONE', #14965, .T. ) ;
#21641=CARTESIAN_POINT ( 'NONE',  ( 18.39361514561510447, 18.39361514561503341, 4.381197846482986158 ) ) ;
#21642=CARTESIAN_POINT ( 'NONE',  ( 17.56042743746777646, 22.87282219338644751, 6.831223922626973533 ) ) ;
#21643=CARTESIAN_POINT ( 'NONE',  ( -3.677829432474411853, -29.77381621822422275, 10.59017455026297405 ) ) ;
#21646=CARTESIAN_POINT ( 'NONE',  ( 22.87163432207205460, 19.41484867808718207, 5.822820249163556561 ) ) ;
#21647=CARTESIAN_POINT ( 'NONE',  ( 23.61528431363239022, 18.30288955771356640, 8.999999999999992895 ) ) ;
#21648=CARTESIAN_POINT ( 'NONE',  ( -3.469446951953614189E-15, -30.00000000000000355, 8.999999999999992895 ) ) ;
#21652=CARTESIAN_POINT ( 'NONE',  ( -2.000000000000003997, -25.52500000000000213, 5.535898384862238508 ) ) ;
#21657=CARTESIAN_POINT ( 'NONE',  ( 25.16843286583313599, 6.741346781237259833, 20.00001200000000523 ) ) ;
#21665=AXIS2_PLACEMENT_3D ( 'NONE', #13260, #3189, #18078 ) ;
#21678=CARTESIAN_POINT ( 'NONE',  ( 15.60496277644160124, 21.26181702593391876, 8.999999999999992895 ) ) ;
#21679=VERTEX_POINT ( 'NONE', #11417 ) ;
#21681=CARTESIAN_POINT ( 'NONE',  ( -1.878215178125004048, -29.37812499938548783, 5.746835883940462963 ) ) ;
#21683=CARTESIAN_POINT ( 'NONE',  ( 21.14249275747780032, 15.48563850798535491, 8.999999999999992895 ) ) ;
#21690=CARTESIAN_POINT ( 'NONE',  ( 1.999999999999995781, -26.44374999877096855, 5.535898384862237620 ) ) ;
#21698=FACE_OUTER_BOUND ( 'NONE', #6841, .T. ) ;
#21708=CARTESIAN_POINT ( 'NONE',  ( -3.756430356249996994, 29.07812499938548356, 8.999999999999992895 ) ) ;
#21714=CARTESIAN_POINT ( 'NONE',  ( -1.071796769724494558, -25.93615380933863435, 4.999999999999992895 ) ) ;
#21717=CARTESIAN_POINT ( 'NONE',  ( -4.000000000000003553, -26.29374999877096997, 8.999999999999992895 ) ) ;
#21718=CARTESIAN_POINT ( 'NONE',  ( -3.756430356249997882, 29.11562499938548143, 11.16877607737301226 ) ) ;
#21722=CARTESIAN_POINT ( 'NONE',  ( 3.999999999999996447, -26.06874999877096855, 8.999999999999992895 ) ) ;
#21727=CIRCLE ( 'NONE', #12538, 24.00000000000000355 ) ;
#21730=ORIENTED_EDGE ( 'NONE', *, *, #19464, .F. ) ;
#21731=CARTESIAN_POINT ( 'NONE',  ( 3.756430356249995661, -28.59062499938548640, 6.831223922626973533 ) ) ;
#21735=VERTEX_POINT ( 'NONE', #17189 ) ;
#21742=CARTESIAN_POINT ( 'NONE',  ( 18.96807563933094798, 21.62427301729024975, 12.25316411605951927 ) ) ;
#21744=CARTESIAN_POINT ( 'NONE',  ( 21.21320343559646915, 21.21320343559638744, 8.999999999999992895 ) ) ;
#21748=CARTESIAN_POINT ( 'NONE',  ( 2.000000000000003997, 28.22500000000000142, 5.535898384862238508 ) ) ;
#21749=ADVANCED_FACE ( 'NONE', ( #5659 ), #21364, .F. ) ;
#21752=CARTESIAN_POINT ( 'NONE',  ( 19.49840572522085935, 22.15460310318015758, 5.746835883940462963 ) ) ;
#21753=CARTESIAN_POINT ( 'NONE',  ( -4.000000000000001776, -29.40624999877096357, 11.30940107675849760 ) ) ;
#21757=( BOUNDED_SURFACE ( )  B_SPLINE_SURFACE ( 1, 2, ( 
 ( #4159, #5866, #21830, #12135, #20112, #9529, #12522, #4300, #16713, #20238, #6631, #22736, #2596, #10558, #18557, #6388, #4815, #638, #20498, #22603, #8606, #22337, #24688, #22213, #14758, #8346, #8726, #4419, #24431, #12790, #6509, #18287, #12393, #2216, #12271, #10173, #16334, #6773, #20360, #14493, #18172, #22460, #375, #2455, #253, #4542, #10418, #16587, #10681, #20636, #18417, #8221, #16194, #24546, #513, #24162, #6253, #14243, #2335, #10295, #24302, #14378, #4686, #8484, #16470, #14623, #12665, #2718, #18670, #756, #17242, #10808, #8996, #21030, #8873, #7292, #889, #20762, #20892, #4932, #13052, #21273, #25212, #7160, #5201, #22857, #13180, #23360, #5449, #3356, #10947, #12915, #9384, #15268, #21150, #19052, #24941, #2841, #2979, #23119, #18801, #22988, #23236, #1409, #3109, #3221, #18938, #7021, #1270, #15151, #16857, #15388, #24822, #6899, #19173, #11193, #1137, #5319, #7408, #15007, #13299 ),
 ( #25074, #11331, #19314, #17363, #25328, #14882, #1022, #9254, #16976, #5073, #11074, #9110, #17099, #25712, #21652, #1655, #9632, #9495, #15772, #19435, #21793, #3876, #5583, #15656, #13441, #3492, #17478, #15908, #11847, #25450, #5700, #17610, #25587, #23741, #7671, #11463, #15530, #3734, #23622, #13679, #7535, #5828, #1526, #19818, #1919, #13564, #11718, #21411, #23496, #21529, #23881, #9880, #3611, #19695, #1794, #9762, #13814, #17741, #11580, #19552, #17866, #7793, #25838, #91, #18002, #7921, #13949, #5966, #21917, #8062, #3998, #11965, #19936, #2040, #10008, #16045, #24007, #6349, #22037, #14462, #18378, #22424, #4505, #2301, #478, #215, #14202, #22175, #2555, #14584, #8447, #12360, #12483, #10138, #6597, #16436, #24400, #24262, #2177, #22304, #724, #14342, #8185, #16163, #10524, #4120, #6476, #18521, #16556, #8575, #20456, #608, #12099, #24515, #10647, #22566, #4647, #24126, #12629, #18141, #6212 ) ),
 .UNSPECIFIED., .F., .F., .F. ) 
 B_SPLINE_SURFACE_WITH_KNOTS ( ( 2, 2 ),
 ( 3, 2, 2, 2, 2, 2, 2, 2, 2, 2, 2, 2, 2, 2, 2, 2, 2, 2, 2, 2, 2, 2, 2, 2, 2, 2, 2, 2, 2, 2, 2, 2, 2, 2, 2, 2, 2, 2, 2, 2, 2, 2, 2, 2, 2, 2, 2, 2, 2, 2, 2, 2, 2, 2, 2, 2, 2, 2, 2, 2, 3 ),
 ( 0.000000000000000000, 1.000000000000000000 ),
 ( 0.000000000000000000, 0.01666666666666666644, 0.03333333333333333287, 0.05000000000000000278, 0.06666666666666666574, 0.08333333333333332871, 0.1000000000000000056, 0.1166666666666666685, 0.1333333333333333315, 0.1499999999999999944, 0.1666666666666666574, 0.1833333333333333204, 0.2000000000000000111, 0.2166666666666666741, 0.2333333333333333370, 0.2500000000000000000, 0.2666666666666666630, 0.2833333333333333259, 0.2999999999999999889, 0.3166666666666666519, 0.3333333333333333148, 0.3499999999999999778, 0.3666666666666666408, 0.3833333333333333592, 0.4000000000000000222, 0.4166666666666666852, 0.4333333333333333481, 0.4500000000000000111, 0.4666666666666666741, 0.4833333333333333370, 0.5000000000000000000, 0.5166666666666667185, 0.5333333333333333259, 0.5500000000000000444, 0.5666666666666666519, 0.5833333333333333703, 0.5999999999999999778, 0.6166666666666666963, 0.6333333333333333037, 0.6500000000000000222, 0.6666666666666666297, 0.6833333333333333481, 0.6999999999999999556, 0.7166666666666666741, 0.7333333333333332815, 0.7500000000000000000, 0.7666666666666667185, 0.7833333333333333259, 0.8000000000000000444, 0.8166666666666666519, 0.8333333333333333703, 0.8499999999999999778, 0.8666666666666666963, 0.8833333333333333037, 0.9000000000000000222, 0.9166666666666666297, 0.9333333333333333481, 0.9499999999999999556, 0.9666666666666666741, 0.9833333333333332815, 1.000000000000000000 ),
 .UNSPECIFIED. ) 
 GEOMETRIC_REPRESENTATION_ITEM ( )  RATIONAL_B_SPLINE_SURFACE ( (
 ( 1.000000000000000000, 0.8660254037844387076, 1.000000000000000000, 0.8660254037844387076, 1.000000000000000000, 0.8660254037844387076, 1.000000000000000000, 0.8660254037844387076, 1.000000000000000000, 0.8660254037844387076, 1.000000000000000000, 0.8660254037844387076, 1.000000000000000000, 0.8660254037844387076, 1.000000000000000000, 0.8660254037844387076, 1.000000000000000000, 0.8660254037844387076, 1.000000000000000000, 0.8660254037844387076, 1.000000000000000000, 0.8660254037844387076, 1.000000000000000000, 0.8660254037844387076, 1.000000000000000000, 0.8660254037844387076, 1.000000000000000000, 0.8660254037844387076, 1.000000000000000000, 0.8660254037844387076, 1.000000000000000000, 0.8660254037844387076, 1.000000000000000000, 0.8660254037844387076, 1.000000000000000000, 0.8660254037844387076, 1.000000000000000000, 0.8660254037844387076, 1.000000000000000000, 0.8660254037844387076, 1.000000000000000000, 0.8660254037844387076, 1.000000000000000000, 0.8660254037844387076, 1.000000000000000000, 0.8660254037844387076, 1.000000000000000000, 0.8660254037844387076, 1.000000000000000000, 0.8660254037844387076, 1.000000000000000000, 0.8660254037844387076, 1.000000000000000000, 0.8660254037844387076, 1.000000000000000000, 0.8660254037844387076, 1.000000000000000000, 0.8660254037844387076, 1.000000000000000000, 0.8660254037844387076, 1.000000000000000000, 0.8660254037844387076, 1.000000000000000000, 0.8660254037844387076, 1.000000000000000000, 0.8660254037844387076, 1.000000000000000000, 0.8660254037844387076, 1.000000000000000000, 0.8660254037844387076, 1.000000000000000000, 0.8660254037844387076, 1.000000000000000000, 0.8660254037844387076, 1.000000000000000000, 0.8660254037844387076, 1.000000000000000000, 0.8660254037844387076, 1.000000000000000000, 0.8660254037844387076, 1.000000000000000000, 0.8660254037844387076, 1.000000000000000000, 0.8660254037844387076, 1.000000000000000000, 0.8660254037844387076, 1.000000000000000000, 0.8660254037844387076, 1.000000000000000000, 0.8660254037844387076, 1.000000000000000000, 0.8660254037844387076, 1.000000000000000000, 0.8660254037844387076, 1.000000000000000000, 0.8660254037844387076, 1.000000000000000000, 0.8660254037844387076, 1.000000000000000000, 0.8660254037844387076, 1.000000000000000000, 0.8660254037844387076, 1.000000000000000000, 0.8660254037844387076, 1.000000000000000000, 0.8660254037844387076, 1.000000000000000000, 0.8660254037844387076, 1.000000000000000000, 0.8660254037844387076, 1.000000000000000000, 0.8660254037844387076, 1.000000000000000000, 0.8660254037844387076, 1.000000000000000000, 0.8660254037844387076, 1.000000000000000000, 0.8660254037844387076, 1.000000000000000000, 0.8660254037844387076, 1.000000000000000000),
 ( 1.000000000000000000, 0.8660254037844387076, 1.000000000000000000, 0.8660254037844387076, 1.000000000000000000, 0.8660254037844387076, 1.000000000000000000, 0.8660254037844387076, 1.000000000000000000, 0.8660254037844387076, 1.000000000000000000, 0.8660254037844387076, 1.000000000000000000, 0.8660254037844387076, 1.000000000000000000, 0.8660254037844387076, 1.000000000000000000, 0.8660254037844387076, 1.000000000000000000, 0.8660254037844387076, 1.000000000000000000, 0.8660254037844387076, 1.000000000000000000, 0.8660254037844387076, 1.000000000000000000, 0.8660254037844387076, 1.000000000000000000, 0.8660254037844387076, 1.000000000000000000, 0.8660254037844387076, 1.000000000000000000, 0.8660254037844387076, 1.000000000000000000, 0.8660254037844387076, 1.000000000000000000, 0.8660254037844387076, 1.000000000000000000, 0.8660254037844387076, 1.000000000000000000, 0.8660254037844387076, 1.000000000000000000, 0.8660254037844387076, 1.000000000000000000, 0.8660254037844387076, 1.000000000000000000, 0.8660254037844387076, 1.000000000000000000, 0.8660254037844387076, 1.000000000000000000, 0.8660254037844387076, 1.000000000000000000, 0.8660254037844387076, 1.000000000000000000, 0.8660254037844387076, 1.000000000000000000, 0.8660254037844387076, 1.000000000000000000, 0.8660254037844387076, 1.000000000000000000, 0.8660254037844387076, 1.000000000000000000, 0.8660254037844387076, 1.000000000000000000, 0.8660254037844387076, 1.000000000000000000, 0.8660254037844387076, 1.000000000000000000, 0.8660254037844387076, 1.000000000000000000, 0.8660254037844387076, 1.000000000000000000, 0.8660254037844387076, 1.000000000000000000, 0.8660254037844387076, 1.000000000000000000, 0.8660254037844387076, 1.000000000000000000, 0.8660254037844387076, 1.000000000000000000, 0.8660254037844387076, 1.000000000000000000, 0.8660254037844387076, 1.000000000000000000, 0.8660254037844387076, 1.000000000000000000, 0.8660254037844387076, 1.000000000000000000, 0.8660254037844387076, 1.000000000000000000, 0.8660254037844387076, 1.000000000000000000, 0.8660254037844387076, 1.000000000000000000, 0.8660254037844387076, 1.000000000000000000, 0.8660254037844387076, 1.000000000000000000, 0.8660254037844387076, 1.000000000000000000, 0.8660254037844387076, 1.000000000000000000, 0.8660254037844387076, 1.000000000000000000, 0.8660254037844387076, 1.000000000000000000, 0.8660254037844387076, 1.000000000000000000, 0.8660254037844387076, 1.000000000000000000, 0.8660254037844387076, 1.000000000000000000, 0.8660254037844387076, 1.000000000000000000, 0.8660254037844387076, 1.000000000000000000, 0.8660254037844387076, 1.000000000000000000, 0.8660254037844387076, 1.000000000000000000, 0.8660254037844387076, 1.000000000000000000) ) ) 
 REPRESENTATION_ITEM ( '' )  SURFACE ( )  );
#21760=CARTESIAN_POINT ( 'NONE',  ( 21.21320343559646915, 21.21320343559638744, 4.999999999999992006 ) ) ;
#21762=ORIENTED_EDGE ( 'NONE', *, *, #925, .F. ) ;
#21781=CARTESIAN_POINT ( 'NONE',  ( 19.99344423804966198, 17.16501711330340996, 12.46410161513774817 ) ) ;
#21782=AXIS2_PLACEMENT_3D ( 'NONE', #1385, #25692, #19286 ) ;
#21783=CARTESIAN_POINT ( 'NONE',  ( 16.92403133439988139, 22.23642609031855244, 6.831223922626973533 ) ) ;
#21789=PLANE ( 'NONE',  #22539 ) ;
#21790=DIRECTION ( 'NONE',  ( 0.000000000000000000, 0.000000000000000000, 1.000000000000000000 ) ) ;
#21793=CARTESIAN_POINT ( 'NONE',  ( 1.999999999999998224, -25.75000000000000355, 12.46410161513774639 ) ) ;
#21809=CARTESIAN_POINT ( 'NONE',  ( 19.14933551713917126, 19.14933551713910376, 12.99999999999999289 ) ) ;
#21810=LINE ( 'NONE', #17881, #23478 ) ;
#21811=CARTESIAN_POINT ( 'NONE',  ( 17.83234913717923220, 23.48920338667153729, 8.999999999999992895 ) ) ;
#21816=CARTESIAN_POINT ( 'NONE',  ( 0.000000000000000000, 10.00000000000000000, 15.00000000000000178 ) ) ;
#21818=EDGE_CURVE ( 'NONE', #1926, #2494, #17516, .T. ) ;
#21820=CARTESIAN_POINT ( 'NONE',  ( -3.369928719974892281E-15, -25.11250000000000426, 4.999999999999992006 ) ) ;
#21823=EDGE_CURVE ( 'NONE', #17660, #8728, #5537, .T. ) ;
#21830=CARTESIAN_POINT ( 'NONE',  ( -1.878215178125004048, -25.21562499938548285, 5.746835883940462963 ) ) ;
#21832=ORIENTED_EDGE ( 'NONE', *, *, #24343, .F. ) ;
#21834=VERTEX_POINT ( 'NONE', #37 ) ;
#21836=CARTESIAN_POINT ( 'NONE',  ( -27.10000000000000497, 0.6000000000000000888, 19.59999999999999787 ) ) ;
#21843=CARTESIAN_POINT ( 'NONE',  ( -1.878215178124995832, 29.45312499938548356, 5.746835883940462963 ) ) ;
#21850=CARTESIAN_POINT ( 'NONE',  ( -4.000000000000002665, -29.87009603951200276, 10.45670610619353980 ) ) ;
#21852=CARTESIAN_POINT ( 'NONE',  ( -2.000000000000003997, -28.61874999877096926, 5.535898384862238508 ) ) ;
#21853=CARTESIAN_POINT ( 'NONE',  ( 1.878215178125004048, 27.57812499938548711, 5.746835883940462963 ) ) ;
#21858=CARTESIAN_POINT ( 'NONE',  ( 3.999999999999997335, -26.10624999877096997, 11.30940107675849404 ) ) ;
#21860=CARTESIAN_POINT ( 'NONE',  ( -1.071796769724487675, -29.14240381056766438, 4.999999999999988454 ) ) ;
#21861=CARTESIAN_POINT ( 'NONE',  ( -3.735045420075836212E-15, -28.85312499938548569, 4.662447845253954171 ) ) ;
#21866=CARTESIAN_POINT ( 'NONE',  ( 1.878215178124998497, -26.34062499938548285, 12.25316411605951927 ) ) ;
#21868=CARTESIAN_POINT ( 'NONE',  ( 21.37230246136343581, 18.54387533661716958, 5.535898384862238508 ) ) ;
#21872=CARTESIAN_POINT ( 'NONE',  ( 2.672651547586948120E-15, 26.94062499938548783, 13.33755215474603162 ) ) ;
#21876=CARTESIAN_POINT ( 'NONE',  ( 18.54381157061901675, 21.20000894857831852, 5.746835883940462963 ) ) ;
#21879=CARTESIAN_POINT ( 'NONE',  ( -3.999999999999997335, 29.31250000000000000, 11.30940107675849404 ) ) ;
#21881=CARTESIAN_POINT ( 'NONE',  ( 22.71372316761954480, 17.40132841170072453, 11.16877607737301403 ) ) ;
#21884=ORIENTED_EDGE ( 'NONE', *, *, #19062, .F. ) ;
#21885=ORIENTED_EDGE ( 'NONE', *, *, #23851, .F. ) ;
#21887=ADVANCED_FACE ( 'NONE', ( #172 ), #23828, .F. ) ;
#21890=CARTESIAN_POINT ( 'NONE',  ( 2.000000000000000888, 29.36874999877096926, 12.46410161513774817 ) ) ;
#21904=CARTESIAN_POINT ( 'NONE',  ( 3.756430356250004099, 26.52812499938548285, 6.831223922626973533 ) ) ;
#21907=DIRECTION ( 'NONE',  ( 0.000000000000000000, 1.000000000000000000, 0.000000000000000000 ) ) ;
#21908=CARTESIAN_POINT ( 'NONE',  ( 19.98460540328484214, 19.98460540328476398, 4.381197846482986158 ) ) ;
#21910=CARTESIAN_POINT ( 'NONE',  ( 0.000000000000000000, 10.00000000000000000, 17.00000000000000000 ) ) ;
#21914=CARTESIAN_POINT ( 'NONE',  ( 19.20672417798141041, 21.86292155594071218, 12.25316411605951927 ) ) ;
#21915=ORIENTED_EDGE ( 'NONE', *, *, #18631, .F. ) ;
#21917=CARTESIAN_POINT ( 'NONE',  ( 1.999999999999998224, -27.55000000000000071, 12.46410161513774639 ) ) ;
#21924=DIRECTION ( 'NONE',  ( -0.000000000000000000, -0.000000000000000000, 1.000000000000000000 ) ) ;
#21928=CARTESIAN_POINT ( 'NONE',  ( -3.756430356250003655, -25.25312499938548427, 8.999999999999992895 ) ) ;
#21937=CARTESIAN_POINT ( 'NONE',  ( 19.35704813498177046, 16.52862101023551844, 12.46410161513774817 ) ) ;
#21941=CARTESIAN_POINT ( 'NONE',  ( 15.89664432368105551, 21.55349857317336415, 6.690598923241487306 ) ) ;
#21943=DIRECTION ( 'NONE',  ( 0.000000000000000000, 1.000000000000000000, 0.000000000000000000 ) ) ;
#21947=CARTESIAN_POINT ( 'NONE',  ( 8.831537335106614961E-15, 26.63124999877096855, 12.99999999999999112 ) ) ;
#21952=DIRECTION ( 'NONE',  ( -0.000000000000000000, -0.000000000000000000, -1.000000000000000000 ) ) ;
#21957=ORIENTED_EDGE ( 'NONE', *, *, #12069, .T. ) ;
#21958=EDGE_CURVE ( 'NONE', #961, #9527, #3825, .T. ) ;
#21968=CARTESIAN_POINT ( 'NONE',  ( 2.672651547586948120E-15, 28.74062499938548498, 13.33755215474602984 ) ) ;
#21974=CYLINDRICAL_SURFACE ( 'NONE', #6691, 4.000000000000000000 ) ;
#21976=CARTESIAN_POINT ( 'NONE',  ( 3.999999999999997335, -29.25624999877096499, 11.30940107675849404 ) ) ;
#21977=CARTESIAN_POINT ( 'NONE',  ( 2.672651547586948120E-15, 28.29062499938548569, 13.33755215474602984 ) ) ;
#21979=CARTESIAN_POINT ( 'NONE',  ( -1.057460391440397258E-14, 29.55624999877096926, 4.999999999999992006 ) ) ;
#21980=LINE ( 'NONE', #12165, #23500 ) ;
#21986=ORIENTED_EDGE ( 'NONE', *, *, #15295, .F. ) ;
#21990=ORIENTED_EDGE ( 'NONE', *, *, #6865, .F. ) ;
#21993=CARTESIAN_POINT ( 'NONE',  ( 1.878215178125000939, 27.42812499938548498, 12.25316411605952283 ) ) ;
#21997=CARTESIAN_POINT ( 'NONE',  ( 15.59820611967510295, 20.91060087559377934, 8.999999999999992895 ) ) ;
#22001=CARTESIAN_POINT ( 'NONE',  ( -3.999999999999996003, 28.78750000000000142, 6.690598923241487306 ) ) ;
#22010=CARTESIAN_POINT ( 'NONE',  ( 8.831537335106614961E-15, 26.23749999999999716, 12.99999999999999112 ) ) ;
#22011=CARTESIAN_POINT ( 'NONE',  ( -3.756430356249997882, 25.96562499938548640, 11.16877607737301226 ) ) ;
#22013=CARTESIAN_POINT ( 'NONE',  ( -1.999999999999998224, 27.49374999877096926, 12.46410161513774639 ) ) ;
#22015=CARTESIAN_POINT ( 'NONE',  ( 1.071796769724488563, -25.76740381056766793, 12.99999999999999289 ) ) ;
#22023=CARTESIAN_POINT ( 'NONE',  ( 16.74068927859332234, 19.39688665655263122, 12.25316411605951927 ) ) ;
#22024=CARTESIAN_POINT ( 'NONE',  ( -3.756430356249996994, 25.81562499938548427, 8.999999999999992895 ) ) ;
#22029=CARTESIAN_POINT ( 'NONE',  ( 17.11198410471449094, 19.94041122946061151, 12.46410161513774639 ) ) ;
#22032=CARTESIAN_POINT ( 'NONE',  ( 23.03842281366517852, 17.38156856417272422, 6.690598923241489970 ) ) ;
#22034=CARTESIAN_POINT ( 'NONE',  ( 18.17030703624117294, 23.48270179215985110, 11.16877607737301048 ) ) ;
#22037=CARTESIAN_POINT ( 'NONE',  ( 3.999999999999996447, -27.92500000000000071, 8.999999999999992895 ) ) ;
#22039=EDGE_LOOP ( 'NONE', ( #8545, #25147 ) ) ;
#22041=CARTESIAN_POINT ( 'NONE',  ( -5.577813053751546416E-15, -25.73124999877096997, 12.99999999999999289 ) ) ;
#22042=CARTESIAN_POINT ( 'NONE',  ( 3.834746474454188013E-15, 26.40624999877096357, 4.999999999999992006 ) ) ;
#22055=CARTESIAN_POINT ( 'NONE',  ( 21.21320343559646915, 21.21320343559638744, 12.99999999999999289 ) ) ;
#22059=CARTESIAN_POINT ( 'NONE',  ( 17.51415108564528467, 23.17100533513759331, 8.999999999999992895 ) ) ;
#22061=CARTESIAN_POINT ( 'NONE',  ( 1.999999999999998224, -27.10000000000000142, 12.46410161513774639 ) ) ;
#22062=CARTESIAN_POINT ( 'NONE',  ( 2.444316569969958497, 29.90105888194226580, 5.822820249163556561 ) ) ;
#22069=CARTESIAN_POINT ( 'NONE',  ( 2.000000000000000888, 26.21874999877096712, 12.46410161513774817 ) ) ;
#22071=PLANE ( 'NONE',  #9160 ) ;
#22072=VERTEX_POINT ( 'NONE', #18981 ) ;
#22086=CARTESIAN_POINT ( 'NONE',  ( 3.735045420075836212E-15, 26.15312499938548285, 4.662447845253954171 ) ) ;
#22087=ADVANCED_FACE ( 'NONE', ( #24868, #22900 ), #24596, .T. ) ;
#22095=CARTESIAN_POINT ( 'NONE',  ( -2.000000000000003997, -28.16874999877096997, 5.535898384862238508 ) ) ;
#22096=CARTESIAN_POINT ( 'NONE',  ( -3.756430356249996994, 29.07812499938548356, 8.999999999999992895 ) ) ;
#22097=LINE ( 'NONE', #8246, #24139 ) ;
#22103=CARTESIAN_POINT ( 'NONE',  ( 23.61528431363239022, 18.30288955771356640, 8.999999999999992895 ) ) ;
#22105=VERTEX_POINT ( 'NONE', #18711 ) ;
#22106=ORIENTED_EDGE ( 'NONE', *, *, #2035, .F. ) ;
#22109=ORIENTED_EDGE ( 'NONE', *, *, #5161, .T. ) ;
#22110=ORIENTED_EDGE ( 'NONE', *, *, #23797, .T. ) ;
#22111=CARTESIAN_POINT ( 'NONE',  ( 21.26623644418545211, 18.43780931943919299, 12.46410161513774817 ) ) ;
#22116=CARTESIAN_POINT ( 'NONE',  ( -1.878215178124995832, 25.40312499938548640, 5.746835883940462963 ) ) ;
#22122=CARTESIAN_POINT ( 'NONE',  ( 19.68856820379214057, 17.03237082583270023, 12.25316411605952283 ) ) ;
#22123=( BOUNDED_CURVE ( )  B_SPLINE_CURVE ( 2, ( #6526, #15028, #6916, #8624, #6653 ),
 .UNSPECIFIED., .F., .F. ) 
 B_SPLINE_CURVE_WITH_KNOTS ( ( 3, 2, 3 ),
 ( 0.000000000000000000, 0.01666666666666666644, 0.02500000000000000486 ),
 .UNSPECIFIED. ) 
 CURVE ( )  GEOMETRIC_REPRESENTATION_ITEM ( )  RATIONAL_B_SPLINE_CURVE ( ( 1.000000000000000000, 0.8660254037844387076, 1.000000000000000000, 0.9330127018922192983, 0.9330127018922194093 ) ) 
 REPRESENTATION_ITEM ( '' )  );
#22126=AXIS2_PLACEMENT_3D ( 'NONE', #10711, #4326, #24197 ) ;
#22128=CARTESIAN_POINT ( 'NONE',  ( 3.752267015613588906E-15, 27.81250000000000000, 4.381197846482986158 ) ) ;
#22129=CARTESIAN_POINT ( 'NONE',  ( 3.735045420075836212E-15, 28.40312499938548640, 4.662447845253954171 ) ) ;
#22130=( BOUNDED_CURVE ( )  B_SPLINE_CURVE ( 2, ( #1979, #11291, #4058, #25411, #5900, #7499, #13886, #3943, #9945 ),
 .UNSPECIFIED., .F., .F. ) 
 B_SPLINE_CURVE_WITH_KNOTS ( ( 3, 2, 2, 2, 3 ),
 ( 0.6750000000000000444, 0.6833333333333333481, 0.6999999999999999556, 0.7166666666666666741, 0.7249999999999999778 ),
 .UNSPECIFIED. ) 
 CURVE ( )  GEOMETRIC_REPRESENTATION_ITEM ( )  RATIONAL_B_SPLINE_CURVE ( ( 0.9330127018922194093, 0.9330127018922198534, 1.000000000000000000, 0.8660254037844387076, 1.000000000000000000, 0.8660254037844387076, 1.000000000000000000, 0.9330127018922194093, 0.9330127018922194093 ) ) 
 REPRESENTATION_ITEM ( '' )  );
#22133=CARTESIAN_POINT ( 'NONE',  ( 16.75401129586974491, 19.58243842061586548, 12.46410161513774639 ) ) ;
#22143=CARTESIAN_POINT ( 'NONE',  ( -1.878215178124998497, 26.00312499938548783, 12.25316411605951927 ) ) ;
#22144=CARTESIAN_POINT ( 'NONE',  ( 15.60496277644160124, 21.26181702593391876, 8.999999999999992895 ) ) ;
#22161=CARTESIAN_POINT ( 'NONE',  ( -1.859271017917182139E-15, -28.88124999877096499, 12.99999999999999289 ) ) ;
#22166=CARTESIAN_POINT ( 'NONE',  ( 19.60447174239884305, 22.26066912035814127, 12.25316411605951927 ) ) ;
#22169=CARTESIAN_POINT ( 'NONE',  ( -3.756430356250003211, -25.62812499938548072, 6.831223922626973533 ) ) ;
#22171=VECTOR ( 'NONE', #16994, 1000.000000000000000 ) ;
#22172=CARTESIAN_POINT ( 'NONE',  ( 27.09999999999999787, -0.5999999999999998668, 19.59999999999999787 ) ) ;
#22175=CARTESIAN_POINT ( 'NONE',  ( -3.752267015613588906E-15, -28.26250000000000284, 4.381197846482986158 ) ) ;
#22184=EDGE_LOOP ( 'NONE', ( #6038, #1019, #7620, #12450 ) ) ;
#22185=CARTESIAN_POINT ( 'NONE',  ( 3.756430356249996994, -25.92812499938548498, 8.999999999999992895 ) ) ;
#22187=CARTESIAN_POINT ( 'NONE',  ( 22.05731215476884088, 16.40045790527639369, 8.999999999999992895 ) ) ;
#22193=DIRECTION ( 'NONE',  ( 0.000000000000000000, -0.000000000000000000, 1.000000000000000000 ) ) ;
#22197=CARTESIAN_POINT ( 'NONE',  ( 18.68840298406382416, 17.17265345621170169, 12.99999999999999467 ) ) ;
#22199=CARTESIAN_POINT ( 'NONE',  ( 21.70609600442870857, 16.39370124850988830, 8.999999999999992895 ) ) ;
#22200=CARTESIAN_POINT ( 'NONE',  ( 17.54066758993977970, 23.19752183943208479, 11.30940107675849404 ) ) ;
#22205=CARTESIAN_POINT ( 'NONE',  ( -3.180741987853693331, 29.83126030492351788, 11.43940974718624837 ) ) ;
#22206=ORIENTED_EDGE ( 'NONE', *, *, #24626, .T. ) ;
#22209=CARTESIAN_POINT ( 'NONE',  ( -3.834746474454188013E-15, -27.81249999999999645, 4.999999999999992006 ) ) ;
#22211=DIRECTION ( 'NONE',  ( 0.000000000000000000, -1.000000000000000000, 0.000000000000000000 ) ) ;
#22212=CARTESIAN_POINT ( 'NONE',  ( 2.000000000000003997, 25.46874999877096712, 5.535898384862238508 ) ) ;
#22213=CARTESIAN_POINT ( 'NONE',  ( -3.756430356250002323, -26.00312499938548427, 11.16877607737301226 ) ) ;
#22214=CARTESIAN_POINT ( 'NONE',  ( 27.09999999999999787, -0.5999999999999998668, 19.59999999999999787 ) ) ;
#22215=ORIENTED_EDGE ( 'NONE', *, *, #24972, .F. ) ;
#22228=CARTESIAN_POINT ( 'NONE',  ( 3.756430356250002323, 26.90312499938548640, 11.16877607737301226 ) ) ;
#22236=CARTESIAN_POINT ( 'NONE',  ( -3.752267015613588906E-15, -29.10624999877096997, 4.381197846482986158 ) ) ;
#22239=CARTESIAN_POINT ( 'NONE',  ( -3.999999999999996447, 29.66874999877096997, 8.999999999999992895 ) ) ;
#22240=LINE ( 'NONE', #10319, #18914 ) ;
#22241=VERTEX_POINT ( 'NONE', #21809 ) ;
#22242=DIRECTION ( 'NONE',  ( 0.000000000000000000, 0.000000000000000000, 1.000000000000000000 ) ) ;
#22250=EDGE_LOOP ( 'NONE', ( #10912, #6570, #6112, #21603, #21915 ) ) ;
#22253=ADVANCED_FACE ( 'NONE', ( #108 ), #1931, .T. ) ;
#22254=ORIENTED_EDGE ( 'NONE', *, *, #24592, .T. ) ;
#22257=CARTESIAN_POINT ( 'NONE',  ( -1.878215178124998497, 26.90312499938548285, 12.25316411605951927 ) ) ;
#22261=CARTESIAN_POINT ( 'NONE',  ( 21.04318339706631846, 15.73078864114750530, 11.16877607737301226 ) ) ;
#22268=CARTESIAN_POINT ( 'NONE',  ( -3.756430356249996105, 28.47812499938548569, 6.831223922626973533 ) ) ;
#22270=DIRECTION ( 'NONE',  ( 0.000000000000000000, -1.000000000000000000, 0.000000000000000000 ) ) ;
#22271=FACE_OUTER_BOUND ( 'NONE', #2107, .T. ) ;
#22272=VERTEX_POINT ( 'NONE', #9893 ) ;
#22275=ORIENTED_EDGE ( 'NONE', *, *, #13998, .T. ) ;
#22280=ORIENTED_EDGE ( 'NONE', *, *, #16411, .T. ) ;
#22286=( BOUNDED_CURVE ( )  B_SPLINE_CURVE ( 2, ( #2071, #15942, #23913, #5996, #9665, #17648, #25619, #13978, #21947 ),
 .UNSPECIFIED., .F., .F. ) 
 B_SPLINE_CURVE_WITH_KNOTS ( ( 3, 2, 2, 2, 3 ),
 ( 0.2250000000000000056, 0.2333333333333333370, 0.2500000000000000000, 0.2666666666666666630, 0.2750000000000000222 ),
 .UNSPECIFIED. ) 
 CURVE ( )  GEOMETRIC_REPRESENTATION_ITEM ( )  RATIONAL_B_SPLINE_CURVE ( ( 0.9330127018922194093, 0.9330127018922194093, 1.000000000000000000, 0.8660254037844387076, 1.000000000000000000, 0.8660254037844387076, 1.000000000000000000, 0.9330127018922191873, 0.9330127018922194093 ) ) 
 REPRESENTATION_ITEM ( '' )  );
#22289=CARTESIAN_POINT ( 'NONE',  ( 2.000000000000003997, 26.87500000000000355, 5.535898384862238508 ) ) ;
#22296=CARTESIAN_POINT ( 'NONE',  ( 3.756430356250002323, 27.35312499938547859, 11.16877607737301226 ) ) ;
#22298=VECTOR ( 'NONE', #5184, 1000.000000000000000 ) ;
#22301=CARTESIAN_POINT ( 'NONE',  ( 3.469446951953614189E-15, 30.00000000000000355, 8.999999999999992895 ) ) ;
#22304=CARTESIAN_POINT ( 'NONE',  ( -3.752267015613588906E-15, -28.71250000000000568, 4.381197846482986158 ) ) ;
#22307=ORIENTED_EDGE ( 'NONE', *, *, #22411, .T. ) ;
#22313=CARTESIAN_POINT ( 'NONE',  ( -1.878215178125000939, -27.42812499938548498, 12.25316411605952283 ) ) ;
#22315=DIRECTION ( 'NONE',  ( 0.000000000000000000, -1.000000000000000000, 0.000000000000000000 ) ) ;
#22318=EDGE_CURVE ( 'NONE', #14822, #23126, #25602, .T. ) ;
#22320=CARTESIAN_POINT ( 'NONE',  ( 1.071796769724488563, -28.46740381056766722, 12.99999999999999289 ) ) ;
#22322=CARTESIAN_POINT ( 'NONE',  ( 1.057460391440397258E-14, -29.55624999877096926, 4.999999999999992006 ) ) ;
#22324=CARTESIAN_POINT ( 'NONE',  ( 17.19146985159974150, 19.84766722955904683, 5.746835883940462963 ) ) ;
#22325=CARTESIAN_POINT ( 'NONE',  ( 22.98538980507618845, 17.32853555558373060, 11.30940107675849760 ) ) ;
#22328=CARTESIAN_POINT ( 'NONE',  ( 1.775433037296146654, 29.94838521766437722, 5.406171146379000092 ) ) ;
#22330=CARTESIAN_POINT ( 'NONE',  ( -2.644755406393140440, 29.88376691385261097, 5.987824696368042154 ) ) ;
#22332=CARTESIAN_POINT ( 'NONE',  ( 18.17485398475098535, 18.17485398475091785, 4.662447845253954171 ) ) ;
#22335=CARTESIAN_POINT ( 'NONE',  ( 0.000000000000000000, 0.000000000000000000, 15.00000000000000178 ) ) ;
#22336=CARTESIAN_POINT ( 'NONE',  ( -3.999999999999997335, 26.55624999877096926, 11.30940107675849404 ) ) ;
#22337=CARTESIAN_POINT ( 'NONE',  ( -2.672651547586948120E-15, -25.92812499938548498, 13.33755215474602984 ) ) ;
#22338=CARTESIAN_POINT ( 'NONE',  ( -1.071796769724487230, 25.13259618943233420, 4.999999999999992006 ) ) ;
#22339=EDGE_LOOP ( 'NONE', ( #17450, #2659, #12987, #7227 ) ) ;
#22340=VERTEX_POINT ( 'NONE', #1811 ) ;
#22341=CARTESIAN_POINT ( 'NONE',  ( -2.672651547586948120E-15, -29.64062499938548356, 13.33755215474602984 ) ) ;
#22349=CARTESIAN_POINT ( 'NONE',  ( -3.756430356249997882, 27.20312499938548001, 11.16877607737301226 ) ) ;
#22350=EDGE_CURVE ( 'NONE', #9107, #13049, #23133, .T. ) ;
#22356=CARTESIAN_POINT ( 'NONE',  ( 1.859271017917182139E-15, 29.78124999877096712, 12.99999999999999289 ) ) ;
#22357=CARTESIAN_POINT ( 'NONE',  ( 3.999999999999996003, -28.28124999877096712, 6.690598923241487306 ) ) ;
#22362=FACE_OUTER_BOUND ( 'NONE', #24103, .T. ) ;
#22363=EDGE_LOOP ( 'NONE', ( #9915, #13242, #9802 ) ) ;
#22376=CARTESIAN_POINT ( 'NONE',  ( 3.735045420075836212E-15, 25.36562499938548854, 4.662447845253954171 ) ) ;
#22378=CARTESIAN_POINT ( 'NONE',  ( 0.000000000000000000, 0.000000000000000000, 20.00000000000000000 ) ) ;
#22380=CARTESIAN_POINT ( 'NONE',  ( 16.97933781724378122, 19.63553519520309010, 12.25316411605951927 ) ) ;
#22383=DIRECTION ( 'NONE',  ( 0.000000000000000000, 1.000000000000000000, -0.000000000000000000 ) ) ;
#22385=CARTESIAN_POINT ( 'NONE',  ( -1.999999999999998224, 27.94374999877096855, 12.46410161513774639 ) ) ;
#22387=CARTESIAN_POINT ( 'NONE',  ( 3.756430356250002323, 29.15312499938548640, 11.16877607737301403 ) ) ;
#22389=ADVANCED_FACE ( 'NONE', ( #24664 ), #12501, .F. ) ;
#22390=FACE_OUTER_BOUND ( 'NONE', #6474, .T. ) ;
#22392=( BOUNDED_CURVE ( )  B_SPLINE_CURVE ( 2, ( #20861, #3468, #21006, #11440, #995, #13157, #21121, #8976, #24919 ),
 .UNSPECIFIED., .F., .F. ) 
 B_SPLINE_CURVE_WITH_KNOTS ( ( 3, 2, 2, 2, 3 ),
 ( 0.1250000000000000000, 0.1333333333333333315, 0.1499999999999999944, 0.1666666666666666574, 0.1749999999999999889 ),
 .UNSPECIFIED. ) 
 CURVE ( )  GEOMETRIC_REPRESENTATION_ITEM ( )  RATIONAL_B_SPLINE_CURVE ( ( 0.9330127018922194093, 0.9330127018922194093, 1.000000000000000000, 0.8660254037844387076, 1.000000000000000000, 0.8660254037844387076, 1.000000000000000000, 0.9330127018922194093, 0.9330127018922194093 ) ) 
 REPRESENTATION_ITEM ( '' )  );
#22393=EDGE_CURVE ( 'NONE', #9154, #12924, #16569, .T. ) ;
#22402=EDGE_LOOP ( 'NONE', ( #1199, #11263, #8962 ) ) ;
#22411=EDGE_CURVE ( 'NONE', #8734, #22340, #16839, .T. ) ;
#22413=CARTESIAN_POINT ( 'NONE',  ( 3.756430356250004099, 26.97812499938548569, 6.831223922626973533 ) ) ;
#22419=DIRECTION ( 'NONE',  ( -0.000000000000000000, -0.000000000000000000, 1.000000000000000000 ) ) ;
#22420=CARTESIAN_POINT ( 'NONE',  ( 3.756430356249996105, -26.22812499938548214, 6.831223922626973533 ) ) ;
#22424=CARTESIAN_POINT ( 'NONE',  ( -2.620986760973688460E-15, -28.03750000000000142, 13.61880215351699874 ) ) ;
#22428=ORIENTED_EDGE ( 'NONE', *, *, #11237, .F. ) ;
#22429=( BOUNDED_CURVE ( )  B_SPLINE_CURVE ( 2, ( #21979, #4322, #10318, #16102, #22239, #2361, #2105, #19874, #24066 ),
 .UNSPECIFIED., .F., .F. ) 
 B_SPLINE_CURVE_WITH_KNOTS ( ( 3, 2, 2, 2, 3 ),
 ( 0.9250000000000000444, 0.9333333333333333481, 0.9499999999999999556, 0.9666666666666666741, 0.9749999999999999778 ),
 .UNSPECIFIED. ) 
 CURVE ( )  GEOMETRIC_REPRESENTATION_ITEM ( )  RATIONAL_B_SPLINE_CURVE ( ( 0.9330127018922194093, 0.9330127018922198534, 1.000000000000000000, 0.8660254037844387076, 1.000000000000000000, 0.8660254037844387076, 1.000000000000000000, 0.9330127018922194093, 0.9330127018922194093 ) ) 
 REPRESENTATION_ITEM ( '' )  );
#22436=CARTESIAN_POINT ( 'NONE',  ( 3.756430356249997438, -27.76562499938549067, 11.16877607737301048 ) ) ;
#22438=( BOUNDED_CURVE ( )  B_SPLINE_CURVE ( 2, ( #12949, #17389, #15423, #7436, #23395, #20788, #10842, #11105, #926 ),
 .UNSPECIFIED., .F., .F. ) 
 B_SPLINE_CURVE_WITH_KNOTS ( ( 3, 2, 2, 2, 3 ),
 ( 0.7750000000000000222, 0.7833333333333333259, 0.8000000000000000444, 0.8166666666666666519, 0.8250000000000000666 ),
 .UNSPECIFIED. ) 
 CURVE ( )  GEOMETRIC_REPRESENTATION_ITEM ( )  RATIONAL_B_SPLINE_CURVE ( ( 0.9330127018922194093, 0.9330127018922194093, 1.000000000000000000, 0.8660254037844387076, 1.000000000000000000, 0.8660254037844387076, 1.000000000000000000, 0.9330127018922189652, 0.9330127018922194093 ) ) 
 REPRESENTATION_ITEM ( '' )  );
#22443=CARTESIAN_POINT ( 'NONE',  ( -1.859271017917182139E-15, -28.48749999999999716, 12.99999999999999289 ) ) ;
#22445=AXIS2_PLACEMENT_3D ( 'NONE', #18105, #17573, #180 ) ;
#22448=CARTESIAN_POINT ( 'NONE',  ( 20.43103032403801578, 17.77483294607857189, 5.746835883940462963 ) ) ;
#22449=CARTESIAN_POINT ( 'NONE',  ( 19.94483064597403299, 19.94483064597396194, 4.381197846482986158 ) ) ;
#22450=DIRECTION ( 'NONE',  ( 0.000000000000000000, 1.000000000000000000, 0.000000000000000000 ) ) ;
#22451=LINE ( 'NONE', #14749, #21360 ) ;
#22453=CARTESIAN_POINT ( 'NONE',  ( -1.036406108997123487, 29.98318460927812268, 5.127803451112008304 ) ) ;
#22456=CARTESIAN_POINT ( 'NONE',  ( 21.77888886054569539, 16.12203461105324820, 8.999999999999992895 ) ) ;
#22457=ORIENTED_EDGE ( 'NONE', *, *, #14170, .T. ) ;
#22460=CARTESIAN_POINT ( 'NONE',  ( 3.756430356249995661, -26.67812499938548498, 6.831223922626973533 ) ) ;
#22463=ORIENTED_EDGE ( 'NONE', *, *, #25163, .T. ) ;
#22464=CARTESIAN_POINT ( 'NONE',  ( 15.92316082797555055, 21.58001507746786274, 8.999999999999992895 ) ) ;
#22467=CARTESIAN_POINT ( 'NONE',  ( 3.756430356249995661, -26.22812499938548214, 6.831223922626973533 ) ) ;
#22478=CARTESIAN_POINT ( 'NONE',  ( 21.05852382634284936, 21.05852382634277831, 12.99999999999999289 ) ) ;
#22479=CARTESIAN_POINT ( 'NONE',  ( 3.756430356250004099, 25.62812499938548072, 6.831223922626973533 ) ) ;
#22480=CARTESIAN_POINT ( 'NONE',  ( 18.38477631085027753, 21.21320343559639454, 12.46410161513774639 ) ) ;
#22486=CARTESIAN_POINT ( 'NONE',  ( -3.756430356250003655, -27.95312499938548711, 8.999999999999992895 ) ) ;
#22495=ORIENTED_EDGE ( 'NONE', *, *, #24165, .F. ) ;
#22498=ORIENTED_EDGE ( 'NONE', *, *, #23220, .F. ) ;
#22502=EDGE_LOOP ( 'NONE', ( #19242, #24307, #20495, #7930, #2720 ) ) ;
#22503=VERTEX_POINT ( 'NONE', #11808 ) ;
#22504=CYLINDRICAL_SURFACE ( 'NONE', #25165, 4.000000000000000000 ) ;
#22507=CARTESIAN_POINT ( 'NONE',  ( 3.756430356250003211, 28.44062499938548427, 6.831223922626973533 ) ) ;
#22514=CARTESIAN_POINT ( 'NONE',  ( 15.57168961538060969, 20.88408437129928785, 6.831223922626973533 ) ) ;
#22516=CYLINDRICAL_SURFACE ( 'NONE', #41, 0.7500000000000001110 ) ;
#22517=AXIS2_PLACEMENT_3D ( 'NONE', #9356, #7381, #10913 ) ;
#22526=CARTESIAN_POINT ( 'NONE',  ( 4.000000000000003553, 27.64374999877096784, 8.999999999999992895 ) ) ;
#22539=AXIS2_PLACEMENT_3D ( 'NONE', #11576, #9627, #3607 ) ;
#22544=CARTESIAN_POINT ( 'NONE',  ( 1.859271017917182139E-15, 28.93749999999999645, 12.99999999999999289 ) ) ;
#22545=VECTOR ( 'NONE', #8909, 1000.000000000000000 ) ;
#22547=CARTESIAN_POINT ( 'NONE',  ( -3.999999999999995559, 28.28124999877096712, 6.690598923241487306 ) ) ;
#22552=( BOUNDED_CURVE ( )  B_SPLINE_CURVE ( 2, ( #12678, #2730, #10694, #18681, #8618, #16597, #24701, #767, #12404 ),
 .UNSPECIFIED., .F., .F. ) 
 B_SPLINE_CURVE_WITH_KNOTS ( ( 3, 2, 2, 2, 3 ),
 ( 0.5750000000000000666, 0.5833333333333333703, 0.5999999999999999778, 0.6166666666666666963, 0.6250000000000000000 ),
 .UNSPECIFIED. ) 
 CURVE ( )  GEOMETRIC_REPRESENTATION_ITEM ( )  RATIONAL_B_SPLINE_CURVE ( ( 0.9330127018922194093, 0.9330127018922198534, 1.000000000000000000, 0.8660254037844387076, 1.000000000000000000, 0.8660254037844387076, 1.000000000000000000, 0.9330127018922194093, 0.9330127018922194093 ) ) 
 REPRESENTATION_ITEM ( '' )  );
#22553=CARTESIAN_POINT ( 'NONE',  ( 2.672651547586948120E-15, 27.27812499938548285, 13.33755215474602984 ) ) ;
#22555=CARTESIAN_POINT ( 'NONE',  ( 20.85756786700484966, 15.54517311108603295, 6.831223922626973533 ) ) ;
#22557=CARTESIAN_POINT ( 'NONE',  ( -1.057460391440397258E-14, 29.16249999999999787, 4.999999999999992006 ) ) ;
#22558=CARTESIAN_POINT ( 'NONE',  ( 3.999999999999996447, -27.86874999877096570, 8.999999999999992895 ) ) ;
#22559=CARTESIAN_POINT ( 'NONE',  ( 3.756430356249996994, -26.71562499938548285, 8.999999999999992895 ) ) ;
#22562=B_SPLINE_CURVE_WITH_KNOTS ( 'NONE', 3,
 ( #6196, #10243, #10127, #18240, #6335, #4370, #14328, #4492 ),
 .UNSPECIFIED., .F., .F.,
 ( 4, 2, 2, 4 ),
 ( 0.01599790909976502723, 0.01669365098321972177, 0.01738939286667441630, 0.01878087663358380885 ),
 .UNSPECIFIED. ) ;
#22563=VERTEX_POINT ( 'NONE', #17823 ) ;
#22566=CARTESIAN_POINT ( 'NONE',  ( 3.999999999999997335, -29.31250000000000000, 11.30940107675849404 ) ) ;
#22575=CARTESIAN_POINT ( 'NONE',  ( -3.756430356250003211, -27.09062499938548640, 6.831223922626973533 ) ) ;
#22577=CARTESIAN_POINT ( 'NONE',  ( 20.59006558380675855, 17.76163845906049943, 12.46410161513774817 ) ) ;
#22581=EDGE_CURVE ( 'NONE', #22072, #14590, #2962, .T. ) ;
#22588=CARTESIAN_POINT ( 'NONE',  ( 3.999999999999997335, -28.35624999877096997, 11.30940107675849404 ) ) ;
#22589=CARTESIAN_POINT ( 'NONE',  ( 16.55280027427694378, 21.86519503019561839, 8.999999999999992895 ) ) ;
#22590=CARTESIAN_POINT ( 'NONE',  ( 20.58122674904193516, 20.58122674904185345, 4.381197846482986158 ) ) ;
#22592=DIRECTION ( 'NONE',  ( -0.000000000000000000, -1.000000000000000000, -0.000000000000000000 ) ) ;
#22602=CARTESIAN_POINT ( 'NONE',  ( 2.000000000000003997, 28.61874999877096926, 5.535898384862238508 ) ) ;
#22603=CARTESIAN_POINT ( 'NONE',  ( 3.756430356249997882, -25.85312499938548925, 11.16877607737301226 ) ) ;
#22606=( BOUNDED_CURVE ( )  B_SPLINE_CURVE ( 2, ( #18324, #23958, #22111, #4066, #16235, #10084, #21868, #14287, #2252 ),
 .UNSPECIFIED., .F., .T. ) 
 B_SPLINE_CURVE_WITH_KNOTS ( ( 3, 2, 2, 2, 3 ),
 ( 0.6750000000000000444, 0.6833333333333333481, 0.6999999999999999556, 0.7166666666666666741, 0.7249999999999999778 ),
 .UNSPECIFIED. ) 
 CURVE ( )  GEOMETRIC_REPRESENTATION_ITEM ( )  RATIONAL_B_SPLINE_CURVE ( ( 0.9330127018922194093, 0.9330127018922198534, 1.000000000000000000, 0.8660254037844387076, 1.000000000000000000, 0.8660254037844387076, 1.000000000000000000, 0.9330127018922194093, 0.9330127018922194093 ) ) 
 REPRESENTATION_ITEM ( '' )  );
#22609=CARTESIAN_POINT ( 'NONE',  ( -3.756430356250004099, -26.52812499938548285, 6.831223922626973533 ) ) ;
#22616=AXIS2_PLACEMENT_3D ( 'NONE', #17228, #15254, #11955 ) ;
#22621=CARTESIAN_POINT ( 'NONE',  ( 3.756430356250003655, 28.29062499938548569, 8.999999999999992895 ) ) ;
#22623=CARTESIAN_POINT ( 'NONE',  ( 23.34336261392093093, 17.68650836442847663, 11.30940107675849760 ) ) ;
#22630=CARTESIAN_POINT ( 'NONE',  ( 1.878215178124998497, -26.00312499938548783, 12.25316411605951927 ) ) ;
#22632=CARTESIAN_POINT ( 'NONE',  ( 3.756430356250002323, 29.71562499938548640, 11.16877607737301226 ) ) ;
#22636=CARTESIAN_POINT ( 'NONE',  ( -25.99307600111999150, 0.5999999999999998668, 19.59999999999999787 ) ) ;
#22639=LINE ( 'NONE', #6540, #19990 ) ;
#22644=ORIENTED_EDGE ( 'NONE', *, *, #8813, .T. ) ;
#22647=ORIENTED_EDGE ( 'NONE', *, *, #4922, .F. ) ;
#22649=CARTESIAN_POINT ( 'NONE',  ( -3.756430356249996994, 28.17812499938548498, 8.999999999999992895 ) ) ;
#22658=CARTESIAN_POINT ( 'NONE',  ( 26.00000000000000711, -1.701696020694468015, 20.00001200000000168 ) ) ;
#22662=CARTESIAN_POINT ( 'NONE',  ( -3.999999999999996447, 27.86874999877096570, 8.999999999999992895 ) ) ;
#22663=CARTESIAN_POINT ( 'NONE',  ( 0.000000000000000000, 0.000000000000000000, 19.00000000000000000 ) ) ;
#22678=CARTESIAN_POINT ( 'NONE',  ( -3.756430356250004099, -25.74062499938548143, 6.831223922626973533 ) ) ;
#22680=DIRECTION ( 'NONE',  ( 1.000000000000000000, 0.000000000000000000, -0.000000000000000000 ) ) ;
#22684=CARTESIAN_POINT ( 'NONE',  ( 16.25461713252580509, 21.91147138201811373, 6.690598923241487306 ) ) ;
#22687=CARTESIAN_POINT ( 'NONE',  ( 20.83105136271035462, 15.51865660679153969, 8.999999999999992895 ) ) ;
#22690=CARTESIAN_POINT ( 'NONE',  ( -3.756430356249996994, 27.16562499938548214, 8.999999999999992895 ) ) ;
#22691=EDGE_CURVE ( 'NONE', #990, #12604, #20287, .T. ) ;
#22693=CARTESIAN_POINT ( 'NONE',  ( 19.74153744638290320, 16.91311032163664407, 5.535898384862238508 ) ) ;
#22695=CARTESIAN_POINT ( 'NONE',  ( 21.21320343559646915, 21.21320343559638744, 4.999999999999992006 ) ) ;
#22698=CARTESIAN_POINT ( 'NONE',  ( 3.756430356249996994, -27.16562499938548214, 8.999999999999992895 ) ) ;
#22703=CARTESIAN_POINT ( 'NONE',  ( 1.427366165835751044, 29.96717973704832261, 12.74788474329069921 ) ) ;
#22705=VERTEX_POINT ( 'NONE', #5129 ) ;
#22706=VERTEX_POINT ( 'NONE', #14810 ) ;
#22710=CARTESIAN_POINT ( 'NONE',  ( -3.756430356250002323, -27.01562499938548356, 11.16877607737301403 ) ) ;
#22713=( GEOMETRIC_REPRESENTATION_CONTEXT ( 3 ) GLOBAL_UNCERTAINTY_ASSIGNED_CONTEXT ( ( #10700 ) ) GLOBAL_UNIT_ASSIGNED_CONTEXT ( ( #1847, #13727, #7839 ) ) REPRESENTATION_CONTEXT ( 'NONE', 'WORKASPACE' ) );
#22721=EDGE_CURVE ( 'NONE', #21735, #18967, #25530, .T. ) ;
#22723=CARTESIAN_POINT ( 'NONE',  ( 3.999999999999995559, -28.28124999877096712, 6.690598923241487306 ) ) ;
#22724=CARTESIAN_POINT ( 'NONE',  ( 20.64316235839397962, 17.98696498043453573, 12.25316411605952283 ) ) ;
#22725=CARTESIAN_POINT ( 'NONE',  ( 16.02247018838703241, 21.33486494430570701, 11.16877607737301226 ) ) ;
#22726=CARTESIAN_POINT ( 'NONE',  ( 3.369928719974892281E-15, 25.50624999877096855, 4.999999999999992006 ) ) ;
#22727=DIRECTION ( 'NONE',  ( 0.2588190451025209615, -0.9659258262890682012, 0.000000000000000000 ) ) ;
#22731=CARTESIAN_POINT ( 'NONE',  ( 21.06969990136081705, 15.75730514544200211, 8.999999999999992895 ) ) ;
#22732=FACE_OUTER_BOUND ( 'NONE', #19061, .T. ) ;
#22735=CARTESIAN_POINT ( 'NONE',  ( 2.620986760973688460E-15, 27.53124999877097068, 13.61880215351699874 ) ) ;
#22736=CARTESIAN_POINT ( 'NONE',  ( -3.756430356250002323, -25.55312499938548143, 11.16877607737301226 ) ) ;
#22739=DIRECTION ( 'NONE',  ( 0.000000000000000000, 1.000000000000000000, 0.000000000000000000 ) ) ;
#22741=CARTESIAN_POINT ( 'NONE',  ( -2.672651547586948120E-15, -25.47812499938548569, 13.33755215474602984 ) ) ;
#22752=CARTESIAN_POINT ( 'NONE',  ( 3.756430356250004099, 28.32812499938548356, 6.831223922626973533 ) ) ;
#22756=CARTESIAN_POINT ( 'NONE',  ( 3.137519842735244810E-15, -26.46249999999999858, 4.999999999999991118 ) ) ;
#22757=CARTESIAN_POINT ( 'NONE',  ( 4.000000000000003553, 25.88124999877096855, 6.690598923241489970 ) ) ;
#22759=CARTESIAN_POINT ( 'NONE',  ( -3.756430356250004099, -27.54062499938548569, 6.831223922626973533 ) ) ;
#22760=CARTESIAN_POINT ( 'NONE',  ( -3.756430356249996994, 29.52812499938548640, 8.999999999999992895 ) ) ;
#22761=CARTESIAN_POINT ( 'NONE',  ( -27.10000000000000497, -0.5999999999999998668, 19.00000000000000000 ) ) ;
#22763=CARTESIAN_POINT ( 'NONE',  ( 3.469446951953614189E-15, 25.00000000000000000, 8.999999999999992895 ) ) ;
#22774=CARTESIAN_POINT ( 'NONE',  ( -4.000000000000003553, -27.70000000000000284, 8.999999999999992895 ) ) ;
#22775=EDGE_CURVE ( 'NONE', #23711, #476, #12579, .T. ) ;
#22778=CARTESIAN_POINT ( 'NONE',  ( 1.878215178125000939, 29.22812499938548569, 12.25316411605952283 ) ) ;
#22781=CARTESIAN_POINT ( 'NONE',  ( 23.27056975780394765, 17.95817500188513094, 11.16877607737301226 ) ) ;
#22782=CARTESIAN_POINT ( 'NONE',  ( -1.878215178124998497, 26.45312499938548711, 12.25316411605951927 ) ) ;
#22783=CARTESIAN_POINT ( 'NONE',  ( -24.67207871933483432, -8.377607117416806304, 20.00001200000000168 ) ) ;
#22789=LINE ( 'NONE', #18990, #25517 ) ;
#22791=CARTESIAN_POINT ( 'NONE',  ( 3.999999999999996447, -26.57500000000000284, 8.999999999999992895 ) ) ;
#22794=ORIENTED_EDGE ( 'NONE', *, *, #19243, .T. ) ;
#22799=CARTESIAN_POINT ( 'NONE',  ( -1.878215178125004048, -25.77812499938548640, 5.746835883940462963 ) ) ;
#22804=ORIENTED_EDGE ( 'NONE', *, *, #25823, .F. ) ;
#22805=LINE ( 'NONE', #9194, #9738 ) ;
#22811=CARTESIAN_POINT ( 'NONE',  ( -1.071796769724487230, 28.22634618820330132, 4.999999999999992006 ) ) ;
#22812=CARTESIAN_POINT ( 'NONE',  ( 18.01348148472910893, 20.66967886268841426, 12.25316411605951927 ) ) ;
#22814=CARTESIAN_POINT ( 'NONE',  ( -3.756430356249997882, 27.20312499938548001, 11.16877607737301226 ) ) ;
#22816=CARTESIAN_POINT ( 'NONE',  ( 20.79777820164935775, 15.14092395215691234, 11.30940107675849760 ) ) ;
#22820=CARTESIAN_POINT ( 'NONE',  ( -2.672651547586948120E-15, -26.82812499938548356, 13.33755215474603162 ) ) ;
#22829=( BOUNDED_CURVE ( )  B_SPLINE_CURVE ( 2, ( #23420, #21467, #19231, #1460, #17676, #5635, #3661, #21714, #25376 ),
 .UNSPECIFIED., .F., .F. ) 
 B_SPLINE_CURVE_WITH_KNOTS ( ( 3, 2, 2, 2, 3 ),
 ( 0.07500000000000001110, 0.08333333333333332871, 0.1000000000000000056, 0.1166666666666666685, 0.1250000000000000000 ),
 .UNSPECIFIED. ) 
 CURVE ( )  GEOMETRIC_REPRESENTATION_ITEM ( )  RATIONAL_B_SPLINE_CURVE ( ( 0.9330127018922192983, 0.9330127018922194093, 1.000000000000000000, 0.8660254037844387076, 1.000000000000000000, 0.8660254037844387076, 1.000000000000000000, 0.9330127018922194093, 0.9330127018922194093 ) ) 
 REPRESENTATION_ITEM ( '' )  );
#22833=CARTESIAN_POINT ( 'NONE',  ( -1.878215178125000939, -29.67812499938548498, 12.25316411605952283 ) ) ;
#22842=CARTESIAN_POINT ( 'NONE',  ( 1.999999999999998224, -28.44999999999999929, 12.46410161513774639 ) ) ;
#22844=CARTESIAN_POINT ( 'NONE',  ( -3.756430356249996994, 25.36562499938548498, 8.999999999999992895 ) ) ;
#22845=CARTESIAN_POINT ( 'NONE',  ( 1.071796769724487230, -28.22634618820330132, 4.999999999999992006 ) ) ;
#22846=CARTESIAN_POINT ( 'NONE',  ( 19.20672417798141041, 21.86292155594071218, 12.25316411605951927 ) ) ;
#22847=CARTESIAN_POINT ( 'NONE',  ( 17.69528343319515784, 20.35148081115446317, 12.25316411605951927 ) ) ;
#22856=CARTESIAN_POINT ( 'NONE',  ( 2.620986760973688460E-15, 28.88124999877096855, 13.61880215351699874 ) ) ;
#22857=CARTESIAN_POINT ( 'NONE',  ( -3.756430356250004099, -28.32812499938548356, 6.831223922626973533 ) ) ;
#22860=CARTESIAN_POINT ( 'NONE',  ( -3.834746474454188013E-15, -25.95624999877096428, 4.999999999999992006 ) ) ;
#22862=CARTESIAN_POINT ( 'NONE',  ( 1.878215178124998497, -29.04062499938548569, 12.25316411605951927 ) ) ;
#22864=VERTEX_POINT ( 'NONE', #11388 ) ;
#22871=CARTESIAN_POINT ( 'NONE',  ( -3.756430356249997882, 28.10312499938548569, 11.16877607737301226 ) ) ;
#22878=DIRECTION ( 'NONE',  ( -0.7071067811865487940, -0.7071067811865463515, 0.000000000000000000 ) ) ;
#22879=CARTESIAN_POINT ( 'NONE',  ( 3.756430356249995661, -27.69062499938548427, 6.831223922626973533 ) ) ;
#22884=ORIENTED_EDGE ( 'NONE', *, *, #17433, .T. ) ;
#22885=CARTESIAN_POINT ( 'NONE',  ( -27.10000000000000497, -0.5999999999999998668, 19.00000000000000000 ) ) ;
#22891=ORIENTED_EDGE ( 'NONE', *, *, #15019, .F. ) ;
#22892=ORIENTED_EDGE ( 'NONE', *, *, #7271, .T. ) ;
#22895=ORIENTED_EDGE ( 'NONE', *, *, #12571, .F. ) ;
#22900=FACE_OUTER_BOUND ( 'NONE', #8975, .T. ) ;
#22901=CARTESIAN_POINT ( 'NONE',  ( 17.48087792458429135, 22.79327268050296240, 6.831223922626973533 ) ) ;
#22903=CARTESIAN_POINT ( 'NONE',  ( -3.756430356249997882, 26.41562499938548569, 11.16877607737301226 ) ) ;
#22904=CARTESIAN_POINT ( 'NONE',  ( 13.02991752792604174, -22.56362157461193263, 20.00001200000000168 ) ) ;
#22909=EDGE_CURVE ( 'NONE', #24428, #9293, #11437, .T. ) ;
#22911=CARTESIAN_POINT ( 'NONE',  ( -4.000000000000003553, -25.39374999877096784, 8.999999999999992895 ) ) ;
#22921=EDGE_LOOP ( 'NONE', ( #3971, #22457, #5456, #20119 ) ) ;
#22925=AXIS2_PLACEMENT_3D ( 'NONE', #1263, #20628, #14752 ) ;
#22934=CARTESIAN_POINT ( 'NONE',  ( 17.27101936448323016, 19.92721674244253549, 5.746835883940462963 ) ) ;
#22937=CARTESIAN_POINT ( 'NONE',  ( -1.999999999999998224, 26.20000000000000284, 12.46410161513774639 ) ) ;
#22939=CARTESIAN_POINT ( 'NONE',  ( 18.54381157061901675, 21.20000894857831852, 5.746835883940462963 ) ) ;
#22940=CARTESIAN_POINT ( 'NONE',  ( 4.000000000000003553, 26.74374999877096926, 8.999999999999992895 ) ) ;
#22946=CARTESIAN_POINT ( 'NONE',  ( 1.878215178124995832, -28.44062499938548427, 5.746835883940462963 ) ) ;
#22950=CARTESIAN_POINT ( 'NONE',  ( -27.10000000000000497, -0.5999999999999998668, 19.00000000000000000 ) ) ;
#22957=CARTESIAN_POINT ( 'NONE',  ( -3.756430356250002323, -28.81562499938548427, 11.16877607737301403 ) ) ;
#22968=( BOUNDED_CURVE ( )  B_SPLINE_CURVE ( 2, ( #1821, #9279, #19460, #23390, #23143 ),
 .UNSPECIFIED., .F., .F. ) 
 B_SPLINE_CURVE_WITH_KNOTS ( ( 3, 2, 3 ),
 ( 0.9749999999999999778, 0.9833333333333332815, 0.9889400238386636399 ),
 .UNSPECIFIED. ) 
 CURVE ( )  GEOMETRIC_REPRESENTATION_ITEM ( )  RATIONAL_B_SPLINE_CURVE ( ( 0.9330127018922194093, 0.9330127018922194093, 1.000000000000000000, 0.9549307542065648136, 0.9401842259098239785 ) ) 
 REPRESENTATION_ITEM ( '' )  );
#22972=CARTESIAN_POINT ( 'NONE',  ( -1.878215178124998497, 25.89062499938548356, 12.25316411605951927 ) ) ;
#22974=CARTESIAN_POINT ( 'NONE',  ( 2.000000000000003997, 25.52500000000000213, 5.535898384862238508 ) ) ;
#22975=CARTESIAN_POINT ( 'NONE',  ( 19.46311415215975771, 16.63468702741349858, 5.535898384862238508 ) ) ;
#22976=CARTESIAN_POINT ( 'NONE',  ( 19.51172774249728192, 22.34015486724339183, 5.535898384862237620 ) ) ;
#22977=LINE ( 'NONE', #24677, #2964 ) ;
#22982=CIRCLE ( 'NONE', #24, 0.5000000000000001110 ) ;
#22983=CARTESIAN_POINT ( 'NONE',  ( 16.57931677857143882, 21.89171153449011697, 11.16877607737301048 ) ) ;
#22984=CYLINDRICAL_SURFACE ( 'NONE', #19627, 4.000000000000000000 ) ;
#22987=CARTESIAN_POINT ( 'NONE',  ( -3.999999999999997335, 27.00624999877096499, 11.30940107675849404 ) ) ;
#22988=CARTESIAN_POINT ( 'NONE',  ( 3.756430356249995661, -28.92812499938548143, 6.831223922626973533 ) ) ;
#22994=CARTESIAN_POINT ( 'NONE',  ( -1.878215178125000939, -28.66562499938548569, 12.25316411605952283 ) ) ;
#22997=CARTESIAN_POINT ( 'NONE',  ( 18.35858150987925086, 23.72704589961136534, 10.28786097927511101 ) ) ;
#23005=CARTESIAN_POINT ( 'NONE',  ( 3.756430356250004099, 29.22812499938548925, 6.831223922626973533 ) ) ;
#23007=CARTESIAN_POINT ( 'NONE',  ( 21.90263254725334363, 19.07420542250708451, 12.46410161513774817 ) ) ;
#23011=CARTESIAN_POINT ( 'NONE',  ( 21.21320343559646915, 21.21320343559638744, 8.999999999999992895 ) ) ;
#23015=CARTESIAN_POINT ( 'NONE',  ( 17.29197772466794802, 18.80772725251993194, 4.999999999999994671 ) ) ;
#23016=CARTESIAN_POINT ( 'NONE',  ( 1.878215178124998497, -26.45312499938548711, 12.25316411605951927 ) ) ;
#23028=VECTOR ( 'NONE', #13580, 1000.000000000000000 ) ;
#23029=ORIENTED_EDGE ( 'NONE', *, *, #25163, .F. ) ;
#23031=VERTEX_POINT ( 'NONE', #2352 ) ;
#23035=CARTESIAN_POINT ( 'NONE',  ( -1.878215178124995832, 28.10312499938548569, 5.746835883940462963 ) ) ;
#23039=CARTESIAN_POINT ( 'NONE',  ( 21.38562447863985483, 18.72942710068040739, 5.746835883940462963 ) ) ;
#23041=CARTESIAN_POINT ( 'NONE',  ( -1.878215178124998497, 25.55312499938548854, 12.25316411605951927 ) ) ;
#23043=CARTESIAN_POINT ( 'NONE',  ( -23.36965697125209473, -11.52193136556785547, 20.00001200000000523 ) ) ;
#23051=CARTESIAN_POINT ( 'NONE',  ( -2.000000000000003997, -25.97500000000000142, 5.535898384862238508 ) ) ;
#23053=EDGE_LOOP ( 'NONE', ( #24229, #24893, #21092 ) ) ;
#23065=VERTEX_POINT ( 'NONE', #1849 ) ;
#23069=CARTESIAN_POINT ( 'NONE',  ( 3.999999999999997335, -27.51250000000000284, 11.30940107675849404 ) ) ;
#23072=CARTESIAN_POINT ( 'NONE',  ( 18.19474136253732865, 18.19474136253726471, 12.99999999999999289 ) ) ;
#23073=CARTESIAN_POINT ( 'NONE',  ( 17.90741546755112523, 20.56361284551042701, 5.746835883940462963 ) ) ;
#23074=CARTESIAN_POINT ( 'NONE',  ( 18.83113746560522728, 18.83113746560514912, 12.99999999999999112 ) ) ;
#23075=AXIS2_PLACEMENT_3D ( 'NONE', #10719, #20800, #18706 ) ;
#23076=CARTESIAN_POINT ( 'NONE',  ( 4.000000000000003553, 26.38750000000000284, 6.690598923241489970 ) ) ;
#23078=CARTESIAN_POINT ( 'NONE',  ( 19.76811771667562567, 17.11192033871618534, 12.25316411605952283 ) ) ;
#23081=VERTEX_POINT ( 'NONE', #7 ) ;
#23083=CARTESIAN_POINT ( 'NONE',  ( -1.878215178125004048, -27.46562499938548640, 5.746835883940462963 ) ) ;
#23096=CARTESIAN_POINT ( 'NONE',  ( 1.878215178124998497, -28.25312499938548427, 12.25316411605951927 ) ) ;
#23106=AXIS2_PLACEMENT_3D ( 'NONE', #6329, #12342, #12462 ) ;
#23107=CARTESIAN_POINT ( 'NONE',  ( 3.756430356250002323, 27.35312499938547859, 11.16877607737301403 ) ) ;
#23109=CARTESIAN_POINT ( 'NONE',  ( 15.03485793497900502, 20.69171218447132077, 11.30940107675849404 ) ) ;
#23110=CARTESIAN_POINT ( 'NONE',  ( 19.20899765223631306, 19.20899765223624200, 4.662447845253954171 ) ) ;
#23111=CARTESIAN_POINT ( 'NONE',  ( 19.98460540328483859, 19.98460540328476398, 4.999999999999992006 ) ) ;
#23114=CARTESIAN_POINT ( 'NONE',  ( 22.34249210749660364, 17.03009735157778337, 8.999999999999992895 ) ) ;
#23115=CARTESIAN_POINT ( 'NONE',  ( 21.64308941267829312, 20.12733988482615288, 4.999999999999997335 ) ) ;
#23118=CARTESIAN_POINT ( 'NONE',  ( -1.999999999999995781, 29.14374999877096784, 5.535898384862237620 ) ) ;
#23119=CARTESIAN_POINT ( 'NONE',  ( -3.735045420075836212E-15, -28.85312499938548569, 4.662447845253954171 ) ) ;
#23125=CARTESIAN_POINT ( 'NONE',  ( 3.756430356249997882, -28.55312499938548498, 11.16877607737301226 ) ) ;
#23126=VERTEX_POINT ( 'NONE', #16213 ) ;
#23133=( BOUNDED_CURVE ( )  B_SPLINE_CURVE ( 2, ( #2572, #8706, #494, #10396, #18652, #4798, #6491, #14739, #18394 ),
 .UNSPECIFIED., .F., .F. ) 
 B_SPLINE_CURVE_WITH_KNOTS ( ( 3, 2, 2, 2, 3 ),
 ( 0.7750000000000000222, 0.7833333333333333259, 0.8000000000000000444, 0.8166666666666666519, 0.8250000000000000666 ),
 .UNSPECIFIED. ) 
 CURVE ( )  GEOMETRIC_REPRESENTATION_ITEM ( )  RATIONAL_B_SPLINE_CURVE ( ( 0.9330127018922194093, 0.9330127018922194093, 1.000000000000000000, 0.8660254037844387076, 1.000000000000000000, 0.8660254037844387076, 1.000000000000000000, 0.9330127018922189652, 0.9330127018922194093 ) ) 
 REPRESENTATION_ITEM ( '' )  );
#23135=LINE ( 'NONE', #1423, #24320 ) ;
#23143=CARTESIAN_POINT ( 'NONE',  ( -3.063240906311874401, -29.84319947910909931, 11.57226653943512851 ) ) ;
#23144=CARTESIAN_POINT ( 'NONE',  ( -1.878215178125000939, -28.77812499938548640, 12.25316411605952283 ) ) ;
#23145=CARTESIAN_POINT ( 'NONE',  ( 18.66319960507342302, 21.49162672981954003, 12.46410161513774639 ) ) ;
#23146=LINE ( 'NONE', #22761, #23322 ) ;
#23147=CARTESIAN_POINT ( 'NONE',  ( 3.834746474454188013E-15, 25.95624999877096428, 4.999999999999992006 ) ) ;
#23148=CARTESIAN_POINT ( 'NONE',  ( 23.05168106668148553, 17.39482681718902768, 8.999999999999992895 ) ) ;
#23152=ORIENTED_EDGE ( 'NONE', *, *, #8977, .F. ) ;
#23161=EDGE_CURVE ( 'NONE', #8256, #7798, #23967, .T. ) ;
#23165=CARTESIAN_POINT ( 'NONE',  ( 3.756430356250002323, 26.11562499938548498, 11.16877607737301226 ) ) ;
#23167=CARTESIAN_POINT ( 'NONE',  ( 1.071796769724498999, 28.45134618820330275, 12.99999999999998757 ) ) ;
#23171=CARTESIAN_POINT ( 'NONE',  ( 17.51415108564528467, 23.17100533513759331, 8.999999999999992895 ) ) ;
#23172=CARTESIAN_POINT ( 'NONE',  ( 1.999999999999998224, -27.94374999877096855, 12.46410161513774639 ) ) ;
#23178=EDGE_LOOP ( 'NONE', ( #12268, #17903, #2603, #21537 ) ) ;
#23179=CARTESIAN_POINT ( 'NONE',  ( -3.469446951953614189E-15, -30.00000000000000355, 8.999999999999992895 ) ) ;
#23190=CARTESIAN_POINT ( 'NONE',  ( 21.81216202160668871, 16.49976726568787200, 6.831223922626973533 ) ) ;
#23193=CARTESIAN_POINT ( 'NONE',  ( -1.999999999999998224, 26.64999999999999858, 12.46410161513774639 ) ) ;
#23194=CARTESIAN_POINT ( 'NONE',  ( 17.27101936448323016, 19.92721674244253549, 5.746835883940462963 ) ) ;
#23196=ORIENTED_EDGE ( 'NONE', *, *, #14305, .F. ) ;
#23200=CARTESIAN_POINT ( 'NONE',  ( -3.756430356250002323, -29.60312499938548569, 11.16877607737301403 ) ) ;
#23207=DIRECTION ( 'NONE',  ( 0.000000000000000000, 0.000000000000000000, -1.000000000000000000 ) ) ;
#23210=EDGE_CURVE ( 'NONE', #24890, #19876, #22123, .T. ) ;
#23211=CARTESIAN_POINT ( 'NONE',  ( 3.756430356249996994, -28.17812499938548498, 8.999999999999992895 ) ) ;
#23220=EDGE_CURVE ( 'NONE', #24134, #18284, #1583, .T. ) ;
#23223=CARTESIAN_POINT ( 'NONE',  ( 3.756430356250003655, 26.04062499938548569, 8.999999999999992895 ) ) ;
#23224=CARTESIAN_POINT ( 'NONE',  ( -3.872397317694597163, -29.74907003676636563, 7.964378325765101962 ) ) ;
#23225=CARTESIAN_POINT ( 'NONE',  ( 19.52492222951535439, 22.18111960747465261, 12.25316411605951927 ) ) ;
#23226=CARTESIAN_POINT ( 'NONE',  ( 17.37708538166121386, 20.03328275962052274, 12.25316411605951927 ) ) ;
#23228=CARTESIAN_POINT ( 'NONE',  ( 16.21484237521500660, 21.87169662470731168, 6.690598923241487306 ) ) ;
#23230=CYLINDRICAL_SURFACE ( 'NONE', #17507, 4.000000000000000000 ) ;
#23231=CARTESIAN_POINT ( 'NONE',  ( 19.76584424242071947, 19.76584424242064486, 4.662447845253954171 ) ) ;
#23232=CARTESIAN_POINT ( 'NONE',  ( 19.94483064597403654, 19.94483064597395838, 4.999999999999992006 ) ) ;
#23235=CARTESIAN_POINT ( 'NONE',  ( 3.756430356250002323, 26.56562499938548427, 11.16877607737301226 ) ) ;
#23236=CARTESIAN_POINT ( 'NONE',  ( 3.756430356249996994, -28.96562499938548285, 8.999999999999992895 ) ) ;
#23237=CARTESIAN_POINT ( 'NONE',  ( -3.999999999999997335, 25.65624999877097068, 11.30940107675849404 ) ) ;
#23241=CARTESIAN_POINT ( 'NONE',  ( -3.735045420075836212E-15, -27.95312499938548001, 4.662447845253954171 ) ) ;
#23255=LINE ( 'NONE', #20920, #13057 ) ;
#23257=CARTESIAN_POINT ( 'NONE',  ( -25.99307600111999150, -0.5999999999999998668, 20.00001200000000168 ) ) ;
#23258=CARTESIAN_POINT ( 'NONE',  ( -2.672651547586948120E-15, -28.29062499938548569, 13.33755215474602984 ) ) ;
#23261=DIRECTION ( 'NONE',  ( 1.000000000000000000, 0.000000000000000000, 0.000000000000000000 ) ) ;
#23274=ORIENTED_EDGE ( 'NONE', *, *, #7451, .F. ) ;
#23276=( BOUNDED_CURVE ( )  B_SPLINE_CURVE ( 2, ( #15830, #23803, #11901, #7986, #2864, #22757, #24327, #10703, #6921 ),
 .UNSPECIFIED., .F., .F. ) 
 B_SPLINE_CURVE_WITH_KNOTS ( ( 3, 2, 2, 2, 3 ),
 ( 0.07500000000000001110, 0.08333333333333332871, 0.1000000000000000056, 0.1166666666666666685, 0.1250000000000000000 ),
 .UNSPECIFIED. ) 
 CURVE ( )  GEOMETRIC_REPRESENTATION_ITEM ( )  RATIONAL_B_SPLINE_CURVE ( ( 0.9330127018922192983, 0.9330127018922194093, 1.000000000000000000, 0.8660254037844387076, 1.000000000000000000, 0.8660254037844387076, 1.000000000000000000, 0.9330127018922194093, 0.9330127018922194093 ) ) 
 REPRESENTATION_ITEM ( '' )  );
#23279=( BOUNDED_CURVE ( )  B_SPLINE_CURVE ( 2, ( #9374, #11183, #17355, #23228, #25205, #7283, #15379, #21140, #15647 ),
 .UNSPECIFIED., .F., .F. ) 
 B_SPLINE_CURVE_WITH_KNOTS ( ( 3, 2, 2, 2, 3 ),
 ( 0.3250000000000000111, 0.3333333333333333148, 0.3499999999999999778, 0.3666666666666666408, 0.3750000000000000000 ),
 .UNSPECIFIED. ) 
 CURVE ( )  GEOMETRIC_REPRESENTATION_ITEM ( )  RATIONAL_B_SPLINE_CURVE ( ( 0.9330127018922194093, 0.9330127018922196314, 1.000000000000000000, 0.8660254037844387076, 1.000000000000000000, 0.8660254037844387076, 1.000000000000000000, 0.9330127018922194093, 0.9330127018922194093 ) ) 
 REPRESENTATION_ITEM ( '' )  );
#23282=CARTESIAN_POINT ( 'NONE',  ( 3.756430356250003655, 25.25312499938548427, 8.999999999999992895 ) ) ;
#23284=LINE ( 'NONE', #21465, #25149 ) ;
#23289=CARTESIAN_POINT ( 'NONE',  ( -4.000000000000001776, -27.60624999877096641, 11.30940107675849760 ) ) ;
#23290=DIRECTION ( 'NONE',  ( -0.7071067811865487940, -0.7071067811865463515, 0.000000000000000000 ) ) ;
#23295=CARTESIAN_POINT ( 'NONE',  ( -2.000000000000000888, -25.82499999999999929, 12.46410161513774817 ) ) ;
#23300=FACE_BOUND ( 'NONE', #12097, .T. ) ;
#23302=CARTESIAN_POINT ( 'NONE',  ( -3.756430356250004099, -27.09062499938548285, 6.831223922626973533 ) ) ;
#23304=CARTESIAN_POINT ( 'NONE',  ( 27.09999999999999787, -0.5999999999999998668, 19.59999999999999787 ) ) ;
#23306=ORIENTED_EDGE ( 'NONE', *, *, #24765, .F. ) ;
#23312=CARTESIAN_POINT ( 'NONE',  ( 20.75150184982686596, 15.43910709390805280, 8.999999999999992895 ) ) ;
#23314=VECTOR ( 'NONE', #5636, 1000.000000000000000 ) ;
#23315=CARTESIAN_POINT ( 'NONE',  ( 4.000000000000001776, 26.31250000000000000, 11.30940107675849760 ) ) ;
#23316=CARTESIAN_POINT ( 'NONE',  ( 19.68629472953723436, 19.68629472953716686, 13.33755215474603162 ) ) ;
#23321=CARTESIAN_POINT ( 'NONE',  ( -3.756430356250002323, -29.15312499938548640, 11.16877607737301403 ) ) ;
#23322=VECTOR ( 'NONE', #23261, 1000.000000000000000 ) ;
#23331=DIRECTION ( 'NONE',  ( 0.000000000000000000, -0.000000000000000000, -1.000000000000000000 ) ) ;
#23334=ORIENTED_EDGE ( 'NONE', *, *, #21042, .F. ) ;
#23335=CARTESIAN_POINT ( 'NONE',  ( 3.756430356249997438, -28.66562499938548569, 11.16877607737301048 ) ) ;
#23342=CARTESIAN_POINT ( 'NONE',  ( 21.21320343559646915, 21.21320343559638744, 12.99999999999999289 ) ) ;
#23346=CARTESIAN_POINT ( 'NONE',  ( 3.735045420075836212E-15, 26.15312499938548285, 4.662447845253954171 ) ) ;
#23348=CARTESIAN_POINT ( 'NONE',  ( 8.000000000000000000, 10.00000000000000000, 15.00000000000000178 ) ) ;
#23349=CARTESIAN_POINT ( 'NONE',  ( 19.41885621233737069, 22.07505359029666536, 5.746835883940462963 ) ) ;
#23350=CARTESIAN_POINT ( 'NONE',  ( 18.01348148472910893, 20.66967886268841426, 12.25316411605951927 ) ) ;
#23353=CARTESIAN_POINT ( 'NONE',  ( 22.58562062835815354, 19.74684143318851781, 5.530155478426870275 ) ) ;
#23355=CARTESIAN_POINT ( 'NONE',  ( 18.65215106205190310, 18.65215106205183915, 13.33755215474603162 ) ) ;
#23359=CARTESIAN_POINT ( 'NONE',  ( -3.756430356249997882, 25.51562499938548356, 11.16877607737301226 ) ) ;
#23360=CARTESIAN_POINT ( 'NONE',  ( -3.735045420075836212E-15, -28.40312499938548640, 4.662447845253954171 ) ) ;
#23369=CARTESIAN_POINT ( 'NONE',  ( 3.756430356249996994, -27.61562499938548143, 8.999999999999992895 ) ) ;
#23375=AXIS2_PLACEMENT_3D ( 'NONE', #3444, #25541, #1748 ) ;
#23384=( BOUNDED_CURVE ( )  B_SPLINE_CURVE ( 2, ( #14457, #17996, #4500, #2548, #10518, #24120, #8057, #18515, #602 ),
 .UNSPECIFIED., .F., .T. ) 
 B_SPLINE_CURVE_WITH_KNOTS ( ( 3, 2, 2, 2, 3 ),
 ( 0.8250000000000000666, 0.8333333333333333703, 0.8499999999999999778, 0.8666666666666666963, 0.8750000000000000000 ),
 .UNSPECIFIED. ) 
 CURVE ( )  GEOMETRIC_REPRESENTATION_ITEM ( )  RATIONAL_B_SPLINE_CURVE ( ( 0.9330127018922194093, 0.9330127018922198534, 1.000000000000000000, 0.8660254037844387076, 1.000000000000000000, 0.8660254037844387076, 1.000000000000000000, 0.9330127018922194093, 0.9330127018922194093 ) ) 
 REPRESENTATION_ITEM ( '' )  );
#23385=CARTESIAN_POINT ( 'NONE',  ( 1.859271017917182139E-15, 26.68750000000000000, 12.99999999999999289 ) ) ;
#23388=CARTESIAN_POINT ( 'NONE',  ( 19.95366948073886348, 17.12524235599260791, 12.46410161513774817 ) ) ;
#23390=CARTESIAN_POINT ( 'NONE',  ( -2.610164000359269210, -29.83019057377770622, 12.11182326528050623 ) ) ;
#23395=CARTESIAN_POINT ( 'NONE',  ( -4.000000000000003553, -28.60000000000000142, 8.999999999999992895 ) ) ;
#23412=ADVANCED_FACE ( 'NONE', ( #3238 ), #19193, .F. ) ;
#23415=CARTESIAN_POINT ( 'NONE',  ( -1.878215178124998497, 27.35312499938548569, 12.25316411605951927 ) ) ;
#23417=DIRECTION ( 'NONE',  ( 0.000000000000000000, 0.000000000000000000, -1.000000000000000000 ) ) ;
#23420=CARTESIAN_POINT ( 'NONE',  ( -5.577813053751546416E-15, -25.73124999877097352, 12.99999999999999289 ) ) ;
#23423=CARTESIAN_POINT ( 'NONE',  ( 1.999999999999998224, -26.14374999877096784, 12.46410161513774639 ) ) ;
#23436=CARTESIAN_POINT ( 'NONE',  ( 3.756430356249997882, -27.76562499938549067, 11.16877607737301226 ) ) ;
#23438=( BOUNDED_SURFACE ( )  B_SPLINE_SURFACE ( 1, 2, ( 
 ( #7815, #13702, #19721, #3900, #1550, #15796, #19838, #25860, #11871, #7564, #9901, #1430, #17887, #17763, #7948, #7427, #15935, #23907, #21678, #15415, #9518, #5987, #23388, #13466, #13972, #23521, #21433, #3514, #5472, #21941, #4020, #3763, #5605, #9401, #23644, #13584, #21552, #19578, #11986, #25611, #7695, #1819, #15676, #9783, #5721, #14482, #16065, #24535, #18160, #24290, #238, #10405, #6497, #8086, #363, #16321, #6239, #2203, #10546, #2582, #12510, #24149, #16576, #8594, #24029, #8209, #6111, #14094, #2323, #4673, #8333, #12124, #20227, #16183, #10281, #22449, #6375, #19960, #20100, #10163, #18545, #14365, #14229, #22325, #12259, #4406, #12382, #18275, #627, #2064, #22059, #22200, #4287, #20347, #20485, #6620, #14609, #116, #2444, #22590, #24420, #4529, #18404, #4146, #10032, #18030, #502, #8472, #16458, #10668, #11065, #24932, #22976, #25062, #12780, #19043, #5192, #11182, #1126, #10798, #13170 ),
 ( #2707, #21139, #3212, #7011, #18659, #4805, #19166, #8715, #24673, #9101, #8860, #6761, #14747, #16702, #1259, #25204, #14997, #20751, #12652, #8988, #18790, #16847, #877, #17090, #9243, #17232, #13042, #15259, #21021, #7282, #7151, #22725, #23226, #24810, #16965, #6889, #3098, #15141, #746, #18927, #5063, #14872, #2830, #20624, #22847, #4920, #12905, #20881, #2969, #10936, #1011, #23110, #17354, #13554, #15899, #11572, #23350, #5575, #19427, #21521, #17733, #1645, #5310, #5439, #21402, #21783, #9621, #3481, #19542, #23489, #1518, #9487, #7663, #25319, #7912, #25704, #11454, #21264, #19301, #17856, #9872, #17600, #5819, #7398, #11839, #25828, #3866, #13803, #15646, #21642, #17468, #25440, #7525, #13288, #15521, #3602, #3725, #15378, #25578, #19810, #3345, #9373, #23612, #1912, #5692, #1400, #13671, #11707, #19685, #13430, #11321, #1786, #9753, #7784, #15765, #23731, #22166, #11958, #9999, #3991, #18870 ) ),
 .UNSPECIFIED., .F., .F., .F. ) 
 B_SPLINE_SURFACE_WITH_KNOTS ( ( 2, 2 ),
 ( 3, 2, 2, 2, 2, 2, 2, 2, 2, 2, 2, 2, 2, 2, 2, 2, 2, 2, 2, 2, 2, 2, 2, 2, 2, 2, 2, 2, 2, 2, 2, 2, 2, 2, 2, 2, 2, 2, 2, 2, 2, 2, 2, 2, 2, 2, 2, 2, 2, 2, 2, 2, 2, 2, 2, 2, 2, 2, 2, 2, 3 ),
 ( 0.000000000000000000, 1.000000000000000000 ),
 ( 0.000000000000000000, 0.01666666666666666644, 0.03333333333333333287, 0.05000000000000000278, 0.06666666666666666574, 0.08333333333333332871, 0.1000000000000000056, 0.1166666666666666685, 0.1333333333333333315, 0.1499999999999999944, 0.1666666666666666574, 0.1833333333333333204, 0.2000000000000000111, 0.2166666666666666741, 0.2333333333333333370, 0.2500000000000000000, 0.2666666666666666630, 0.2833333333333333259, 0.2999999999999999889, 0.3166666666666666519, 0.3333333333333333148, 0.3499999999999999778, 0.3666666666666666408, 0.3833333333333333592, 0.4000000000000000222, 0.4166666666666666852, 0.4333333333333333481, 0.4500000000000000111, 0.4666666666666666741, 0.4833333333333333370, 0.5000000000000000000, 0.5166666666666667185, 0.5333333333333333259, 0.5500000000000000444, 0.5666666666666666519, 0.5833333333333333703, 0.5999999999999999778, 0.6166666666666666963, 0.6333333333333333037, 0.6500000000000000222, 0.6666666666666666297, 0.6833333333333333481, 0.6999999999999999556, 0.7166666666666666741, 0.7333333333333332815, 0.7500000000000000000, 0.7666666666666667185, 0.7833333333333333259, 0.8000000000000000444, 0.8166666666666666519, 0.8333333333333333703, 0.8499999999999999778, 0.8666666666666666963, 0.8833333333333333037, 0.9000000000000000222, 0.9166666666666666297, 0.9333333333333333481, 0.9499999999999999556, 0.9666666666666666741, 0.9833333333333332815, 1.000000000000000000 ),
 .UNSPECIFIED. ) 
 GEOMETRIC_REPRESENTATION_ITEM ( )  RATIONAL_B_SPLINE_SURFACE ( (
 ( 1.000000000000000000, 0.8660254037844387076, 1.000000000000000000, 0.8660254037844387076, 1.000000000000000000, 0.8660254037844387076, 1.000000000000000000, 0.8660254037844387076, 1.000000000000000000, 0.8660254037844387076, 1.000000000000000000, 0.8660254037844387076, 1.000000000000000000, 0.8660254037844387076, 1.000000000000000000, 0.8660254037844387076, 1.000000000000000000, 0.8660254037844387076, 1.000000000000000000, 0.8660254037844387076, 1.000000000000000000, 0.8660254037844387076, 1.000000000000000000, 0.8660254037844387076, 1.000000000000000000, 0.8660254037844387076, 1.000000000000000000, 0.8660254037844387076, 1.000000000000000000, 0.8660254037844387076, 1.000000000000000000, 0.8660254037844387076, 1.000000000000000000, 0.8660254037844387076, 1.000000000000000000, 0.8660254037844387076, 1.000000000000000000, 0.8660254037844387076, 1.000000000000000000, 0.8660254037844387076, 1.000000000000000000, 0.8660254037844387076, 1.000000000000000000, 0.8660254037844387076, 1.000000000000000000, 0.8660254037844387076, 1.000000000000000000, 0.8660254037844387076, 1.000000000000000000, 0.8660254037844387076, 1.000000000000000000, 0.8660254037844387076, 1.000000000000000000, 0.8660254037844387076, 1.000000000000000000, 0.8660254037844387076, 1.000000000000000000, 0.8660254037844387076, 1.000000000000000000, 0.8660254037844387076, 1.000000000000000000, 0.8660254037844387076, 1.000000000000000000, 0.8660254037844387076, 1.000000000000000000, 0.8660254037844387076, 1.000000000000000000, 0.8660254037844387076, 1.000000000000000000, 0.8660254037844387076, 1.000000000000000000, 0.8660254037844387076, 1.000000000000000000, 0.8660254037844387076, 1.000000000000000000, 0.8660254037844387076, 1.000000000000000000, 0.8660254037844387076, 1.000000000000000000, 0.8660254037844387076, 1.000000000000000000, 0.8660254037844387076, 1.000000000000000000, 0.8660254037844387076, 1.000000000000000000, 0.8660254037844387076, 1.000000000000000000, 0.8660254037844387076, 1.000000000000000000, 0.8660254037844387076, 1.000000000000000000, 0.8660254037844387076, 1.000000000000000000, 0.8660254037844387076, 1.000000000000000000, 0.8660254037844387076, 1.000000000000000000, 0.8660254037844387076, 1.000000000000000000, 0.8660254037844387076, 1.000000000000000000, 0.8660254037844387076, 1.000000000000000000, 0.8660254037844387076, 1.000000000000000000, 0.8660254037844387076, 1.000000000000000000, 0.8660254037844387076, 1.000000000000000000, 0.8660254037844387076, 1.000000000000000000, 0.8660254037844387076, 1.000000000000000000, 0.8660254037844387076, 1.000000000000000000, 0.8660254037844387076, 1.000000000000000000, 0.8660254037844387076, 1.000000000000000000, 0.8660254037844387076, 1.000000000000000000),
 ( 1.000000000000000000, 0.8660254037844387076, 1.000000000000000000, 0.8660254037844387076, 1.000000000000000000, 0.8660254037844387076, 1.000000000000000000, 0.8660254037844387076, 1.000000000000000000, 0.8660254037844387076, 1.000000000000000000, 0.8660254037844387076, 1.000000000000000000, 0.8660254037844387076, 1.000000000000000000, 0.8660254037844387076, 1.000000000000000000, 0.8660254037844387076, 1.000000000000000000, 0.8660254037844387076, 1.000000000000000000, 0.8660254037844387076, 1.000000000000000000, 0.8660254037844387076, 1.000000000000000000, 0.8660254037844387076, 1.000000000000000000, 0.8660254037844387076, 1.000000000000000000, 0.8660254037844387076, 1.000000000000000000, 0.8660254037844387076, 1.000000000000000000, 0.8660254037844387076, 1.000000000000000000, 0.8660254037844387076, 1.000000000000000000, 0.8660254037844387076, 1.000000000000000000, 0.8660254037844387076, 1.000000000000000000, 0.8660254037844387076, 1.000000000000000000, 0.8660254037844387076, 1.000000000000000000, 0.8660254037844387076, 1.000000000000000000, 0.8660254037844387076, 1.000000000000000000, 0.8660254037844387076, 1.000000000000000000, 0.8660254037844387076, 1.000000000000000000, 0.8660254037844387076, 1.000000000000000000, 0.8660254037844387076, 1.000000000000000000, 0.8660254037844387076, 1.000000000000000000, 0.8660254037844387076, 1.000000000000000000, 0.8660254037844387076, 1.000000000000000000, 0.8660254037844387076, 1.000000000000000000, 0.8660254037844387076, 1.000000000000000000, 0.8660254037844387076, 1.000000000000000000, 0.8660254037844387076, 1.000000000000000000, 0.8660254037844387076, 1.000000000000000000, 0.8660254037844387076, 1.000000000000000000, 0.8660254037844387076, 1.000000000000000000, 0.8660254037844387076, 1.000000000000000000, 0.8660254037844387076, 1.000000000000000000, 0.8660254037844387076, 1.000000000000000000, 0.8660254037844387076, 1.000000000000000000, 0.8660254037844387076, 1.000000000000000000, 0.8660254037844387076, 1.000000000000000000, 0.8660254037844387076, 1.000000000000000000, 0.8660254037844387076, 1.000000000000000000, 0.8660254037844387076, 1.000000000000000000, 0.8660254037844387076, 1.000000000000000000, 0.8660254037844387076, 1.000000000000000000, 0.8660254037844387076, 1.000000000000000000, 0.8660254037844387076, 1.000000000000000000, 0.8660254037844387076, 1.000000000000000000, 0.8660254037844387076, 1.000000000000000000, 0.8660254037844387076, 1.000000000000000000, 0.8660254037844387076, 1.000000000000000000, 0.8660254037844387076, 1.000000000000000000, 0.8660254037844387076, 1.000000000000000000, 0.8660254037844387076, 1.000000000000000000, 0.8660254037844387076, 1.000000000000000000, 0.8660254037844387076, 1.000000000000000000) ) ) 
 REPRESENTATION_ITEM ( '' )  SURFACE ( )  );
#23444=AXIS2_PLACEMENT_3D ( 'NONE', #22335, #10416, #18415 ) ;
#23446=AXIS2_PLACEMENT_3D ( 'NONE', #15030, #1425, #25343 ) ;
#23449=CARTESIAN_POINT ( 'NONE',  ( 23.08495422774248240, 17.77255947182365503, 6.831223922626973533 ) ) ;
#23451=CARTESIAN_POINT ( 'NONE',  ( 0.000000000000000000, 0.000000000000000000, 19.59999999999999787 ) ) ;
#23452=CARTESIAN_POINT ( 'NONE',  ( 4.000000000000003553, 25.44999999999999929, 8.999999999999992895 ) ) ;
#23453=CARTESIAN_POINT ( 'NONE',  ( 15.99595368409253915, 21.30834844001121553, 8.999999999999992895 ) ) ;
#23454=LINE ( 'NONE', #17828, #19159 ) ;
#23460=CARTESIAN_POINT ( 'NONE',  ( -1.878215178125000939, -29.56562499938548427, 12.25316411605952283 ) ) ;
#23463=CARTESIAN_POINT ( 'NONE',  ( 4.000000000000003553, 26.38750000000000284, 6.690598923241489970 ) ) ;
#23465=CARTESIAN_POINT ( 'NONE',  ( -3.834746474454188013E-15, -26.40624999877096357, 4.999999999999992006 ) ) ;
#23467=VERTEX_POINT ( 'NONE', #15546 ) ;
#23470=VERTEX_POINT ( 'NONE', #5601 ) ;
#23476=CARTESIAN_POINT ( 'NONE',  ( -2.000000000000000888, -26.21874999877096712, 12.46410161513774817 ) ) ;
#23478=VECTOR ( 'NONE', #2317, 1000.000000000000000 ) ;
#23481=CARTESIAN_POINT ( 'NONE',  ( -1.878215178124998497, 29.04062499938548569, 12.25316411605951927 ) ) ;
#23482=DIRECTION ( 'NONE',  ( -0.7071067811865487940, -0.7071067811865463515, 0.000000000000000000 ) ) ;
#23486=CARTESIAN_POINT ( 'NONE',  ( 2.672651547586948120E-15, 26.82812499938548356, 13.33755215474603162 ) ) ;
#23488=CARTESIAN_POINT ( 'NONE',  ( 20.94803839265150458, 18.11961126790524901, 12.46410161513774817 ) ) ;
#23489=CARTESIAN_POINT ( 'NONE',  ( 19.68629472953723436, 19.68629472953716686, 13.33755215474602984 ) ) ;
#23492=FACE_OUTER_BOUND ( 'NONE', #10298, .T. ) ;
#23493=CARTESIAN_POINT ( 'NONE',  ( 20.78451994863305430, 15.12766569914060888, 8.999999999999992895 ) ) ;
#23496=CARTESIAN_POINT ( 'NONE',  ( -4.000000000000003553, -26.80000000000000071, 8.999999999999992895 ) ) ;
#23500=VECTOR ( 'NONE', #15982, 1000.000000000000000 ) ;
#23502=CARTESIAN_POINT ( 'NONE',  ( -25.83240171513484640, 3.403349963601426165, 20.00001199999999812 ) ) ;
#23503=CARTESIAN_POINT ( 'NONE',  ( 1.071796769724494558, 26.38615380933864074, 4.999999999999992895 ) ) ;
#23514=CARTESIAN_POINT ( 'NONE',  ( 1.999999999999998224, -27.49374999877096926, 12.46410161513774639 ) ) ;
#23516=DIRECTION ( 'NONE',  ( 0.000000000000000000, 0.000000000000000000, -1.000000000000000000 ) ) ;
#23521=CARTESIAN_POINT ( 'NONE',  ( 21.44743255599544440, 15.79057830650299721, 6.690598923241489970 ) ) ;
#23526=CARTESIAN_POINT ( 'NONE',  ( 8.831537335106614961E-15, 26.63124999877096855, 12.99999999999999112 ) ) ;
#23527=CARTESIAN_POINT ( 'NONE',  ( 2.000000000000003997, 27.32500000000000284, 5.535898384862238508 ) ) ;
#23530=CARTESIAN_POINT ( 'NONE',  ( 1.071796769724490117, -26.87634618820330701, 4.999999999999992895 ) ) ;
#23534=VERTEX_POINT ( 'NONE', #5716 ) ;
#23536=VERTEX_POINT ( 'NONE', #11865 ) ;
#23541=CARTESIAN_POINT ( 'NONE',  ( -1.071796769724494558, -28.18615380933863435, 4.999999999999992895 ) ) ;
#23549=CARTESIAN_POINT ( 'NONE',  ( 3.756430356250002323, 28.36562499938548854, 11.16877607737301226 ) ) ;
#23558=CARTESIAN_POINT ( 'NONE',  ( -2.620986760973688460E-15, -26.63124999877097565, 13.61880215351699874 ) ) ;
#23559=CARTESIAN_POINT ( 'NONE',  ( -3.756430356249995661, 27.69062499938548427, 6.831223922626973533 ) ) ;
#23564=EDGE_CURVE ( 'NONE', #13049, #10227, #10734, .T. ) ;
#23569=DIRECTION ( 'NONE',  ( 1.000000000000000000, 0.000000000000000000, 0.000000000000000000 ) ) ;
#23572=CARTESIAN_POINT ( 'NONE',  ( 3.756430356249995661, -28.14062499938548356, 6.831223922626973533 ) ) ;
#23573=VERTEX_POINT ( 'NONE', #2318 ) ;
#23575=ORIENTED_EDGE ( 'NONE', *, *, #14777, .T. ) ;
#23579=CARTESIAN_POINT ( 'NONE',  ( 20.45982030258741702, 15.14742554666860208, 6.831223922626973533 ) ) ;
#23580=FACE_OUTER_BOUND ( 'NONE', #22502, .T. ) ;
#23582=CARTESIAN_POINT ( 'NONE',  ( -3.999999999999997335, 27.96250000000000213, 11.30940107675849404 ) ) ;
#23584=CARTESIAN_POINT ( 'NONE',  ( 23.05843772344798381, 17.74604296752915999, 8.999999999999992895 ) ) ;
#23588=ORIENTED_EDGE ( 'NONE', *, *, #20808, .T. ) ;
#23601=CARTESIAN_POINT ( 'NONE',  ( 3.469446951953614189E-15, 30.00000000000000355, 4.999999999999992006 ) ) ;
#23606=CARTESIAN_POINT ( 'NONE',  ( 3.756430356250004099, 26.07812499938548356, 6.831223922626973533 ) ) ;
#23611=CARTESIAN_POINT ( 'NONE',  ( 21.46069080901174786, 15.80383655951930066, 8.999999999999992895 ) ) ;
#23612=CARTESIAN_POINT ( 'NONE',  ( 17.90514199329621903, 23.21753674921489008, 8.999999999999992895 ) ) ;
#23614=CARTESIAN_POINT ( 'NONE',  ( -1.071796769724494558, -28.63615380933863364, 4.999999999999992895 ) ) ;
#23616=FACE_OUTER_BOUND ( 'NONE', #10387, .T. ) ;
#23617=ADVANCED_FACE ( 'NONE', ( #111 ), #24025, .F. ) ;
#23622=CARTESIAN_POINT ( 'NONE',  ( -2.000000000000003997, -26.42500000000000071, 5.535898384862238508 ) ) ;
#23638=CARTESIAN_POINT ( 'NONE',  ( -3.834746474454188013E-15, -27.36250000000000426, 4.999999999999992006 ) ) ;
#23639=CARTESIAN_POINT ( 'NONE',  ( 19.29959570814131808, 22.12802283288743155, 12.46410161513774639 ) ) ;
#23644=CARTESIAN_POINT ( 'NONE',  ( 20.27186753227280747, 17.44344040752655545, 12.46410161513774817 ) ) ;
#23646=DIRECTION ( 'NONE',  ( -0.000000000000000000, -0.000000000000000000, -1.000000000000000000 ) ) ;
#23649=CARTESIAN_POINT ( 'NONE',  ( 18.39361514561510091, 18.39361514561503341, 4.999999999999992006 ) ) ;
#23655=CARTESIAN_POINT ( 'NONE',  ( -2.000000000000003997, -26.42500000000000071, 5.535898384862238508 ) ) ;
#23665=CARTESIAN_POINT ( 'NONE',  ( 23.26836714124207361, 18.93629030671969460, 11.57226653943513028 ) ) ;
#23669=CARTESIAN_POINT ( 'NONE',  ( 3.735045420075836212E-15, 27.16562499938548569, 4.662447845253954171 ) ) ;
#23676=CARTESIAN_POINT ( 'NONE',  ( 1.999999999999998224, -25.69374999877097210, 12.46410161513774639 ) ) ;
#23677=CARTESIAN_POINT ( 'NONE',  ( 3.756430356250003655, 28.85312499938548569, 8.999999999999992895 ) ) ;
#23682=EDGE_LOOP ( 'NONE', ( #8225, #19216 ) ) ;
#23686=CARTESIAN_POINT ( 'NONE',  ( -1.878215178125000939, -26.97812499938548569, 12.25316411605952283 ) ) ;
#23687=ORIENTED_EDGE ( 'NONE', *, *, #14503, .T. ) ;
#23688=CARTESIAN_POINT ( 'NONE',  ( -3.834746474454188013E-15, -26.01249999999999574, 4.999999999999992006 ) ) ;
#23696=CARTESIAN_POINT ( 'NONE',  ( 15.30652457243565223, 20.61891932835433394, 11.16877607737301226 ) ) ;
#23700=CARTESIAN_POINT ( 'NONE',  ( 2.620986760973688460E-15, 28.93750000000000000, 13.61880215351699874 ) ) ;
#23702=CARTESIAN_POINT ( 'NONE',  ( 18.96807563933094798, 21.62427301729024975, 12.25316411605951927 ) ) ;
#23711=VERTEX_POINT ( 'NONE', #24416 ) ;
#23724=CARTESIAN_POINT ( 'NONE',  ( -1.878215178124998497, 25.89062499938548356, 12.25316411605951927 ) ) ;
#23726=LINE ( 'NONE', #80, #11735 ) ;
#23730=CARTESIAN_POINT ( 'NONE',  ( 18.38477631085027753, 21.21320343559639454, 12.46410161513774639 ) ) ;
#23731=CARTESIAN_POINT ( 'NONE',  ( 18.24985654912466515, 23.56225130504333976, 11.16877607737301226 ) ) ;
#23732=DIRECTION ( 'NONE',  ( 0.000000000000000000, 0.000000000000000000, 1.000000000000000000 ) ) ;
#23741=CARTESIAN_POINT ( 'NONE',  ( -2.620986760973688460E-15, -26.23750000000000071, 13.61880215351699874 ) ) ;
#23743=EDGE_LOOP ( 'NONE', ( #14831, #13119, #13054, #6032, #12179, #9381, #9560, #640, #1029, #17658, #6604, #24521, #24078, #20534, #20009, #794, #15658, #551, #7447, #7380, #15881, #22254, #21527, #213, #20825 ) ) ;
#23745=CARTESIAN_POINT ( 'NONE',  ( 1.057460391440397258E-14, -29.55624999877096926, 4.999999999999992006 ) ) ;
#23746=CARTESIAN_POINT ( 'NONE',  ( 1.701696020694463574, 25.99999999999999645, 20.00001200000000168 ) ) ;
#23757=EDGE_CURVE ( 'NONE', #5938, #3647, #18655, .T. ) ;
#23763=CARTESIAN_POINT ( 'NONE',  ( 3.834746474454188013E-15, 27.36250000000000071, 4.999999999999992006 ) ) ;
#23778=CARTESIAN_POINT ( 'NONE',  ( 1.999999999999998224, -26.59374999877096712, 12.46410161513774639 ) ) ;
#23795=CARTESIAN_POINT ( 'NONE',  ( 3.756430356250004099, 28.44062499938548783, 6.831223922626973533 ) ) ;
#23797=EDGE_CURVE ( 'NONE', #19408, #4579, #8467, .T. ) ;
#23803=CARTESIAN_POINT ( 'NONE',  ( 1.071796769724494336, 25.75134618820330346, 12.99999999999999467 ) ) ;
#23805=CARTESIAN_POINT ( 'NONE',  ( 3.999999999999996447, -28.31874999877096855, 8.999999999999992895 ) ) ;
#23806=CARTESIAN_POINT ( 'NONE',  ( 1.878215178125000939, 28.77812499938548640, 12.25316411605952283 ) ) ;
#23807=CARTESIAN_POINT ( 'NONE',  ( -3.834746474454188013E-15, -26.01249999999999574, 4.999999999999992006 ) ) ;
#23809=DIRECTION ( 'NONE',  ( 0.000000000000000000, -1.000000000000000000, 0.000000000000000000 ) ) ;
#23810=CARTESIAN_POINT ( 'NONE',  ( -1.859271017917182139E-15, -26.18124999877096570, 12.99999999999999289 ) ) ;
#23812=CARTESIAN_POINT ( 'NONE',  ( -4.000000000000003553, -29.08750000000000213, 6.690598923241489970 ) ) ;
#23813=EDGE_LOOP ( 'NONE', ( #15598, #15390, #4060, #17305, #8376 ) ) ;
#23816=EDGE_LOOP ( 'NONE', ( #19059, #11016, #14164 ) ) ;
#23819=CARTESIAN_POINT ( 'NONE',  ( -1.878215178125004048, -27.57812499938548711, 5.746835883940462963 ) ) ;
#23825=CARTESIAN_POINT ( 'NONE',  ( 2.000000000000000888, 29.81874999877096855, 12.46410161513774817 ) ) ;
#23826=CARTESIAN_POINT ( 'NONE',  ( 1.878215178125004048, 26.67812499938548498, 5.746835883940462963 ) ) ;
#23828=CYLINDRICAL_SURFACE ( 'NONE', #18354, 4.000000000000000000 ) ;
#23829=CARTESIAN_POINT ( 'NONE',  ( 22.71372316761954124, 17.40132841170072808, 11.16877607737301226 ) ) ;
#23834=CARTESIAN_POINT ( 'NONE',  ( -3.999999999999996003, 29.23750000000000071, 6.690598923241487306 ) ) ;
#23842=ORIENTED_EDGE ( 'NONE', *, *, #6754, .F. ) ;
#23848=CARTESIAN_POINT ( 'NONE',  ( 3.756430356250004099, 26.64062499938549067, 6.831223922626973533 ) ) ;
#23849=CARTESIAN_POINT ( 'NONE',  ( 18.35384038830430597, 18.35384038830423492, 4.999999999999992006 ) ) ;
#23851=EDGE_CURVE ( 'NONE', #446, #2329, #16454, .T. ) ;
#23856=CARTESIAN_POINT ( 'NONE',  ( 3.999999999999996447, -25.67500000000000071, 8.999999999999992895 ) ) ;
#23862=CARTESIAN_POINT ( 'NONE',  ( 3.137519842735244810E-15, -26.91249999999999787, 4.999999999999991118 ) ) ;
#23866=CARTESIAN_POINT ( 'NONE',  ( -1.878215178124995832, 25.29062499938548569, 5.746835883940462963 ) ) ;
#23871=CARTESIAN_POINT ( 'NONE',  ( 18.06657825931632999, 20.89500538406245056, 12.46410161513774639 ) ) ;
#23874=EDGE_CURVE ( 'NONE', #3881, #22864, #21516, .T. ) ;
#23878=CARTESIAN_POINT ( 'NONE',  ( 22.02202058170775345, 19.36582320374829891, 5.746835883940462963 ) ) ;
#23881=CARTESIAN_POINT ( 'NONE',  ( -2.000000000000003997, -26.87500000000000355, 5.535898384862238508 ) ) ;
#23882=EDGE_CURVE ( 'NONE', #20963, #8492, #25198, .T. ) ;
#23892=ORIENTED_EDGE ( 'NONE', *, *, #15880, .F. ) ;
#23906=CARTESIAN_POINT ( 'NONE',  ( 19.15823811790222919, 16.50204073994278531, 5.746835883940462963 ) ) ;
#23907=CARTESIAN_POINT ( 'NONE',  ( 15.57844627214710975, 21.23530052163942372, 6.690598923241487306 ) ) ;
#23910=CARTESIAN_POINT ( 'NONE',  ( 2.645323980344223447, 29.88371542788442881, 5.988343842124890237 ) ) ;
#23913=CARTESIAN_POINT ( 'NONE',  ( -1.999999999999995781, 26.44374999877096855, 5.535898384862237620 ) ) ;
#23917=CARTESIAN_POINT ( 'NONE',  ( 4.000000000000003553, 25.43124999877096926, 6.690598923241489970 ) ) ;
#23920=ORIENTED_EDGE ( 'NONE', *, *, #14777, .F. ) ;
#23921=EDGE_CURVE ( 'NONE', #8698, #4544, #17463, .T. ) ;
#23927=AXIS2_PLACEMENT_3D ( 'NONE', #9803, #6008, #17782 ) ;
#23933=CARTESIAN_POINT ( 'NONE',  ( 3.735045420075836212E-15, 27.61562499938548498, 4.662447845253954171 ) ) ;
#23938=FACE_OUTER_BOUND ( 'NONE', #24345, .T. ) ;
#23941=CARTESIAN_POINT ( 'NONE',  ( -2.000000000000003997, -29.06874999877096855, 5.535898384862238508 ) ) ;
#23942=CARTESIAN_POINT ( 'NONE',  ( -1.878215178124995832, 28.10312499938548569, 5.746835883940462963 ) ) ;
#23944=MECHANICAL_DESIGN_GEOMETRIC_PRESENTATION_REPRESENTATION('',(#8495),#1396);
#23949=CARTESIAN_POINT ( 'NONE',  ( 1.878215178124998497, -29.49062499938548498, 12.25316411605951927 ) ) ;
#23953=VERTEX_POINT ( 'NONE', #5306 ) ;
#23954=CARTESIAN_POINT ( 'NONE',  ( 17.39040739893763643, 20.21883452368375700, 12.46410161513774639 ) ) ;
#23958=CARTESIAN_POINT ( 'NONE',  ( 20.59759129326749871, 19.08184176541537624, 12.99999999999998757 ) ) ;
#23962=CARTESIAN_POINT ( 'NONE',  ( -3.756430356249996105, 26.79062499938548569, 6.831223922626973533 ) ) ;
#23966=CARTESIAN_POINT ( 'NONE',  ( 19.76584424242071947, 19.76584424242064486, 4.662447845253954171 ) ) ;
#23967=( BOUNDED_CURVE ( )  B_SPLINE_CURVE ( 2, ( #1965, #9929, #2095, #20779, #912, #2736, #22480, #10575, #18573 ),
 .UNSPECIFIED., .F., .F. ) 
 B_SPLINE_CURVE_WITH_KNOTS ( ( 3, 2, 2, 2, 3 ),
 ( 0.6250000000000000000, 0.6333333333333333037, 0.6500000000000000222, 0.6666666666666666297, 0.6750000000000000444 ),
 .UNSPECIFIED. ) 
 CURVE ( )  GEOMETRIC_REPRESENTATION_ITEM ( )  RATIONAL_B_SPLINE_CURVE ( ( 0.9330127018922194093, 0.9330127018922194093, 1.000000000000000000, 0.8660254037844387076, 1.000000000000000000, 0.8660254037844387076, 1.000000000000000000, 0.9330127018922189652, 0.9330127018922194093 ) ) 
 REPRESENTATION_ITEM ( '' )  );
#23970=CARTESIAN_POINT ( 'NONE',  ( 4.000000000000003553, 28.60000000000000142, 8.999999999999992895 ) ) ;
#23971=( BOUNDED_CURVE ( )  B_SPLINE_CURVE ( 2, ( #19457, #15287, #13197, #1817, #21550, #19719, #17263, #7425, #21431 ),
 .UNSPECIFIED., .F., .F. ) 
 B_SPLINE_CURVE_WITH_KNOTS ( ( 3, 2, 2, 2, 3 ),
 ( 0.3250000000000000111, 0.3333333333333333148, 0.3499999999999999778, 0.3666666666666666408, 0.3750000000000000000 ),
 .UNSPECIFIED. ) 
 CURVE ( )  GEOMETRIC_REPRESENTATION_ITEM ( )  RATIONAL_B_SPLINE_CURVE ( ( 0.9330127018922194093, 0.9330127018922196314, 1.000000000000000000, 0.8660254037844387076, 1.000000000000000000, 0.8660254037844387076, 1.000000000000000000, 0.9330127018922194093, 0.9330127018922194093 ) ) 
 REPRESENTATION_ITEM ( '' )  );
#23980=DIRECTION ( 'NONE',  ( 0.000000000000000000, 0.000000000000000000, -1.000000000000000000 ) ) ;
#23981=CARTESIAN_POINT ( 'NONE',  ( -3.756430356249995661, 25.44062499938548427, 6.831223922626973533 ) ) ;
#23984=CARTESIAN_POINT ( 'NONE',  ( 3.999999999999997335, -25.71249999999999503, 11.30940107675849404 ) ) ;
#23993=AXIS2_PLACEMENT_3D ( 'NONE', #7786, #15649, #15380 ) ;
#23994=CARTESIAN_POINT ( 'NONE',  ( 1.878215178125004048, 25.21562499938548285, 5.746835883940462963 ) ) ;
#23997=CARTESIAN_POINT ( 'NONE',  ( 18.99023649137219039, 18.99023649137212999, 4.999999999999991118 ) ) ;
#23998=CARTESIAN_POINT ( 'NONE',  ( 16.62584819264874270, 22.28270244214105134, 11.30940107675849404 ) ) ;
#24003=CARTESIAN_POINT ( 'NONE',  ( 20.24314131972164077, 20.24314131972156972, 13.33755215474603162 ) ) ;
#24007=CARTESIAN_POINT ( 'NONE',  ( 1.999999999999995781, -27.85000000000000142, 5.535898384862237620 ) ) ;
#24024=CARTESIAN_POINT ( 'NONE',  ( 0.000000000000000000, 0.000000000000000000, 20.00000000000000000 ) ) ;
#24025=CYLINDRICAL_SURFACE ( 'NONE', #17191, 4.000000000000000000 ) ;
#24029=CARTESIAN_POINT ( 'NONE',  ( 18.23893553636149534, 21.06736266110760880, 5.535898384862237620 ) ) ;
#24031=DIRECTION ( 'NONE',  ( 0.000000000000000000, 0.000000000000000000, -1.000000000000000000 ) ) ;
#24032=CARTESIAN_POINT ( 'NONE',  ( 3.795382382264993915, 29.75912104221810495, 7.710170883190207824 ) ) ;
#24034=CARTESIAN_POINT ( 'NONE',  ( 3.959305739469038251E-15, 30.00000000000000355, 12.99999999999999289 ) ) ;
#24040=CARTESIAN_POINT ( 'NONE',  ( 3.752267015613588906E-15, 25.50624999877097565, 4.381197846482986158 ) ) ;
#24042=DIRECTION ( 'NONE',  ( 0.000000000000000000, 0.000000000000000000, -1.000000000000000000 ) ) ;
#24054=CARTESIAN_POINT ( 'NONE',  ( 3.756430356250003655, 25.14062499938548356, 8.999999999999992895 ) ) ;
#24059=CYLINDRICAL_SURFACE ( 'NONE', #25089, 4.000000000000000000 ) ;
#24060=CARTESIAN_POINT ( 'NONE',  ( 3.999999999999996447, -25.61874999877096926, 8.999999999999992895 ) ) ;
#24062=CARTESIAN_POINT ( 'NONE',  ( -3.756430356250003655, -25.25312499938548427, 8.999999999999992895 ) ) ;
#24063=ADVANCED_FACE ( 'NONE', ( #24928 ), #13038, .F. ) ;
#24064=CARTESIAN_POINT ( 'NONE',  ( 1.878215178125004048, 28.47812499938548569, 5.746835883940462963 ) ) ;
#24065=CARTESIAN_POINT ( 'NONE',  ( 1.999999999999998224, -26.20000000000000284, 12.46410161513774639 ) ) ;
#24066=CARTESIAN_POINT ( 'NONE',  ( 1.859271017917182139E-15, 29.78124999877096712, 12.99999999999999289 ) ) ;
#24068=ORIENTED_EDGE ( 'NONE', *, *, #16370, .T. ) ;
#24070=CARTESIAN_POINT ( 'NONE',  ( -3.756430356250003655, -29.64062499938548356, 8.999999999999992895 ) ) ;
#24073=EDGE_CURVE ( 'NONE', #20170, #23534, #23726, .T. ) ;
#24078=ORIENTED_EDGE ( 'NONE', *, *, #2001, .T. ) ;
#24080=CARTESIAN_POINT ( 'NONE',  ( -1.878215178124995832, 27.20312499938548711, 5.746835883940462963 ) ) ;
#24084=CARTESIAN_POINT ( 'NONE',  ( 21.41441445718925962, 16.10201970127043936, 6.831223922626973533 ) ) ;
#24089=CARTESIAN_POINT ( 'NONE',  ( 2.000000000000000888, 27.17500000000000071, 12.46410161513774817 ) ) ;
#24090=CARTESIAN_POINT ( 'NONE',  ( -3.756430356249997438, 29.00312499938548072, 11.16877607737301048 ) ) ;
#24092=DIRECTION ( 'NONE',  ( 0.000000000000000000, 0.000000000000000000, -1.000000000000000000 ) ) ;
#24100=CARTESIAN_POINT ( 'NONE',  ( 3.756430356250003655, 25.25312499938548427, 8.999999999999992895 ) ) ;
#24103=EDGE_LOOP ( 'NONE', ( #12879, #15983, #12788, #18803 ) ) ;
#24105=ORIENTED_EDGE ( 'NONE', *, *, #8699, .T. ) ;
#24110=CARTESIAN_POINT ( 'NONE',  ( -2.000000000000000888, -26.72500000000000142, 12.46410161513774817 ) ) ;
#24114=CARTESIAN_POINT ( 'NONE',  ( 1.878215178125004048, 26.56562499938548427, 5.746835883940462963 ) ) ;
#24119=CARTESIAN_POINT ( 'NONE',  ( 3.878215178125003604, 25.07031249969274356, 8.999999999999992895 ) ) ;
#24120=CARTESIAN_POINT ( 'NONE',  ( -3.999999999999997335, 29.25624999877096855, 11.30940107675849404 ) ) ;
#24122=VECTOR ( 'NONE', #19398, 1000.000000000000000 ) ;
#24126=CARTESIAN_POINT ( 'NONE',  ( -2.620986760973688460E-15, -29.38749999999999929, 13.61880215351699874 ) ) ;
#24134=VERTEX_POINT ( 'NONE', #13800 ) ;
#24135=CARTESIAN_POINT ( 'NONE',  ( -3.735045420075836212E-15, -25.36562499938548854, 4.662447845253954171 ) ) ;
#24139=VECTOR ( 'NONE', #278, 1000.000000000000000 ) ;
#24142=CARTESIAN_POINT ( 'NONE',  ( 17.85886564147372724, 23.51571989096603588, 11.30940107675849404 ) ) ;
#24145=CIRCLE ( 'NONE', #9965, 26.00000000000000355 ) ;
#24147=DIRECTION ( 'NONE',  ( -0.7071067811865487940, -0.7071067811865463515, 0.000000000000000000 ) ) ;
#24148=CARTESIAN_POINT ( 'NONE',  ( 17.50966790313369259, 20.16586528109299437, 5.746835883940462963 ) ) ;
#24149=CARTESIAN_POINT ( 'NONE',  ( 22.40202671059728345, 16.74517246110483271, 6.690598923241489970 ) ) ;
#24158=LINE ( 'NONE', #16583, #25500 ) ;
#24160=CARTESIAN_POINT ( 'NONE',  ( -3.834746474454188013E-15, -28.26249999999999929, 4.999999999999992006 ) ) ;
#24161=CARTESIAN_POINT ( 'NONE',  ( 3.752267015613588906E-15, 25.95624999877096784, 4.381197846482986158 ) ) ;
#24162=CARTESIAN_POINT ( 'NONE',  ( 3.756430356249997882, -27.20312499938548001, 11.16877607737301226 ) ) ;
#24165=EDGE_CURVE ( 'NONE', #20732, #8492, #4400, .T. ) ;
#24166=AXIS2_PLACEMENT_3D ( 'NONE', #7569, #17387, #1555 ) ;
#24170=ADVANCED_FACE ( 'NONE', ( #21638 ), #17853, .F. ) ;
#24181=CARTESIAN_POINT ( 'NONE',  ( -1.878215178124998497, 26.79062499938548214, 12.25316411605951927 ) ) ;
#24188=CARTESIAN_POINT ( 'NONE',  ( 15.35305598651295256, 21.00991023600527186, 11.30940107675849404 ) ) ;
#24189=CARTESIAN_POINT ( 'NONE',  ( 3.756430356249995661, -25.44062499938548427, 6.831223922626973533 ) ) ;
#24191=LINE ( 'NONE', #542, #4518 ) ;
#24197=DIRECTION ( 'NONE',  ( 0.000000000000000000, 0.000000000000000000, -1.000000000000000000 ) ) ;
#24199=ORIENTED_EDGE ( 'NONE', *, *, #18631, .T. ) ;
#24206=VECTOR ( 'NONE', #23482, 1000.000000000000000 ) ;
#24211=CARTESIAN_POINT ( 'NONE',  ( 1.878215178125004048, 25.32812499938548356, 5.746835883940462963 ) ) ;
#24212=AXIS2_PLACEMENT_3D ( 'NONE', #22378, #10725, #12437 ) ;
#24215=DIRECTION ( 'NONE',  ( 0.000000000000000000, -1.000000000000000000, 0.000000000000000000 ) ) ;
#24216=CARTESIAN_POINT ( 'NONE',  ( 20.00676625532608455, 17.35056887736664422, 12.25316411605952283 ) ) ;
#24221=CARTESIAN_POINT ( 'NONE',  ( 4.000000000000001776, 29.46250000000000568, 11.30940107675849760 ) ) ;
#24222=CARTESIAN_POINT ( 'NONE',  ( -1.878215178124998497, 29.49062499938548498, 12.25316411605951927 ) ) ;
#24225=CARTESIAN_POINT ( 'NONE',  ( -1.071796769724487230, 27.38259618943233420, 4.999999999999992006 ) ) ;
#24227=( BOUNDED_CURVE ( )  B_SPLINE_CURVE ( 2, ( #7269, #2955, #21007, #12767, #14859, #1113, #14982, #2696, #15247 ),
 .UNSPECIFIED., .F., .F. ) 
 B_SPLINE_CURVE_WITH_KNOTS ( ( 3, 2, 2, 2, 3 ),
 ( 0.1749999999999999889, 0.1833333333333333204, 0.2000000000000000111, 0.2166666666666666741, 0.2250000000000000056 ),
 .UNSPECIFIED. ) 
 CURVE ( )  GEOMETRIC_REPRESENTATION_ITEM ( )  RATIONAL_B_SPLINE_CURVE ( ( 0.9330127018922194093, 0.9330127018922194093, 1.000000000000000000, 0.8660254037844387076, 1.000000000000000000, 0.8660254037844387076, 1.000000000000000000, 0.9330127018922194093, 0.9330127018922194093 ) ) 
 REPRESENTATION_ITEM ( '' )  );
#24228=ORIENTED_EDGE ( 'NONE', *, *, #14650, .T. ) ;
#24229=ORIENTED_EDGE ( 'NONE', *, *, #2035, .T. ) ;
#24235=ORIENTED_EDGE ( 'NONE', *, *, #25005, .T. ) ;
#24240=ORIENTED_EDGE ( 'NONE', *, *, #24489, .T. ) ;
#24245=VECTOR ( 'NONE', #8342, 1000.000000000000227 ) ;
#24247=CARTESIAN_POINT ( 'NONE',  ( 2.000000000000000888, 29.36874999877096926, 12.46410161513774817 ) ) ;
#24250=CARTESIAN_POINT ( 'NONE',  ( -1.878215178124995832, 27.09062499938548640, 5.746835883940462963 ) ) ;
#24252=AXIS2_PLACEMENT_3D ( 'NONE', #15322, #23290, #8936 ) ;
#24253=CARTESIAN_POINT ( 'NONE',  ( 17.87212389449003425, 23.52897814398233933, 8.999999999999992895 ) ) ;
#24256=DIRECTION ( 'NONE',  ( -1.000000000000000000, 0.000000000000000000, 0.000000000000000000 ) ) ;
#24257=CARTESIAN_POINT ( 'NONE',  ( -3.756430356250003655, -25.14062499938548356, 8.999999999999992895 ) ) ;
#24259=CARTESIAN_POINT ( 'NONE',  ( 17.75721904254721295, 17.75721904254714545, 4.999999999999992006 ) ) ;
#24262=CARTESIAN_POINT ( 'NONE',  ( -4.000000000000003553, -28.63750000000000284, 6.690598923241489970 ) ) ;
#24273=CARTESIAN_POINT ( 'NONE',  ( 3.756430356249997438, -27.31562499938548427, 11.16877607737301048 ) ) ;
#24275=( BOUNDED_CURVE ( )  B_SPLINE_CURVE ( 2, ( #22209, #20235, #12661, #10414, #2331, #18413, #14374, #10291, #371 ),
 .UNSPECIFIED., .F., .F. ) 
 B_SPLINE_CURVE_WITH_KNOTS ( ( 3, 2, 2, 2, 3 ),
 ( 0.6250000000000000000, 0.6333333333333333037, 0.6500000000000000222, 0.6666666666666666297, 0.6750000000000000444 ),
 .UNSPECIFIED. ) 
 CURVE ( )  GEOMETRIC_REPRESENTATION_ITEM ( )  RATIONAL_B_SPLINE_CURVE ( ( 0.9330127018922194093, 0.9330127018922194093, 1.000000000000000000, 0.8660254037844387076, 1.000000000000000000, 0.8660254037844387076, 1.000000000000000000, 0.9330127018922189652, 0.9330127018922194093 ) ) 
 REPRESENTATION_ITEM ( '' )  );
#24278=VECTOR ( 'NONE', #3713, 1000.000000000000000 ) ;
#24280=AXIS2_PLACEMENT_3D ( 'NONE', #21910, #23732, #3992 ) ;
#24287=CARTESIAN_POINT ( 'NONE',  ( 20.09187391231935393, 18.57612438446723857, 4.999999999999992895 ) ) ;
#24289=CARTESIAN_POINT ( 'NONE',  ( 19.79463422097012426, 17.13843684301067682, 5.746835883940462963 ) ) ;
#24290=CARTESIAN_POINT ( 'NONE',  ( 22.08382865906333947, 16.42697440957088872, 6.690598923241489970 ) ) ;
#24295=LINE ( 'NONE', #506, #10786 ) ;
#24300=FACE_OUTER_BOUND ( 'NONE', #20702, .T. ) ;
#24301=FACE_OUTER_BOUND ( 'NONE', #12426, .T. ) ;
#24302=CARTESIAN_POINT ( 'NONE',  ( -3.756430356250003655, -27.39062499938548356, 8.999999999999992895 ) ) ;
#24304=EDGE_LOOP ( 'NONE', ( #12519, #22463, #22307, #25142 ) ) ;
#24307=ORIENTED_EDGE ( 'NONE', *, *, #24390, .T. ) ;
#24308=CARTESIAN_POINT ( 'NONE',  ( -3.756430356250004099, -25.17812499938548498, 6.831223922626973533 ) ) ;
#24309=ORIENTED_EDGE ( 'NONE', *, *, #4746, .T. ) ;
#24320=VECTOR ( 'NONE', #5465, 1000.000000000000000 ) ;
#24321=CARTESIAN_POINT ( 'NONE',  ( 3.756430356250004099, 26.07812499938548356, 6.831223922626973533 ) ) ;
#24326=FACE_OUTER_BOUND ( 'NONE', #12761, .T. ) ;
#24327=CARTESIAN_POINT ( 'NONE',  ( 2.000000000000003997, 25.91874999877096997, 5.535898384862238508 ) ) ;
#24330=CARTESIAN_POINT ( 'NONE',  ( -4.000000000000003553, -28.13124999877096855, 6.690598923241489970 ) ) ;
#24343=EDGE_CURVE ( 'NONE', #18977, #1175, #7769, .T. ) ;
#24345=EDGE_LOOP ( 'NONE', ( #7257, #18728, #9676, #11619 ) ) ;
#24349=CARTESIAN_POINT ( 'NONE',  ( -1.878215178124998497, 25.55312499938548854, 12.25316411605951927 ) ) ;
#24354=CARTESIAN_POINT ( 'NONE',  ( 17.16267987305034382, 22.47507462896901842, 6.831223922626973533 ) ) ;
#24358=AXIS2_PLACEMENT_3D ( 'NONE', #11944, #13658, #6069 ) ;
#24361=CARTESIAN_POINT ( 'NONE',  ( 3.834746474454188013E-15, 27.75624999877096855, 4.999999999999992006 ) ) ;
#24364=CARTESIAN_POINT ( 'NONE',  ( 1.878215178125000939, 29.56562499938548427, 12.25316411605952283 ) ) ;
#24368=CARTESIAN_POINT ( 'NONE',  ( -4.000000000000003553, -28.18750000000000000, 6.690598923241489970 ) ) ;
#24373=CARTESIAN_POINT ( 'NONE',  ( 3.959305671612554781E-15, 30.00000000000000355, 12.99999999999999289 ) ) ;
#24387=CARTESIAN_POINT ( 'NONE',  ( 20.51285331117640709, 15.20045855525759393, 8.999999999999992895 ) ) ;
#24389=CARTESIAN_POINT ( 'NONE',  ( 3.756430356250002323, 28.25312499938548427, 11.16877607737301226 ) ) ;
#24390=EDGE_CURVE ( 'NONE', #1927, #2390, #12197, .T. ) ;
#24392=CARTESIAN_POINT ( 'NONE',  ( 23.02516456238698694, 17.36831031289452909, 11.30940107675849760 ) ) ;
#24395=CYLINDRICAL_SURFACE ( 'NONE', #17651, 0.5000000000000001110 ) ;
#24396=CARTESIAN_POINT ( 'NONE',  ( -3.756430356250003211, -25.17812499938548498, 6.831223922626973533 ) ) ;
#24400=CARTESIAN_POINT ( 'NONE',  ( -4.000000000000003553, -28.60000000000000142, 8.999999999999992895 ) ) ;
#24410=CARTESIAN_POINT ( 'NONE',  ( 3.756430356249996105, -27.69062499938548072, 6.831223922626973533 ) ) ;
#24416=CARTESIAN_POINT ( 'NONE',  ( -3.959305739469038251E-15, -30.00000000000000355, 12.99999999999999289 ) ) ;
#24419=CARTESIAN_POINT ( 'NONE',  ( 17.29753586877772520, 19.95373324673703408, 12.25316411605951927 ) ) ;
#24420=CARTESIAN_POINT ( 'NONE',  ( 19.19352969096333439, 22.02195681570944785, 5.535898384862237620 ) ) ;
#24425=ORIENTED_EDGE ( 'NONE', *, *, #4982, .F. ) ;
#24427=CARTESIAN_POINT ( 'NONE',  ( 19.64299713866565611, 18.12724761081355140, 12.99999999999999467 ) ) ;
#24428=VERTEX_POINT ( 'NONE', #20416 ) ;
#24431=CARTESIAN_POINT ( 'NONE',  ( 1.878215178124995832, -26.19062499938548427, 5.746835883940462963 ) ) ;
#24437=ORIENTED_EDGE ( 'NONE', *, *, #19712, .F. ) ;
#24438=CARTESIAN_POINT ( 'NONE',  ( -3.756430356250002323, -26.00312499938548427, 11.16877607737301226 ) ) ;
#24439=ORIENTED_EDGE ( 'NONE', *, *, #24343, .T. ) ;
#24440=ORIENTED_EDGE ( 'NONE', *, *, #8103, .T. ) ;
#24442=FACE_OUTER_BOUND ( 'NONE', #10653, .T. ) ;
#24443=DIRECTION ( 'NONE',  ( 0.000000000000000000, 0.000000000000000000, 1.000000000000000000 ) ) ;
#24447=CARTESIAN_POINT ( 'NONE',  ( 3.735045420075836212E-15, 25.70312499938548001, 4.662447845253954171 ) ) ;
#24449=CARTESIAN_POINT ( 'NONE',  ( 3.999999999999997335, -28.86250000000000071, 11.30940107675849404 ) ) ;
#24453=CARTESIAN_POINT ( 'NONE',  ( 3.834746474454188013E-15, 28.65624999877096712, 4.999999999999992006 ) ) ;
#24454=CARTESIAN_POINT ( 'NONE',  ( 3.756430356249995661, -26.34062499938548285, 6.831223922626973533 ) ) ;
#24458=CARTESIAN_POINT ( 'NONE',  ( 0.2646063747045178660, -30.00000000000000000, 4.999999999999992895 ) ) ;
#24471=EDGE_CURVE ( 'NONE', #2042, #13481, #16397, .T. ) ;
#24477=CARTESIAN_POINT ( 'NONE',  ( 20.43103032403801578, 17.77483294607857189, 5.746835883940462963 ) ) ;
#24482=CARTESIAN_POINT ( 'NONE',  ( -3.756430356250003655, -25.19687499938548569, 8.999999999999992895 ) ) ;
#24483=CARTESIAN_POINT ( 'NONE',  ( -1.878215178124995832, 28.44062499938548427, 5.746835883940462963 ) ) ;
#24485=CARTESIAN_POINT ( 'NONE',  ( 4.000000000000001776, 27.60624999877096641, 11.30940107675849760 ) ) ;
#24489=EDGE_CURVE ( 'NONE', #5294, #21622, #14952, .T. ) ;
#24494=ADVANCED_FACE ( 'NONE', ( #22390 ), #10976, .T. ) ;
#24498=ORIENTED_EDGE ( 'NONE', *, *, #18335, .F. ) ;
#24499=EDGE_CURVE ( 'NONE', #7895, #24428, #15035, .T. ) ;
#24505=FACE_OUTER_BOUND ( 'NONE', #18276, .T. ) ;
#24506=CARTESIAN_POINT ( 'NONE',  ( -1.878215178124998497, 27.24062499938548498, 12.25316411605951927 ) ) ;
#24507=CARTESIAN_POINT ( 'NONE',  ( 18.09530447186750024, 18.09530447186743629, 13.33755215474603162 ) ) ;
#24511=CARTESIAN_POINT ( 'NONE',  ( -3.756430356250003211, -26.52812499938548285, 6.831223922626973533 ) ) ;
#24515=CARTESIAN_POINT ( 'NONE',  ( 3.999999999999996003, -29.23750000000000071, 6.690598923241487306 ) ) ;
#24521=ORIENTED_EDGE ( 'NONE', *, *, #24665, .T. ) ;
#24523=CARTESIAN_POINT ( 'NONE',  ( -3.756430356250003655, -26.15312499938548640, 8.999999999999992895 ) ) ;
#24529=CARTESIAN_POINT ( 'NONE',  ( 16.62584819264874270, 22.28270244214105134, 11.30940107675849404 ) ) ;
#24532=CARTESIAN_POINT ( 'NONE',  ( 3.756430356250003211, 25.17812499938548498, 6.831223922626973533 ) ) ;
#24534=CARTESIAN_POINT ( 'NONE',  ( 22.34249210749660364, 17.03009735157778337, 8.999999999999992895 ) ) ;
#24535=CARTESIAN_POINT ( 'NONE',  ( 22.03079565047434585, 16.37394140098190221, 11.30940107675849760 ) ) ;
#24536=CARTESIAN_POINT ( 'NONE',  ( 4.000000000000003553, 29.69687499938548569, 8.999999999999992895 ) ) ;
#24540=ORIENTED_EDGE ( 'NONE', *, *, #9570, .F. ) ;
#24545=CARTESIAN_POINT ( 'NONE',  ( 4.000000000000003553, 26.78124999877097068, 6.690598923241489970 ) ) ;
#24546=CARTESIAN_POINT ( 'NONE',  ( 3.756430356249995661, -27.12812499938548427, 6.831223922626973533 ) ) ;
#24548=ORIENTED_EDGE ( 'NONE', *, *, #10988, .T. ) ;
#24552=CARTESIAN_POINT ( 'NONE',  ( 3.756430356249996994, -25.36562499938548498, 8.999999999999992895 ) ) ;
#24557=EDGE_CURVE ( 'NONE', #14822, #10843, #20285, .T. ) ;
#24562=CARTESIAN_POINT ( 'NONE',  ( -3.756430356249997882, 26.30312499938548498, 11.16877607737301226 ) ) ;
#24570=CARTESIAN_POINT ( 'NONE',  ( 19.82550637751787548, 19.82550637751778666, 12.99999999999999289 ) ) ;
#24571=CARTESIAN_POINT ( 'NONE',  ( -3.735045420075836212E-15, -26.26562499938548356, 4.662447845253954171 ) ) ;
#24579=CYLINDRICAL_SURFACE ( 'NONE', #20402, 4.000000000000000000 ) ;
#24584=ORIENTED_EDGE ( 'NONE', *, *, #23874, .F. ) ;
#24587=EDGE_CURVE ( 'NONE', #6155, #5488, #1297, .T. ) ;
#24591=CARTESIAN_POINT ( 'NONE',  ( -1.878215178124995832, 29.00312499938548427, 5.746835883940462963 ) ) ;
#24592=EDGE_CURVE ( 'NONE', #476, #5606, #22968, .T. ) ;
#24596=PLANE ( 'NONE',  #24212 ) ;
#24610=FACE_OUTER_BOUND ( 'NONE', #11260, .T. ) ;
#24611=ORIENTED_EDGE ( 'NONE', *, *, #3089, .T. ) ;
#24625=CARTESIAN_POINT ( 'NONE',  ( -3.834746474454188013E-15, -27.36250000000000426, 4.999999999999992006 ) ) ;
#24626=EDGE_CURVE ( 'NONE', #19250, #10990, #4255, .T. ) ;
#24629=CARTESIAN_POINT ( 'NONE',  ( 19.20899765223631306, 19.20899765223624200, 4.662447845253954171 ) ) ;
#24632=CARTESIAN_POINT ( 'NONE',  ( 3.756430356250002323, 27.80312499938548143, 11.16877607737301226 ) ) ;
#24637=ADVANCED_FACE ( 'NONE', ( #11743, #3516, #25613 ), #25480, .T. ) ;
#24640=CARTESIAN_POINT ( 'NONE',  ( -3.756430356250003211, -27.42812499938548143, 6.831223922626973533 ) ) ;
#24643=ORIENTED_EDGE ( 'NONE', *, *, #2543, .T. ) ;
#24644=B_SPLINE_CURVE_WITH_KNOTS ( 'NONE', 3,
 ( #11354, #15286, #5603, #15793, #3630, #17262, #15673, #9398, #13581, #21549 ),
 .UNSPECIFIED., .F., .F.,
 ( 4, 2, 2, 2, 4 ),
 ( 0.01251976117704806969, 0.01338929815772730951, 0.01425883513840654759, 0.01512837211908578741, 0.01599790909976502723 ),
 .UNSPECIFIED. ) ;
#24650=CARTESIAN_POINT ( 'NONE',  ( 1.071796769724488563, -29.31115380933863790, 12.99999999999999289 ) ) ;
#24652=VECTOR ( 'NONE', #4565, 1000.000000000000000 ) ;
#24657=CARTESIAN_POINT ( 'NONE',  ( -1.878215178125000939, -26.97812499938548569, 12.25316411605952283 ) ) ;
#24658=CARTESIAN_POINT ( 'NONE',  ( -27.10000000000000497, 0.6000000000000000888, 19.59999999999999787 ) ) ;
#24664=FACE_OUTER_BOUND ( 'NONE', #24915, .T. ) ;
#24665=EDGE_CURVE ( 'NONE', #4649, #23534, #10431, .T. ) ;
#24670=CARTESIAN_POINT ( 'NONE',  ( 19.34820930021694352, 19.34820930021687246, 4.999999999999992006 ) ) ;
#24671=CARTESIAN_POINT ( 'NONE',  ( 1.999999999999998224, -28.39374999877096784, 12.46410161513774639 ) ) ;
#24672=CARTESIAN_POINT ( 'NONE',  ( 21.36138144860026600, 16.04898669268145639, 11.16877607737301226 ) ) ;
#24673=CARTESIAN_POINT ( 'NONE',  ( 16.74068927859332234, 19.39688665655263122, 12.25316411605951927 ) ) ;
#24675=AXIS2_PLACEMENT_3D ( 'NONE', #14076, #96, #12488 ) ;
#24677=CARTESIAN_POINT ( 'NONE',  ( -3.959305671612554781E-15, -30.00000000000000355, 12.99999999999999289 ) ) ;
#24687=CARTESIAN_POINT ( 'NONE',  ( -3.999999999999997335, 28.80624999877096926, 11.30940107675849404 ) ) ;
#24688=CARTESIAN_POINT ( 'NONE',  ( -1.878215178125000939, -25.96562499938548285, 12.25316411605952283 ) ) ;
#24694=CARTESIAN_POINT ( 'NONE',  ( -3.735045420075836212E-15, -25.70312499938548001, 4.662447845253954171 ) ) ;
#24701=CARTESIAN_POINT ( 'NONE',  ( 2.000000000000003997, 27.77500000000000213, 5.535898384862238508 ) ) ;
#24705=CARTESIAN_POINT ( 'NONE',  ( 3.756430356250002323, 28.70312499938548356, 11.16877607737301226 ) ) ;
#24709=CARTESIAN_POINT ( 'NONE',  ( 19.62663259444009611, 19.62663259444001085, 4.999999999999992006 ) ) ;
#24710=CARTESIAN_POINT ( 'NONE',  ( 23.26836714124207361, 18.93629030671969460, 11.57226653943513028 ) ) ;
#24713=CARTESIAN_POINT ( 'NONE',  ( 3.756430356249997882, -27.76562499938549067, 11.16877607737301226 ) ) ;
#24718=FACE_OUTER_BOUND ( 'NONE', #3111, .T. ) ;
#24720=PLANE ( 'NONE',  #25167 ) ;
#24735=CARTESIAN_POINT ( 'NONE',  ( -3.756430356249996105, 29.49062499938548498, 6.831223922626973533 ) ) ;
#24743=CARTESIAN_POINT ( 'NONE',  ( 6.741346781237209207, -25.16843286583315731, 20.00001199999999812 ) ) ;
#24748=EDGE_CURVE ( 'NONE', #15602, #2722, #18162, .T. ) ;
#24752=CARTESIAN_POINT ( 'NONE',  ( 1.071796769724494558, 27.73615380933863861, 4.999999999999992895 ) ) ;
#24762=CARTESIAN_POINT ( 'NONE',  ( 1.878215178124998497, -26.45312499938548711, 12.25316411605951927 ) ) ;
#24764=CARTESIAN_POINT ( 'NONE',  ( -3.469446951953614189E-15, -25.00000000000000000, 4.999999999999992006 ) ) ;
#24765=EDGE_CURVE ( 'NONE', #933, #23953, #12280, .T. ) ;
#24771=DIRECTION ( 'NONE',  ( 0.000000000000000000, 1.000000000000000000, 0.000000000000000000 ) ) ;
#24772=CARTESIAN_POINT ( 'NONE',  ( -0.7500000000000001110, 9.184850993605150903E-17, 17.00000000000000000 ) ) ;
#24773=CARTESIAN_POINT ( 'NONE',  ( 18.73170057493538820, 18.73170057493532781, 13.33755215474602984 ) ) ;
#24774=CARTESIAN_POINT ( 'NONE',  ( 3.756430356250004099, 29.22812499938548925, 6.831223922626973533 ) ) ;
#24781=CARTESIAN_POINT ( 'NONE',  ( -1.878215178125004048, -28.36562499938548143, 5.746835883940462963 ) ) ;
#24783=CARTESIAN_POINT ( 'NONE',  ( 0.000000000000000000, 0.000000000000000000, 15.00000000000000178 ) ) ;
#24788=VERTEX_POINT ( 'NONE', #21820 ) ;
#24793=CARTESIAN_POINT ( 'NONE',  ( -3.756430356250003211, -28.89062499938548356, 6.831223922626973533 ) ) ;
#24804=( BOUNDED_CURVE ( )  B_SPLINE_CURVE ( 2, ( #8452, #339, #18767, #18526, #6738, #6480, #16440, #24650, #2811 ),
 .UNSPECIFIED., .F., .F. ) 
 B_SPLINE_CURVE_WITH_KNOTS ( ( 3, 2, 2, 2, 3 ),
 ( 0.8250000000000000666, 0.8333333333333333703, 0.8499999999999999778, 0.8666666666666666963, 0.8750000000000000000 ),
 .UNSPECIFIED. ) 
 CURVE ( )  GEOMETRIC_REPRESENTATION_ITEM ( )  RATIONAL_B_SPLINE_CURVE ( ( 0.9330127018922194093, 0.9330127018922198534, 1.000000000000000000, 0.8660254037844387076, 1.000000000000000000, 0.8660254037844387076, 1.000000000000000000, 0.9330127018922194093, 0.9330127018922194093 ) ) 
 REPRESENTATION_ITEM ( '' )  );
#24807=CARTESIAN_POINT ( 'NONE',  ( 18.69544865292348490, 20.21119818077545460, 12.99999999999999467 ) ) ;
#24809=CARTESIAN_POINT ( 'NONE',  ( 18.11727402765218287, 23.42966878357085037, 6.831223922626973533 ) ) ;
#24810=CARTESIAN_POINT ( 'NONE',  ( 18.73170057493538820, 18.73170057493532781, 13.33755215474602984 ) ) ;
#24821=CARTESIAN_POINT ( 'NONE',  ( -3.999999999999996003, 28.28124999877096712, 6.690598923241487306 ) ) ;
#24822=CARTESIAN_POINT ( 'NONE',  ( 1.878215178124995832, -29.34062499938548285, 5.746835883940462963 ) ) ;
#24823=CARTESIAN_POINT ( 'NONE',  ( -3.999999999999996447, 25.22500000000000142, 8.999999999999992895 ) ) ;
#24825=CARTESIAN_POINT ( 'NONE',  ( 15.94967733227004558, 21.60653158176235777, 11.30940107675849404 ) ) ;
#24828=CARTESIAN_POINT ( 'NONE',  ( 3.756430356249997882, -25.85312499938548925, 11.16877607737301226 ) ) ;
#24838=CARTESIAN_POINT ( 'NONE',  ( 2.672651547586948120E-15, 28.62812499938548783, 13.33755215474602984 ) ) ;
#24847=CARTESIAN_POINT ( 'NONE',  ( 17.42265644678770187, 18.93840597463967512, 12.99999999999999467 ) ) ;
#24848=CARTESIAN_POINT ( 'NONE',  ( -1.878215178125004048, -26.67812499938548498, 5.746835883940462963 ) ) ;
#24850=LINE ( 'NONE', #16746, #11204 ) ;
#24851=CARTESIAN_POINT ( 'NONE',  ( 3.999999999999995559, -25.18750000000000000, 6.690598923241487306 ) ) ;
#24861=CARTESIAN_POINT ( 'NONE',  ( -3.834746474454188013E-15, -27.81249999999999645, 4.999999999999992006 ) ) ;
#24863=EDGE_CURVE ( 'NONE', #19630, #12953, #8883, .T. ) ;
#24865=CARTESIAN_POINT ( 'NONE',  ( 3.756430356250002323, 29.71562499938548640, 11.16877607737301403 ) ) ;
#24868=FACE_BOUND ( 'NONE', #21347, .T. ) ;
#24869=CARTESIAN_POINT ( 'NONE',  ( -2.000000000000003997, -25.46874999877096712, 5.535898384862238508 ) ) ;
#24876=CARTESIAN_POINT ( 'NONE',  ( -8.000000000000000000, 10.00000000000000178, 17.00000000000000000 ) ) ;
#24882=CARTESIAN_POINT ( 'NONE',  ( -5.577813053751546416E-15, -25.33750000000000213, 12.99999999999999289 ) ) ;
#24886=CARTESIAN_POINT ( 'NONE',  ( -1.859271017917182139E-15, -27.08124999877096784, 12.99999999999999289 ) ) ;
#24890=VERTEX_POINT ( 'NONE', #18660 ) ;
#24893=ORIENTED_EDGE ( 'NONE', *, *, #4942, .T. ) ;
#24900=CARTESIAN_POINT ( 'NONE',  ( 22.42204162038009230, 17.10964686446126848, 8.999999999999992895 ) ) ;
#24902=CARTESIAN_POINT ( 'NONE',  ( 2.000000000000003997, 25.07499999999999929, 5.535898384862238508 ) ) ;
#24903=ADVANCED_FACE ( 'NONE', ( #18791 ), #879, .F. ) ;
#24904=CARTESIAN_POINT ( 'NONE',  ( 22.44855812467459089, 17.13616336875576351, 6.831223922626973533 ) ) ;
#24909=CARTESIAN_POINT ( 'NONE',  ( -3.756430356250003211, -26.97812499938547859, 6.831223922626973533 ) ) ;
#24910=LINE ( 'NONE', #1103, #18781 ) ;
#24912=CARTESIAN_POINT ( 'NONE',  ( 4.000000000000002665, 29.87009603951200276, 10.45670610619353980 ) ) ;
#24915=EDGE_LOOP ( 'NONE', ( #19825, #11824, #753, #17395 ) ) ;
#24919=CARTESIAN_POINT ( 'NONE',  ( 1.859271017917182139E-15, 25.78750000000000142, 12.99999999999999289 ) ) ;
#24928=FACE_OUTER_BOUND ( 'NONE', #24304, .T. ) ;
#24929=CARTESIAN_POINT ( 'NONE',  ( -1.878215178124995832, 27.99062499938548143, 5.746835883940462963 ) ) ;
#24930=CARTESIAN_POINT ( 'NONE',  ( 21.71259759894040187, 16.05574334944795112, 11.30940107675849760 ) ) ;
#24931=CARTESIAN_POINT ( 'NONE',  ( 17.48087792458429135, 22.79327268050296240, 6.831223922626973533 ) ) ;
#24932=CARTESIAN_POINT ( 'NONE',  ( 20.89942480057588270, 20.89942480057580099, 4.381197846482986158 ) ) ;
#24935=CARTESIAN_POINT ( 'NONE',  ( 23.85222316637486273, 18.19536891688240843, 8.735714247490120599 ) ) ;
#24936=CARTESIAN_POINT ( 'NONE',  ( 20.96136040992792715, 18.30516303196848327, 12.25316411605952283 ) ) ;
#24937=DIRECTION ( 'NONE',  ( 0.000000000000000000, 0.000000000000000000, -1.000000000000000000 ) ) ;
#24940=CARTESIAN_POINT ( 'NONE',  ( 2.620986760973688460E-15, 27.98124999877096997, 13.61880215351699874 ) ) ;
#24941=CARTESIAN_POINT ( 'NONE',  ( -3.756430356250003655, -28.74062499938548498, 8.999999999999992895 ) ) ;
#24943=EDGE_LOOP ( 'NONE', ( #4697, #14940, #20856, #16973 ) ) ;
#24945=VERTEX_POINT ( 'NONE', #22726 ) ;
#24946=CARTESIAN_POINT ( 'NONE',  ( -3.735045420075836212E-15, -27.50312499938548783, 4.662447845253954171 ) ) ;
#24947=VERTEX_POINT ( 'NONE', #628 ) ;
#24949=CARTESIAN_POINT ( 'NONE',  ( 19.74889435023732887, 22.58381402607102473, 5.528701699505818468 ) ) ;
#24951=DIRECTION ( 'NONE',  ( 1.000000000000000000, 0.000000000000000000, 0.000000000000000000 ) ) ;
#24955=CARTESIAN_POINT ( 'NONE',  ( -1.859271017917182139E-15, -27.08124999877096784, 12.99999999999999289 ) ) ;
#24957=CARTESIAN_POINT ( 'NONE',  ( -3.756430356249996994, 28.51562499938548356, 8.999999999999992895 ) ) ;
#24958=EDGE_CURVE ( 'NONE', #125, #5938, #13128, .T. ) ;
#24964=EDGE_CURVE ( 'NONE', #22864, #1602, #20487, .T. ) ;
#24966=CARTESIAN_POINT ( 'NONE',  ( 3.756430356249995661, -28.14062499938548356, 6.831223922626973533 ) ) ;
#24969=CARTESIAN_POINT ( 'NONE',  ( 4.000000000000003553, 27.25000000000000000, 8.999999999999992895 ) ) ;
#24972=EDGE_CURVE ( 'NONE', #15499, #21679, #18476, .T. ) ;
#24976=ORIENTED_EDGE ( 'NONE', *, *, #18142, .F. ) ;
#24979=EDGE_LOOP ( 'NONE', ( #8970, #24498, #12632, #2520 ) ) ;
#24985=CARTESIAN_POINT ( 'NONE',  ( 1.878215178125000939, 29.67812499938548498, 12.25316411605952283 ) ) ;
#24990=EDGE_CURVE ( 'NONE', #15349, #11855, #10269, .T. ) ;
#24991=CARTESIAN_POINT ( 'NONE',  ( 3.403349963601436823, -25.83240171513484995, 20.00001200000000878 ) ) ;
#24995=CARTESIAN_POINT ( 'NONE',  ( 0.000000000000000000, 0.000000000000000000, 17.00000000000000000 ) ) ;
#24999=CARTESIAN_POINT ( 'NONE',  ( -30.00000000000000355, 0.000000000000000000, 0.000000000000000000 ) ) ;
#25004=EDGE_LOOP ( 'NONE', ( #24540, #24105, #13530, #21986 ) ) ;
#25005=EDGE_CURVE ( 'NONE', #8582, #15499, #4131, .T. ) ;
#25008=ORIENTED_EDGE ( 'NONE', *, *, #9035, .T. ) ;
#25009=CARTESIAN_POINT ( 'NONE',  ( -1.878215178125004048, -26.67812499938548498, 5.746835883940462963 ) ) ;
#25019=AXIS2_PLACEMENT_3D ( 'NONE', #15837, #1974, #9941 ) ;
#25022=CARTESIAN_POINT ( 'NONE',  ( 21.44093096148375466, 16.12853620556493794, 11.16877607737301226 ) ) ;
#25024=CARTESIAN_POINT ( 'NONE',  ( 2.672651547586948120E-15, 29.52812499938548285, 13.33755215474602984 ) ) ;
#25025=CARTESIAN_POINT ( 'NONE',  ( 18.64987758779700044, 21.30607496575630222, 12.25316411605951927 ) ) ;
#25028=EDGE_CURVE ( 'NONE', #22241, #25114, #2410, .T. ) ;
#25033=CARTESIAN_POINT ( 'NONE',  ( 1.878215178124998497, -28.14062499938548356, 12.25316411605951927 ) ) ;
#25042=FACE_OUTER_BOUND ( 'NONE', #1985, .T. ) ;
#25046=CARTESIAN_POINT ( 'NONE',  ( -3.756430356250003211, -28.44062499938548427, 6.831223922626973533 ) ) ;
#25051=CARTESIAN_POINT ( 'NONE',  ( 22.44180146790808905, 16.78494721841563475, 6.690598923241489970 ) ) ;
#25058=CARTESIAN_POINT ( 'NONE',  ( 2.672651547586948120E-15, 26.37812499938548427, 13.33755215474603162 ) ) ;
#25061=CARTESIAN_POINT ( 'NONE',  ( 18.88852612644745932, 21.54472350440676109, 12.25316411605951927 ) ) ;
#25062=CARTESIAN_POINT ( 'NONE',  ( 18.12403068441868470, 23.78088493391098979, 6.690598923241487306 ) ) ;
#25064=CARTESIAN_POINT ( 'NONE',  ( 17.20921128712764414, 22.86606553661995278, 6.690598923241487306 ) ) ;
#25069=CARTESIAN_POINT ( 'NONE',  ( 20.64316235839397962, 17.98696498043453573, 12.25316411605952283 ) ) ;
#25070=CARTESIAN_POINT ( 'NONE',  ( 23.67481891673307715, 18.01796466724061929, 6.690598923241489970 ) ) ;
#25073=CARTESIAN_POINT ( 'NONE',  ( -1.999999999999995781, 27.79374999877096997, 5.535898384862237620 ) ) ;
#25074=CARTESIAN_POINT ( 'NONE',  ( -4.000000000000003553, -25.00000000000000000, 8.999999999999992895 ) ) ;
#25075=CARTESIAN_POINT ( 'NONE',  ( -1.999999999999995781, 25.54374999877096997, 5.535898384862237620 ) ) ;
#25079=EDGE_CURVE ( 'NONE', #8492, #8072, #5112, .T. ) ;
#25081=CARTESIAN_POINT ( 'NONE',  ( 3.756430356249995661, -28.47812499938548569, 6.831223922626973533 ) ) ;
#25082=ORIENTED_EDGE ( 'NONE', *, *, #9962, .F. ) ;
#25084=CARTESIAN_POINT ( 'NONE',  ( 20.28273967276687628, 22.10586454194350736, 12.79562863665509553 ) ) ;
#25089=AXIS2_PLACEMENT_3D ( 'NONE', #6406, #149, #7985 ) ;
#25100=CARTESIAN_POINT ( 'NONE',  ( -1.071796769724495668, -27.55134618820330061, 12.99999999999999112 ) ) ;
#25101=CARTESIAN_POINT ( 'NONE',  ( -3.735045420075836212E-15, -28.96562499938548640, 4.662447845253954171 ) ) ;
#25106=VERTEX_POINT ( 'NONE', #6099 ) ;
#25112=VERTEX_POINT ( 'NONE', #8460 ) ;
#25114=VERTEX_POINT ( 'NONE', #20470 ) ;
#25116=( BOUNDED_CURVE ( )  B_SPLINE_CURVE ( 2, ( #23147, #5610, #1049, #13591, #7053, #15041, #3138, #5226, #13206 ),
 .UNSPECIFIED., .F., .F. ) 
 B_SPLINE_CURVE_WITH_KNOTS ( ( 3, 2, 2, 2, 3 ),
 ( 0.1250000000000000000, 0.1333333333333333315, 0.1499999999999999944, 0.1666666666666666574, 0.1749999999999999889 ),
 .UNSPECIFIED. ) 
 CURVE ( )  GEOMETRIC_REPRESENTATION_ITEM ( )  RATIONAL_B_SPLINE_CURVE ( ( 0.9330127018922194093, 0.9330127018922194093, 1.000000000000000000, 0.8660254037844387076, 1.000000000000000000, 0.8660254037844387076, 1.000000000000000000, 0.9330127018922194093, 0.9330127018922194093 ) ) 
 REPRESENTATION_ITEM ( '' )  );
#25117=FACE_OUTER_BOUND ( 'NONE', #4585, .T. ) ;
#25121=( BOUNDED_CURVE ( )  B_SPLINE_CURVE ( 2, ( #7572, #3639, #2072, #3521, #17509, #13709, #10040, #7702, #9526 ),
 .UNSPECIFIED., .F., .F. ) 
 B_SPLINE_CURVE_WITH_KNOTS ( ( 3, 2, 2, 2, 3 ),
 ( 0.7750000000000000222, 0.7833333333333333259, 0.8000000000000000444, 0.8166666666666666519, 0.8250000000000000666 ),
 .UNSPECIFIED. ) 
 CURVE ( )  GEOMETRIC_REPRESENTATION_ITEM ( )  RATIONAL_B_SPLINE_CURVE ( ( 0.9330127018922194093, 0.9330127018922194093, 1.000000000000000000, 0.8660254037844387076, 1.000000000000000000, 0.8660254037844387076, 1.000000000000000000, 0.9330127018922189652, 0.9330127018922194093 ) ) 
 REPRESENTATION_ITEM ( '' )  );
#25124=CARTESIAN_POINT ( 'NONE',  ( 19.20672417798141041, 21.86292155594071218, 12.25316411605951927 ) ) ;
#25127=CARTESIAN_POINT ( 'NONE',  ( -3.756430356249996994, 26.37812499938548783, 8.999999999999992895 ) ) ;
#25135=CARTESIAN_POINT ( 'NONE',  ( 3.999999999999996003, -25.58124999877097139, 6.690598923241487306 ) ) ;
#25142=ORIENTED_EDGE ( 'NONE', *, *, #8912, .F. ) ;
#25144=CARTESIAN_POINT ( 'NONE',  ( 17.67766952966372429, 17.67766952966365324, 4.999999999999992006 ) ) ;
#25146=CARTESIAN_POINT ( 'NONE',  ( 3.756430356249996994, -26.82812499938548711, 8.999999999999992895 ) ) ;
#25147=ORIENTED_EDGE ( 'NONE', *, *, #11775, .F. ) ;
#25149=VECTOR ( 'NONE', #25509, 1000.000000000000000 ) ;
#25155=CARTESIAN_POINT ( 'NONE',  ( 3.999999999999995559, -29.23750000000000071, 6.690598923241487306 ) ) ;
#25158=CYLINDRICAL_SURFACE ( 'NONE', #21012, 4.000000000000000000 ) ;
#25162=CARTESIAN_POINT ( 'NONE',  ( 17.69528343319515784, 20.35148081115446317, 12.25316411605951927 ) ) ;
#25163=EDGE_CURVE ( 'NONE', #13512, #8734, #21133, .T. ) ;
#25165=AXIS2_PLACEMENT_3D ( 'NONE', #4586, #12566, #19475 ) ;
#25166=CARTESIAN_POINT ( 'NONE',  ( -3.756430356249997882, 29.45312499938548356, 11.16877607737301226 ) ) ;
#25167=AXIS2_PLACEMENT_3D ( 'NONE', #2486, #18195, #12299 ) ;
#25168=CARTESIAN_POINT ( 'NONE',  ( 16.34066823992097994, 21.65306299583965455, 11.16877607737301048 ) ) ;
#25169=DIRECTION ( 'NONE',  ( 0.000000000000000000, -1.000000000000000000, 0.000000000000000000 ) ) ;
#25174=CARTESIAN_POINT ( 'NONE',  ( 3.756430356249997438, -29.00312499938548072, 11.16877607737301048 ) ) ;
#25176=DIRECTION ( 'NONE',  ( 1.000000000000000000, 0.000000000000000000, 0.000000000000000000 ) ) ;
#25180=EDGE_LOOP ( 'NONE', ( #14586, #8914, #7565, #3016 ) ) ;
#25181=DIRECTION ( 'NONE',  ( 0.000000000000000000, -1.000000000000000000, 0.000000000000000000 ) ) ;
#25183=DIRECTION ( 'NONE',  ( -1.000000000000000000, 0.000000000000000000, 0.000000000000000000 ) ) ;
#25185=CARTESIAN_POINT ( 'NONE',  ( -3.756430356250002323, -29.71562499938548640, 11.16877607737301403 ) ) ;
#25198=LINE ( 'NONE', #7278, #9651 ) ;
#25201=CARTESIAN_POINT ( 'NONE',  ( 3.735045420075836212E-15, 26.60312499938547859, 4.662447845253954171 ) ) ;
#25202=FACE_BOUND ( 'NONE', #3147, .T. ) ;
#25203=CARTESIAN_POINT ( 'NONE',  ( 19.78131220369370169, 16.95288507894744257, 5.535898384862238508 ) ) ;
#25204=CARTESIAN_POINT ( 'NONE',  ( 18.25440349763447756, 18.25440349763440295, 4.662447845253954171 ) ) ;
#25205=CARTESIAN_POINT ( 'NONE',  ( 16.24135887950949808, 21.89821312900181027, 8.999999999999992895 ) ) ;
#25208=CARTESIAN_POINT ( 'NONE',  ( 22.68720666332504265, 17.37481190740622239, 6.831223922626973533 ) ) ;
#25211=CARTESIAN_POINT ( 'NONE',  ( -3.756430356249997882, 26.41562499938548569, 11.16877607737301226 ) ) ;
#25212=CARTESIAN_POINT ( 'NONE',  ( -1.878215178125000939, -28.21562499938548640, 12.25316411605952283 ) ) ;
#25217=CARTESIAN_POINT ( 'NONE',  ( 3.756430356249997882, -28.10312499938548569, 11.16877607737301226 ) ) ;
#25226=CARTESIAN_POINT ( 'NONE',  ( -0.5000000000000001110, 10.00000000000000000, 13.00000000000000178 ) ) ;
#25231=DIRECTION ( 'NONE',  ( 0.000000000000000000, 0.000000000000000000, -1.000000000000000000 ) ) ;
#25234=CARTESIAN_POINT ( 'NONE',  ( -3.756430356250003655, -28.40312499938548640, 8.999999999999992895 ) ) ;
#25238=DIRECTION ( 'NONE',  ( 0.000000000000000000, 0.000000000000000000, -1.000000000000000000 ) ) ;
#25256=CARTESIAN_POINT ( 'NONE',  ( -1.878215178124995832, 25.40312499938548640, 5.746835883940462963 ) ) ;
#25264=CARTESIAN_POINT ( 'NONE',  ( -2.620986760973688460E-15, -25.73124999877096997, 13.61880215351699874 ) ) ;
#25272=ORIENTED_EDGE ( 'NONE', *, *, #19907, .F. ) ;
#25274=EDGE_LOOP ( 'NONE', ( #5868, #25276, #19171, #21762 ) ) ;
#25275=CARTESIAN_POINT ( 'NONE',  ( 3.756430356249996994, -29.07812499938548356, 8.999999999999992895 ) ) ;
#25276=ORIENTED_EDGE ( 'NONE', *, *, #15479, .T. ) ;
#25277=CARTESIAN_POINT ( 'NONE',  ( -1.999999999999995781, 28.75000000000000000, 5.535898384862237620 ) ) ;
#25284=CARTESIAN_POINT ( 'NONE',  ( 18.01575495898401513, 18.01575495898394408, 13.33755215474602984 ) ) ;
#25285=DIRECTION ( 'NONE',  ( 1.000000000000000000, 0.000000000000000000, 0.000000000000000000 ) ) ;
#25287=CARTESIAN_POINT ( 'NONE',  ( 4.000000000000001776, 25.86250000000000071, 11.30940107675849760 ) ) ;
#25289=CARTESIAN_POINT ( 'NONE',  ( 18.57260154916842154, 18.57260154916834693, 4.662447845253954171 ) ) ;
#25300=LINE ( 'NONE', #21504, #5460 ) ;
#25315=CARTESIAN_POINT ( 'NONE',  ( -3.756430356249997438, 25.85312499938548569, 11.16877607737301048 ) ) ;
#25318=CARTESIAN_POINT ( 'NONE',  ( 22.66069015903055117, 17.34829540311172735, 8.999999999999992895 ) ) ;
#25319=CARTESIAN_POINT ( 'NONE',  ( 22.44855812467459089, 17.13616336875576351, 6.831223922626973533 ) ) ;
#25322=DIRECTION ( 'NONE',  ( 0.000000000000000000, 0.000000000000000000, -1.000000000000000000 ) ) ;
#25323=CARTESIAN_POINT ( 'NONE',  ( 20.32496430686003208, 17.66876692890059530, 12.25316411605952283 ) ) ;
#25327=CARTESIAN_POINT ( 'NONE',  ( -3.756430356249996994, 25.92812499938548498, 8.999999999999992895 ) ) ;
#25328=CARTESIAN_POINT ( 'NONE',  ( 1.999999999999995781, -25.15000000000000213, 5.535898384862237620 ) ) ;
#25331=ORIENTED_EDGE ( 'NONE', *, *, #2089, .T. ) ;
#25333=EDGE_CURVE ( 'NONE', #19280, #15184, #11659, .T. ) ;
#25334=CARTESIAN_POINT ( 'NONE',  ( 17.18149551509901940, 19.58805710660145039, 20.00001200000000168 ) ) ;
#25335=CARTESIAN_POINT ( 'NONE',  ( -3.735045420075836212E-15, -28.40312499938548640, 4.662447845253954171 ) ) ;
#25343=DIRECTION ( 'NONE',  ( 0.000000000000000000, 0.000000000000000000, -1.000000000000000000 ) ) ;
#25345=DIRECTION ( 'NONE',  ( 0.000000000000000000, -1.000000000000000000, 0.000000000000000000 ) ) ;
#25348=CARTESIAN_POINT ( 'NONE',  ( -3.834746474454188013E-15, -27.75624999877096855, 4.999999999999992006 ) ) ;
#25349=CARTESIAN_POINT ( 'NONE',  ( -2.672651547586948120E-15, -29.19062499938548783, 13.33755215474602984 ) ) ;
#25353=EDGE_CURVE ( 'NONE', #23031, #4358, #15338, .T. ) ;
#25354=CARTESIAN_POINT ( 'NONE',  ( 3.470226642398214878, -29.79897209676519765, 11.00633161724385900 ) ) ;
#25356=CARTESIAN_POINT ( 'NONE',  ( 21.21320343559646915, 21.21320343559638744, 12.99999999999999289 ) ) ;
#25372=CARTESIAN_POINT ( 'NONE',  ( 1.878215178125004048, 28.47812499938548569, 5.746835883940462963 ) ) ;
#25376=CARTESIAN_POINT ( 'NONE',  ( -3.834746474454188013E-15, -25.95624999877096428, 4.999999999999992006 ) ) ;
#25379=CARTESIAN_POINT ( 'NONE',  ( 3.999999999999996003, -27.38124999877096855, 6.690598923241487306 ) ) ;
#25381=CARTESIAN_POINT ( 'NONE',  ( 0.000000000000000000, 10.00000000000000000, 17.00000000000000000 ) ) ;
#25388=ADVANCED_FACE ( 'NONE', ( #18885 ), #25158, .F. ) ;
#25392=CARTESIAN_POINT ( 'NONE',  ( -3.756430356250004099, -27.54062499938548569, 6.831223922626973533 ) ) ;
#25402=CARTESIAN_POINT ( 'NONE',  ( 19.49840572522085935, 22.15460310318015758, 5.746835883940462963 ) ) ;
#25403=DIRECTION ( 'NONE',  ( -1.000000000000000000, 0.000000000000000000, -0.000000000000000000 ) ) ;
#25405=CARTESIAN_POINT ( 'NONE',  ( -3.756430356249995661, 29.37812499938548427, 6.831223922626973533 ) ) ;
#25406=CARTESIAN_POINT ( 'NONE',  ( 20.72271187127746828, 18.06651449331802439, 12.25316411605952283 ) ) ;
#25409=VERTEX_POINT ( 'NONE', #17432 ) ;
#25411=CARTESIAN_POINT ( 'NONE',  ( 4.000000000000001776, 28.11250000000000071, 11.30940107675849760 ) ) ;
#25416=CARTESIAN_POINT ( 'NONE',  ( -3.137519842735244810E-15, 27.30624999877096926, 4.999999999999991118 ) ) ;
#25428=CARTESIAN_POINT ( 'NONE',  ( 1.859271017917182139E-15, 28.48749999999999716, 12.99999999999999289 ) ) ;
#25432=CARTESIAN_POINT ( 'NONE',  ( 3.756430356250004099, 28.77812499938548285, 6.831223922626973533 ) ) ;
#25433=CARTESIAN_POINT ( 'NONE',  ( -1.999999999999998224, 27.10000000000000142, 12.46410161513774639 ) ) ;
#25436=CARTESIAN_POINT ( 'NONE',  ( 3.756430356250003655, 26.94062499938548427, 8.999999999999992895 ) ) ;
#25438=DIRECTION ( 'NONE',  ( 0.000000000000000000, -1.000000000000000000, 0.000000000000000000 ) ) ;
#25439=CARTESIAN_POINT ( 'NONE',  ( 22.44180146790808905, 16.78494721841563475, 6.690598923241489970 ) ) ;
#25440=CARTESIAN_POINT ( 'NONE',  ( 17.61346044605677008, 22.92585520197544469, 11.16877607737301226 ) ) ;
#25441=CARTESIAN_POINT ( 'NONE',  ( 17.23572779142213918, 22.89258204091444782, 8.999999999999992895 ) ) ;
#25442=CYLINDRICAL_SURFACE ( 'NONE', #18164, 4.000000000000000000 ) ;
#25444=CARTESIAN_POINT ( 'NONE',  ( 16.84448182151639628, 22.15687657743507089, 6.831223922626973533 ) ) ;
#25446=CARTESIAN_POINT ( 'NONE',  ( 0.000000000000000000, 0.000000000000000000, 17.00000000000000000 ) ) ;
#25448=CARTESIAN_POINT ( 'NONE',  ( 19.32479908713171213, 17.80904955927959676, 12.99999999999999112 ) ) ;
#25450=CARTESIAN_POINT ( 'NONE',  ( 3.999999999999996003, -26.08750000000000213, 6.690598923241487306 ) ) ;
#25454=VECTOR ( 'NONE', #11175, 1000.000000000000000 ) ;
#25455=CARTESIAN_POINT ( 'NONE',  ( -3.959305671612554781E-15, -30.00000000000000355, 12.99999999999999289 ) ) ;
#25457=CARTESIAN_POINT ( 'NONE',  ( 23.36965697125207342, 11.52193136556788211, 20.00001200000000523 ) ) ;
#25460=ORIENTED_EDGE ( 'NONE', *, *, #9072, .F. ) ;
#25471=AXIS2_PLACEMENT_3D ( 'NONE', #11126, #20813, #2897 ) ;
#25475=CARTESIAN_POINT ( 'NONE',  ( -1.071796769724490117, 26.48259618943233562, 4.999999999999992895 ) ) ;
#25480=CYLINDRICAL_SURFACE ( 'NONE', #6332, 30.00000000000000355 ) ;
#25481=CARTESIAN_POINT ( 'NONE',  ( -3.756430356250004099, -28.44062499938548783, 6.831223922626973533 ) ) ;
#25490=CARTESIAN_POINT ( 'NONE',  ( 3.999999999999997335, -26.55624999877096570, 11.30940107675849404 ) ) ;
#25491=ORIENTED_EDGE ( 'NONE', *, *, #22581, .F. ) ;
#25493=VECTOR ( 'NONE', #1377, 1000.000000000000000 ) ;
#25497=LINE ( 'NONE', #13604, #15145 ) ;
#25498=( BOUNDED_CURVE ( )  B_SPLINE_CURVE ( 2, ( #1436, #3905, #11609, #5477, #21683, #15421, #15681, #17892, #23649 ),
 .UNSPECIFIED., .F., .F. ) 
 B_SPLINE_CURVE_WITH_KNOTS ( ( 3, 2, 2, 2, 3 ),
 ( 0.1750000000000000167, 0.1833333333333333204, 0.2000000000000000111, 0.2166666666666666741, 0.2250000000000000056 ),
 .UNSPECIFIED. ) 
 CURVE ( )  GEOMETRIC_REPRESENTATION_ITEM ( )  RATIONAL_B_SPLINE_CURVE ( ( 0.9330127018922194093, 0.9330127018922196314, 1.000000000000000000, 0.8660254037844387076, 1.000000000000000000, 0.8660254037844387076, 1.000000000000000000, 0.9330127018922194093, 0.9330127018922194093 ) ) 
 REPRESENTATION_ITEM ( '' )  );
#25499=CARTESIAN_POINT ( 'NONE',  ( -1.071796769724498999, -28.00134618820329635, 12.99999999999998757 ) ) ;
#25500=VECTOR ( 'NONE', #6249, 1000.000000000000000 ) ;
#25506=CARTESIAN_POINT ( 'NONE',  ( 2.672651547586948120E-15, 28.29062499938548569, 13.33755215474602984 ) ) ;
#25508=CARTESIAN_POINT ( 'NONE',  ( -2.000000000000000888, -26.66874999877096641, 12.46410161513774817 ) ) ;
#25509=DIRECTION ( 'NONE',  ( -0.7071067811865487940, -0.7071067811865463515, 0.000000000000000000 ) ) ;
#25510=VECTOR ( 'NONE', #21924, 1000.000000000000000 ) ;
#25515=CARTESIAN_POINT ( 'NONE',  ( 1.999999999999995781, -26.89374999877097139, 5.535898384862237620 ) ) ;
#25517=VECTOR ( 'NONE', #19107, 1000.000000000000000 ) ;
#25518=CARTESIAN_POINT ( 'NONE',  ( 3.756430356250003655, 28.40312499938548640, 8.999999999999992895 ) ) ;
#25522=CARTESIAN_POINT ( 'NONE',  ( -1.859271017917182139E-15, -28.88124999877096499, 12.99999999999999289 ) ) ;
#25529=ORIENTED_EDGE ( 'NONE', *, *, #4012, .T. ) ;
#25530=B_SPLINE_CURVE_WITH_KNOTS ( 'NONE', 3,
 ( #2648, #3036, #4596, #17025, #22783, #23043, #3155, #950, #15067, #21079, #20810, #12717, #16908, #13108, #4860, #8652, #6685, #6557, #24991, #24743, #12969, #14678, #22904, #9043, #2893, #12836, #20953, #10860, #7077, #10609, #11123, #10729, #22658, #19101 ),
 .UNSPECIFIED., .F., .F.,
 ( 4, 2, 2, 2, 2, 2, 2, 2, 2, 2, 2, 2, 2, 2, 2, 2, 4 ),
 ( 0.5000000000000000000, 0.5312500000000000000, 0.5625000000000000000, 0.5937500000000000000, 0.6250000000000000000, 0.6562500000000000000, 0.6875000000000000000, 0.7187500000000000000, 0.7500000000000000000, 0.7812500000000000000, 0.8125000000000000000, 0.8437500000000000000, 0.8750000000000000000, 0.9062500000000000000, 0.9375000000000000000, 0.9687500000000000000, 1.000000000000000000 ),
 .UNSPECIFIED. ) ;
#25531=CARTESIAN_POINT ( 'NONE',  ( -1.878215178125000939, -29.22812499938548569, 12.25316411605952283 ) ) ;
#25535=VERTEX_POINT ( 'NONE', #13519 ) ;
#25541=DIRECTION ( 'NONE',  ( 0.000000000000000000, -1.000000000000000000, 0.000000000000000000 ) ) ;
#25542=CARTESIAN_POINT ( 'NONE',  ( 17.56042743746777646, 22.87282219338644751, 6.831223922626973533 ) ) ;
#25546=CARTESIAN_POINT ( 'NONE',  ( -3.999999999999996447, 27.47499999999999787, 8.999999999999992895 ) ) ;
#25555=ADVANCED_FACE ( 'NONE', ( #15609 ), #21218, .F. ) ;
#25569=LINE ( 'NONE', #3856, #24278 ) ;
#25571=CARTESIAN_POINT ( 'NONE',  ( 3.756430356250003655, 28.74062499938548498, 8.999999999999992895 ) ) ;
#25573=CARTESIAN_POINT ( 'NONE',  ( 3.999999999999997335, -28.80624999877096926, 11.30940107675849404 ) ) ;
#25574=CARTESIAN_POINT ( 'NONE',  ( 3.756430356250002323, 28.70312499938548356, 11.16877607737301403 ) ) ;
#25575=EDGE_CURVE ( 'NONE', #12924, #8943, #10660, .T. ) ;
#25576=CARTESIAN_POINT ( 'NONE',  ( -2.007320019195686811, -29.93357098804190741, 5.530155478426868498 ) ) ;
#25577=CARTESIAN_POINT ( 'NONE',  ( 20.41770830676159676, 17.58928118201533408, 5.535898384862238508 ) ) ;
#25578=CARTESIAN_POINT ( 'NONE',  ( 21.78337204305729458, 19.12717466509784003, 5.746835883940462963 ) ) ;
#25583=CARTESIAN_POINT ( 'NONE',  ( 17.79907597611823533, 23.11147073203690994, 6.831223922626973533 ) ) ;
#25587=CARTESIAN_POINT ( 'NONE',  ( 1.999999999999998224, -26.20000000000000284, 12.46410161513774639 ) ) ;
#25594=CARTESIAN_POINT ( 'NONE',  ( 26.00000000000000355, 1.592040838891558898E-15, 20.00000599999999906 ) ) ;
#25596=ORIENTED_EDGE ( 'NONE', *, *, #10988, .F. ) ;
#25601=VECTOR ( 'NONE', #15886, 1000.000000000000000 ) ;
#25602=LINE ( 'NONE', #8078, #16283 ) ;
#25611=CARTESIAN_POINT ( 'NONE',  ( 18.99023649137220104, 18.99023649137212288, 4.381197846482986158 ) ) ;
#25613=FACE_OUTER_BOUND ( 'NONE', #11190, .T. ) ;
#25614=CARTESIAN_POINT ( 'NONE',  ( 3.756430356249995661, -29.49062499938548498, 6.831223922626973533 ) ) ;
#25619=CARTESIAN_POINT ( 'NONE',  ( -1.999999999999998224, 26.59374999877096712, 12.46410161513774639 ) ) ;
#25622=CARTESIAN_POINT ( 'NONE',  ( 3.999999999999995559, -26.93124999877096926, 6.690598923241487306 ) ) ;
#25624=CARTESIAN_POINT ( 'NONE',  ( -3.834746474454188013E-15, -26.40624999877096357, 4.999999999999992006 ) ) ;
#25631=EDGE_CURVE ( 'NONE', #1348, #18727, #19450, .T. ) ;
#25639=CARTESIAN_POINT ( 'NONE',  ( 3.756430356250003655, 29.30312499938548498, 8.999999999999992895 ) ) ;
#25642=CARTESIAN_POINT ( 'NONE',  ( 18.12403068441868470, 23.78088493391098979, 6.690598923241487306 ) ) ;
#25644=CARTESIAN_POINT ( 'NONE',  ( 1.859271017917182139E-15, 28.93749999999999645, 12.99999999999999289 ) ) ;
#25648=CARTESIAN_POINT ( 'NONE',  ( -2.000000000000000888, -26.66874999877096641, 12.46410161513774817 ) ) ;
#25649=CARTESIAN_POINT ( 'NONE',  ( -1.878215178124998497, 28.70312499938548356, 12.25316411605951927 ) ) ;
#25655=ORIENTED_EDGE ( 'NONE', *, *, #12593, .F. ) ;
#25656=( BOUNDED_CURVE ( )  B_SPLINE_CURVE ( 2, ( #4181, #21850, #14127 ),
 .UNSPECIFIED., .F., .F. ) 
 B_SPLINE_CURVE_WITH_KNOTS ( ( 3, 3 ),
 ( 0.9889400238386636399, 1.000000000000000000 ),
 .UNSPECIFIED. ) 
 CURVE ( )  GEOMETRIC_REPRESENTATION_ITEM ( )  RATIONAL_B_SPLINE_CURVE ( ( 0.9401842259098239785, 0.9110946495778740051, 1.000000000000000000 ) ) 
 REPRESENTATION_ITEM ( '' )  );
#25659=ORIENTED_EDGE ( 'NONE', *, *, #20142, .F. ) ;
#25660=CARTESIAN_POINT ( 'NONE',  ( 1.878215178124998497, -27.35312499938548569, 12.25316411605951927 ) ) ;
#25671=CARTESIAN_POINT ( 'NONE',  ( 21.35910797434536335, 18.70291059638591946, 12.25316411605952283 ) ) ;
#25674=CARTESIAN_POINT ( 'NONE',  ( -3.999999999999996447, 27.02500000000000213, 8.999999999999992895 ) ) ;
#25679=ORIENTED_EDGE ( 'NONE', *, *, #15303, .F. ) ;
#25681=ORIENTED_EDGE ( 'NONE', *, *, #25697, .F. ) ;
#25685=CARTESIAN_POINT ( 'NONE',  ( 17.01355443044479898, 18.52930395829678289, 4.999999999999992895 ) ) ;
#25686=ORIENTED_EDGE ( 'NONE', *, *, #13214, .T. ) ;
#25690=ORIENTED_EDGE ( 'NONE', *, *, #19030, .T. ) ;
#25692=DIRECTION ( 'NONE',  ( 0.000000000000000000, 0.000000000000000000, 1.000000000000000000 ) ) ;
#25697=EDGE_CURVE ( 'NONE', #13143, #15567, #19221, .T. ) ;
#25698=CARTESIAN_POINT ( 'NONE',  ( -3.756430356249996994, 25.36562499938548498, 8.999999999999992895 ) ) ;
#25703=CARTESIAN_POINT ( 'NONE',  ( 17.00591808753650724, 19.83434521228262426, 5.535898384862237620 ) ) ;
#25704=CARTESIAN_POINT ( 'NONE',  ( 19.84539375530421168, 19.84539375530412997, 4.662447845253954171 ) ) ;
#25707=CARTESIAN_POINT ( 'NONE',  ( 21.58253194665774188, 20.83893265812701046, 5.025965267902964939 ) ) ;
#25708=CARTESIAN_POINT ( 'NONE',  ( 22.97888821056449515, 17.66649345464567489, 8.999999999999992895 ) ) ;
#25709=CARTESIAN_POINT ( 'NONE',  ( 3.878215178125003604, 29.57031249969274356, 8.999999999999992895 ) ) ;
#25712=CARTESIAN_POINT ( 'NONE',  ( -4.000000000000003553, -25.48750000000000071, 6.690598923241489970 ) ) ;
#25720=ORIENTED_EDGE ( 'NONE', *, *, #202, .F. ) ;
#25730=CARTESIAN_POINT ( 'NONE',  ( 4.000000000000001776, 28.56249999999999645, 11.30940107675849760 ) ) ;
#25731=CARTESIAN_POINT ( 'NONE',  ( 18.17485398475098535, 18.17485398475091785, 4.662447845253954171 ) ) ;
#25732=LINE ( 'NONE', #13839, #1353 ) ;
#25741=CARTESIAN_POINT ( 'NONE',  ( 3.999999999999997335, -27.00624999877096855, 11.30940107675849404 ) ) ;
#25742=FACE_OUTER_BOUND ( 'NONE', #9295, .T. ) ;
#25743=CARTESIAN_POINT ( 'NONE',  ( -8.831537335106614961E-15, -26.63124999877096855, 12.99999999999999112 ) ) ;
#25747=ORIENTED_EDGE ( 'NONE', *, *, #12019, .F. ) ;
#25749=CARTESIAN_POINT ( 'NONE',  ( 18.67203843983824996, 18.67203843983818246, 4.999999999999991118 ) ) ;
#25754=EDGE_CURVE ( 'NONE', #25535, #22864, #22562, .T. ) ;
#25759=CARTESIAN_POINT ( 'NONE',  ( 3.756430356250002323, 27.91562499938548569, 11.16877607737301226 ) ) ;
#25765=ADVANCED_FACE ( 'NONE', ( #24505 ), #18017, .F. ) ;
#25767=CARTESIAN_POINT ( 'NONE',  ( 3.999999999999996003, -26.03124999877097068, 6.690598923241487306 ) ) ;
#25768=CARTESIAN_POINT ( 'NONE',  ( -1.878215178124998497, 26.90312499938548285, 12.25316411605951927 ) ) ;
#25770=CYLINDRICAL_SURFACE ( 'NONE', #25019, 4.000000000000000000 ) ;
#25773=CARTESIAN_POINT ( 'NONE',  ( 1.071796769724494336, 25.48615380933863150, 4.999999999999992895 ) ) ;
#25775=VERTEX_POINT ( 'NONE', #11002 ) ;
#25776=DIRECTION ( 'NONE',  ( -0.8660254037844397068, 0.4999999999999983347, -0.000000000000000000 ) ) ;
#25778=CARTESIAN_POINT ( 'NONE',  ( 1.878215178124998497, -28.25312499938548427, 12.25316411605951927 ) ) ;
#25781=ORIENTED_EDGE ( 'NONE', *, *, #16961, .T. ) ;
#25786=CARTESIAN_POINT ( 'NONE',  ( 21.67730602587931088, 19.02110864791986344, 12.25316411605952283 ) ) ;
#25794=CARTESIAN_POINT ( 'NONE',  ( -3.999999999999997335, 27.06250000000000000, 11.30940107675849404 ) ) ;
#25795=( BOUNDED_CURVE ( )  B_SPLINE_CURVE ( 2, ( #18477, #12576, #20286, #14299, #2767, #174, #18599, #2382, #6168 ),
 .UNSPECIFIED., .F., .F. ) 
 B_SPLINE_CURVE_WITH_KNOTS ( ( 3, 2, 2, 2, 3 ),
 ( 0.8249999999999999556, 0.8333333333333333703, 0.8499999999999999778, 0.8666666666666666963, 0.8750000000000000000 ),
 .UNSPECIFIED. ) 
 CURVE ( )  GEOMETRIC_REPRESENTATION_ITEM ( )  RATIONAL_B_SPLINE_CURVE ( ( 0.9330127018922194093, 0.9330127018922189652, 1.000000000000000000, 0.8660254037844387076, 1.000000000000000000, 0.8660254037844387076, 1.000000000000000000, 0.9330127018922194093, 0.9330127018922194093 ) ) 
 REPRESENTATION_ITEM ( '' )  );
#25798=CARTESIAN_POINT ( 'NONE',  ( 17.93165849759071762, 23.24405325350938867, 11.16877607737301048 ) ) ;
#25805=CARTESIAN_POINT ( 'NONE',  ( 3.756430356250004099, 25.74062499938548143, 6.831223922626973533 ) ) ;
#25813=FACE_OUTER_BOUND ( 'NONE', #5649, .T. ) ;
#25816=AXIS2_PLACEMENT_3D ( 'NONE', #3662, #11779, #2099 ) ;
#25820=EDGE_CURVE ( 'NONE', #15394, #1602, #9150, .T. ) ;
#25821=CARTESIAN_POINT ( 'NONE',  ( -1.878215178124995832, 26.19062499938548427, 5.746835883940462963 ) ) ;
#25823=EDGE_CURVE ( 'NONE', #19628, #12515, #18692, .T. ) ;
#25827=CARTESIAN_POINT ( 'NONE',  ( 15.96293558528635081, 21.61978983477866478, 8.999999999999992895 ) ) ;
#25828=CARTESIAN_POINT ( 'NONE',  ( 22.76675617620853131, 17.45436142028971460, 6.831223922626973533 ) ) ;
#25829=CARTESIAN_POINT ( 'NONE',  ( -2.000000000000003997, -28.61874999877096926, 5.535898384862238508 ) ) ;
#25834=FACE_OUTER_BOUND ( 'NONE', #7740, .T. ) ;
#25835=AXIS2_PLACEMENT_3D ( 'NONE', #21816, #7694, #6109 ) ;
#25838=CARTESIAN_POINT ( 'NONE',  ( -2.000000000000003997, -27.32500000000000284, 5.535898384862238508 ) ) ;
#25843=CARTESIAN_POINT ( 'NONE',  ( -11.52193136556785369, 23.36965697125208052, 20.00001200000000168 ) ) ;
#25859=CARTESIAN_POINT ( 'NONE',  ( 20.43330379829292198, 15.12090904237410527, 8.999999999999992895 ) ) ;
#25860=CARTESIAN_POINT ( 'NONE',  ( 15.31328122920215229, 20.97013547869446626, 11.30940107675849404 ) ) ;
#25861=ORIENTED_EDGE ( 'NONE', *, *, #7069, .T. ) ;
#25863=CARTESIAN_POINT ( 'NONE',  ( 1.042539689874651954, 29.98299368898127071, 5.129272290912049392 ) ) ;
#25873=CARTESIAN_POINT ( 'NONE',  ( -1.999999999999995781, 25.99374999877096926, 5.535898384862237620 ) ) ;
#25901=COLOUR_RGB('Sky Blue',0.24,0.69,0.87);
#25902=FILL_AREA_STYLE_COLOUR('',#25901);
#25903=FILL_AREA_STYLE('',(#25902));
#25904=SURFACE_STYLE_FILL_AREA(#25903);
#25905=SURFACE_SIDE_STYLE('',(#25904));
#25906=SURFACE_STYLE_USAGE(.BOTH.,#25905);
#25907=PRESENTATION_STYLE_ASSIGNMENT((#25906));
ENDSEC;
END-ISO-10303-21;
